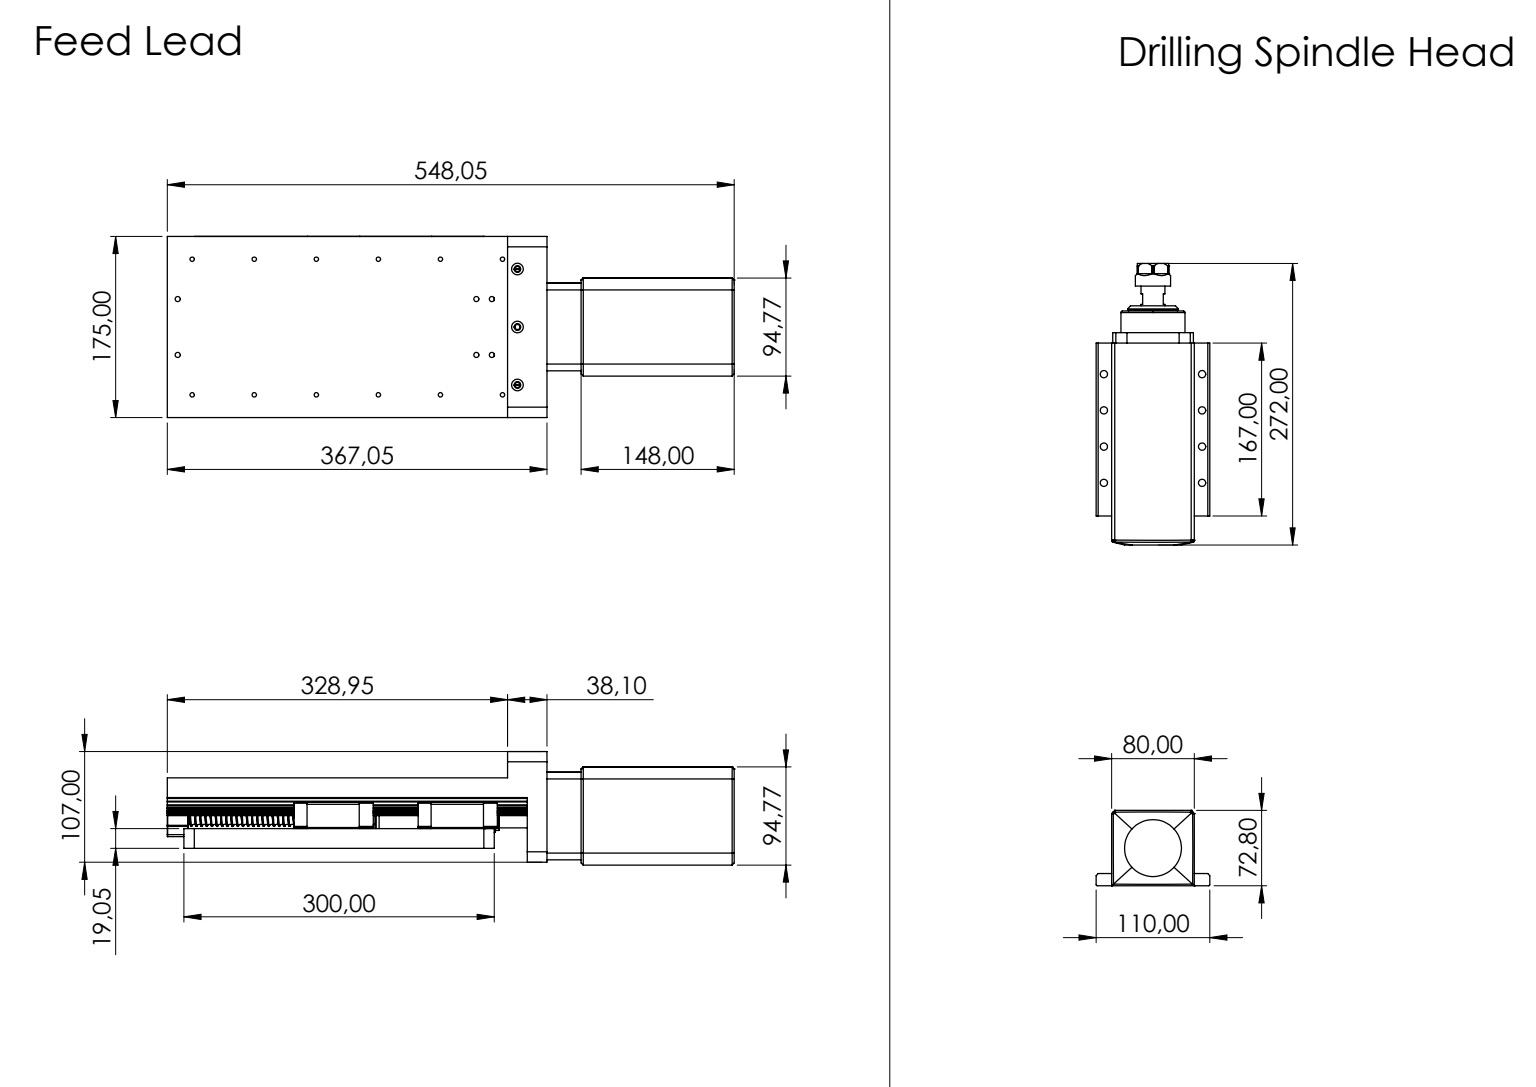
ISO-10303-21;
HEADER;
FILE_DESCRIPTION (('STEP AP214'),
    '1' );
FILE_NAME ('Drilling Spindle Head.step',
    '2026-10-07T11:37:37',
    ( '' ),
    ( '' ),
    'SwSTEP 2.0',
    'SolidWorks 2020',
    '' );
FILE_SCHEMA (( 'AUTOMOTIVE_DESIGN' ));
ENDSEC;

DATA;
#5=LINE ( 'NONE', #3140, #30301 ) ;
#8=EDGE_CURVE ( 'NONE', #34789, #75812, #45689, .T. ) ;
#18=EDGE_CURVE ( 'NONE', #81211, #49424, #24383, .T. ) ;
#40=CARTESIAN_POINT ( 'NONE',  ( 90.06670390244703128, -104.2784471599414644, 0.2178068554180012661 ) ) ;
#41=CIRCLE ( 'NONE', #63855, 11.49999999999999645 ) ;
#57=FACE_OUTER_BOUND ( 'NONE', #13007, .T. ) ;
#62=EDGE_CURVE ( 'NONE', #88900, #78359, #73421, .T. ) ;
#77=CARTESIAN_POINT ( 'NONE',  ( 128.6924155486683503, -121.3595312563307260, 250.2191008560389776 ) ) ;
#86=CARTESIAN_POINT ( 'NONE',  ( 143.0667039024470171, -90.27844715994091018, 230.7030882296565721 ) ) ;
#104=CARTESIAN_POINT ( 'NONE',  ( 107.0667039024470313, -104.2784471599420897, -20.48315503890502143 ) ) ;
#107=CARTESIAN_POINT ( 'NONE',  ( 102.3035641816324102, -89.52844715994213232, -21.78219314458246103 ) ) ;
#108=ORIENTED_EDGE ( 'NONE', *, *, #23655, .T. ) ;
#117=ORIENTED_EDGE ( 'NONE', *, *, #52215, .T. ) ;
#119=EDGE_CURVE ( 'NONE', #83222, #86794, #67726, .T. ) ;
#129=ORIENTED_EDGE ( 'NONE', *, *, #9296, .T. ) ;
#134=EDGE_CURVE ( 'NONE', #34012, #57634, #4396, .T. ) ;
#149=CARTESIAN_POINT ( 'NONE',  ( 70.08426215166053908, -140.6784470016797570, 245.7568090486316805 ) ) ;
#153=ORIENTED_EDGE ( 'NONE', *, *, #81834, .T. ) ;
#161=CARTESIAN_POINT ( 'NONE',  ( 93.91125933621934507, -111.8737466215629013, -21.78219314458179667 ) ) ;
#162=DIRECTION ( 'NONE',  ( 3.100000000000000258E-29, -3.100000000000000044E-14, -1.000000000000000000 ) ) ;
#166=ADVANCED_FACE ( 'NONE', ( #82057 ), #80705, .F. ) ;
#170=CARTESIAN_POINT ( 'NONE',  ( 147.0667039024470739, -140.6784471599409017, 222.2178068554179902 ) ) ;
#211=CARTESIAN_POINT ( 'NONE',  ( 67.65599188636636541, -68.44419502099285069, 246.9104243438740696 ) ) ;
#220=CARTESIAN_POINT ( 'NONE',  ( 107.0667039024470313, -104.2784471599414502, 0.2178068554180012661 ) ) ;
#222=ORIENTED_EDGE ( 'NONE', *, *, #9367, .T. ) ;
#256=VECTOR ( 'NONE', #25789, 1000.000000000000000 ) ;
#281=CARTESIAN_POINT ( 'NONE',  ( 147.0268936274260057, -137.6319380618105015, 245.9633055630636704 ) ) ;
#299=ORIENTED_EDGE ( 'NONE', *, *, #29707, .F. ) ;
#314=DIRECTION ( 'NONE',  ( 1.000000000000000078E-15, -1.000000000000000000, 3.100000000000000044E-14 ) ) ;
#334=DIRECTION ( 'NONE',  ( -1.000000000000000078E-15, 1.000000000000000000, 0.000000000000000000 ) ) ;
#335=ORIENTED_EDGE ( 'NONE', *, *, #11625, .F. ) ;
#377=DIRECTION ( 'NONE',  ( -3.100000000000000258E-29, 3.100000000000000044E-14, 1.000000000000000000 ) ) ;
#379=FACE_OUTER_BOUND ( 'NONE', #43441, .T. ) ;
#381=CYLINDRICAL_SURFACE ( 'NONE', #47045, 27.49999999999999645 ) ;
#390=DIRECTION ( 'NONE',  ( 0.000000000000000000, 0.000000000000000000, -1.000000000000000000 ) ) ;
#399=AXIS2_PLACEMENT_3D ( 'NONE', #39695, #12012, #46047 ) ;
#405=LINE ( 'NONE', #34471, #15075 ) ;
#407=DIRECTION ( 'NONE',  ( -1.000000000000000078E-15, 1.000000000000000000, 0.000000000000000000 ) ) ;
#413=ORIENTED_EDGE ( 'NONE', *, *, #1503, .F. ) ;
#498=CARTESIAN_POINT ( 'NONE',  ( 68.18676274767041434, -81.16192765749869409, 247.4310652601930087 ) ) ;
#503=PLANE ( 'NONE',  #15905 ) ;
#508=DIRECTION ( 'NONE',  ( -1.000000000000000000, -1.734723475976808672E-15, 0.000000000000000000 ) ) ;
#521=ORIENTED_EDGE ( 'NONE', *, *, #75430, .F. ) ;
#525=CARTESIAN_POINT ( 'NONE',  ( 114.6154092934512647, -77.76606036807542921, 250.2178068554179902 ) ) ;
#553=ORIENTED_EDGE ( 'NONE', *, *, #37978, .T. ) ;
#587=CARTESIAN_POINT ( 'NONE',  ( 96.67439905703392355, -92.77844715994214653, -21.78219314458237932 ) ) ;
#588=CARTESIAN_POINT ( 'NONE',  ( 70.69106258991376990, -139.4536831229399070, 247.3802696298695594 ) ) ;
#602=CARTESIAN_POINT ( 'NONE',  ( 68.69590989347372556, -139.3001951612658900, 245.8075977448462197 ) ) ;
#604=DIRECTION ( 'NONE',  ( -0.6757246285173468259, -5.929722281754665310E-16, 0.7371541402007408816 ) ) ;
#612=CARTESIAN_POINT ( 'NONE',  ( 103.2512128930084288, -131.5792096921222480, 250.2178068554180470 ) ) ;
#622=EDGE_CURVE ( 'NONE', #11051, #83707, #61099, .T. ) ;
#624=DIRECTION ( 'NONE',  ( -3.100000000000000258E-29, 3.100000000000000044E-14, 1.000000000000000000 ) ) ;
#625=EDGE_LOOP ( 'NONE', ( #85460, #52936 ) ) ;
#638=VERTEX_POINT ( 'NONE', #15986 ) ;
#645=FACE_OUTER_BOUND ( 'NONE', #52755, .T. ) ;
#646=CIRCLE ( 'NONE', #12254, 3.000000000000002665 ) ;
#650=CARTESIAN_POINT ( 'NONE',  ( 54.06670390244700997, -79.67844715994098692, 222.2178068554179902 ) ) ;
#651=CARTESIAN_POINT ( 'NONE',  ( 67.18382773639109473, -67.99014260483819783, 246.1660416551738990 ) ) ;
#655=ORIENTED_EDGE ( 'NONE', *, *, #13603, .F. ) ;
#661=AXIS2_PLACEMENT_3D ( 'NONE', #79117, #10504, #25470 ) ;
#663=DIRECTION ( 'NONE',  ( -0.8660254037844382635, -0.5000000000000008882, 1.550000000000000022E-14 ) ) ;
#672=DIRECTION ( 'NONE',  ( 3.100000000000000258E-29, -3.100000000000000044E-14, -1.000000000000000000 ) ) ;
#694=DIRECTION ( 'NONE',  ( -0.8660254037844392627, 0.4999999999999990008, -1.549999999999999706E-14 ) ) ;
#696=FACE_OUTER_BOUND ( 'NONE', #29082, .T. ) ;
#701=VERTEX_POINT ( 'NONE', #9167 ) ;
#714=PLANE ( 'NONE',  #87235 ) ;
#716=ORIENTED_EDGE ( 'NONE', *, *, #77579, .T. ) ;
#719=CARTESIAN_POINT ( 'NONE',  ( 107.5667039024470455, -113.7784471599413791, 2.217806855418308132 ) ) ;
#720=CARTESIAN_POINT ( 'NONE',  ( 146.8610933598213251, -137.5366814833658395, 246.4167843500817412 ) ) ;
#734=CARTESIAN_POINT ( 'NONE',  ( 107.0667039024470313, -104.2784471599418197, -11.78219314458200984 ) ) ;
#753=VERTEX_POINT ( 'NONE', #23701 ) ;
#786=ORIENTED_EDGE ( 'NONE', *, *, #30299, .T. ) ;
#793=AXIS2_PLACEMENT_3D ( 'NONE', #52763, #58282, #86014 ) ;
#811=AXIS2_PLACEMENT_3D ( 'NONE', #82943, #28399, #22065 ) ;
#817=DIRECTION ( 'NONE',  ( -3.100000000000000258E-29, 3.100000000000000044E-14, 1.000000000000000000 ) ) ;
#830=CYLINDRICAL_SURFACE ( 'NONE', #17828, 3.500000000000003109 ) ;
#835=DIRECTION ( 'NONE',  ( -1.000000000000000000, -1.734723475976808672E-15, 0.000000000000000000 ) ) ;
#887=EDGE_CURVE ( 'NONE', #701, #2874, #49105, .T. ) ;
#916=LINE ( 'NONE', #34531, #21635 ) ;
#921=FACE_BOUND ( 'NONE', #56521, .T. ) ;
#922=EDGE_CURVE ( 'NONE', #4290, #47689, #37387, .T. ) ;
#930=CIRCLE ( 'NONE', #79267, 30.99999999999998579 ) ;
#936=VECTOR ( 'NONE', #85029, 1000.000000000000000 ) ;
#942=ORIENTED_EDGE ( 'NONE', *, *, #84667, .T. ) ;
#958=DIRECTION ( 'NONE',  ( -1.000000000000000078E-15, 1.000000000000000000, 0.000000000000000000 ) ) ;
#960=VERTEX_POINT ( 'NONE', #11251 ) ;
#967=CARTESIAN_POINT ( 'NONE',  ( 99.06670390244704549, -104.2784471599421323, -21.78219314458201694 ) ) ;
#975=CARTESIAN_POINT ( 'NONE',  ( 90.06670420047028358, -137.6784471599409585, 222.2178068554179902 ) ) ;
#981=CARTESIAN_POINT ( 'NONE',  ( 103.2512128930081730, -76.97768462775967180, 250.2178068554180470 ) ) ;
#984=CARTESIAN_POINT ( 'NONE',  ( 68.76253601752615907, -136.8623718444874555, 247.4903208786739981 ) ) ;
#998=CARTESIAN_POINT ( 'NONE',  ( 158.0667039024469886, -67.87844715994090450, 120.2178068554179902 ) ) ;
#1013=DIRECTION ( 'NONE',  ( -3.100000000000000258E-29, 3.100000000000000044E-14, 1.000000000000000000 ) ) ;
#1027=DIRECTION ( 'NONE',  ( 0.000000000000000000, 0.000000000000000000, -1.000000000000000000 ) ) ;
#1060=CARTESIAN_POINT ( 'NONE',  ( 68.70366513962476063, -139.2930699478345389, 245.9105554508155649 ) ) ;
#1067=AXIS2_PLACEMENT_3D ( 'NONE', #89420, #55748, #68523 ) ;
#1076=DIRECTION ( 'NONE',  ( 0.000000000000000000, 0.000000000000000000, 1.000000000000000000 ) ) ;
#1093=DIRECTION ( 'NONE',  ( 1.000000000000000000, 1.132880637372608296E-15, 0.000000000000000000 ) ) ;
#1108=CARTESIAN_POINT ( 'NONE',  ( 107.0667039024470313, -104.2784471599413934, 2.217806855418003043 ) ) ;
#1119=AXIS2_PLACEMENT_3D ( 'NONE', #62798, #47484, #18902 ) ;
#1121=LINE ( 'NONE', #34282, #64196 ) ;
#1125=VECTOR ( 'NONE', #24217, 1000.000000000000000 ) ;
#1141=AXIS2_PLACEMENT_3D ( 'NONE', #65937, #38679, #53176 ) ;
#1172=CARTESIAN_POINT ( 'NONE',  ( 107.0667039024470313, -104.2784471599420471, -19.18411693322902423 ) ) ;
#1177=DIRECTION ( 'NONE',  ( -3.100000000000000258E-29, 3.100000000000000044E-14, 1.000000000000000000 ) ) ;
#1179=CARTESIAN_POINT ( 'NONE',  ( 151.0667039024469886, -79.67844715994088745, 190.2178068554179902 ) ) ;
#1185=ORIENTED_EDGE ( 'NONE', *, *, #8505, .T. ) ;
#1215=VECTOR ( 'NONE', #17266, 1000.000000000000000 ) ;
#1217=ORIENTED_EDGE ( 'NONE', *, *, #20900, .F. ) ;
#1226=CARTESIAN_POINT ( 'NONE',  ( 74.06670390244701707, -90.27844715994098124, 45.21780685541799727 ) ) ;
#1252=VECTOR ( 'NONE', #76868, 1000.000000000000000 ) ;
#1284=EDGE_LOOP ( 'NONE', ( #79248, #45274, #6602, #1217 ) ) ;
#1286=DIRECTION ( 'NONE',  ( 0.8660254037844345998, 0.5000000000000069944, -1.550000000000018954E-14 ) ) ;
#1289=ORIENTED_EDGE ( 'NONE', *, *, #60837, .T. ) ;
#1303=EDGE_LOOP ( 'NONE', ( #77384, #63806 ) ) ;
#1304=VERTEX_POINT ( 'NONE', #47095 ) ;
#1309=DIRECTION ( 'NONE',  ( 0.7759704746411385523, -0.6307692307692301936, 0.000000000000000000 ) ) ;
#1336=ORIENTED_EDGE ( 'NONE', *, *, #44690, .T. ) ;
#1337=VERTEX_POINT ( 'NONE', #84803 ) ;
#1348=ORIENTED_EDGE ( 'NONE', *, *, #46560, .F. ) ;
#1361=ORIENTED_EDGE ( 'NONE', *, *, #7930, .F. ) ;
#1369=ORIENTED_EDGE ( 'NONE', *, *, #61406, .F. ) ;
#1409=CARTESIAN_POINT ( 'NONE',  ( 67.06670390244705970, -127.7048595798752899, 245.5588919304049682 ) ) ;
#1424=CARTESIAN_POINT ( 'NONE',  ( 144.0667052733537901, -83.77844715994089597, 55.21780685541800437 ) ) ;
#1431=CYLINDRICAL_SURFACE ( 'NONE', #27367, 3.000000000000002665 ) ;
#1435=VECTOR ( 'NONE', #88705, 1000.000000000000227 ) ;
#1500=CARTESIAN_POINT ( 'NONE',  ( 99.48898161933324502, -91.15344715994181968, -11.78219314458242550 ) ) ;
#1503=EDGE_CURVE ( 'NONE', #25396, #23110, #20428, .T. ) ;
#1504=ORIENTED_EDGE ( 'NONE', *, *, #70487, .F. ) ;
#1506=DIRECTION ( 'NONE',  ( -3.100000000000000258E-29, 3.100000000000000044E-14, 1.000000000000000000 ) ) ;
#1507=CARTESIAN_POINT ( 'NONE',  ( 70.74156425739846554, -139.3372952672478675, 247.4251605867160890 ) ) ;
#1539=VERTEX_POINT ( 'NONE', #34271 ) ;
#1546=AXIS2_PLACEMENT_3D ( 'NONE', #84659, #29240, #27879 ) ;
#1567=CARTESIAN_POINT ( 'NONE',  ( 67.64413875234457407, -68.43291640910719309, 246.8985623378813159 ) ) ;
#1569=ORIENTED_EDGE ( 'NONE', *, *, #59201, .F. ) ;
#1573=ADVANCED_FACE ( 'NONE', ( #75171, #55136 ), #5237, .T. ) ;
#1585=ORIENTED_EDGE ( 'NONE', *, *, #13032, .F. ) ;
#1602=ORIENTED_EDGE ( 'NONE', *, *, #5397, .T. ) ;
#1605=EDGE_CURVE ( 'NONE', #72685, #51113, #82002, .T. ) ;
#1616=AXIS2_PLACEMENT_3D ( 'NONE', #45612, #38825, #79744 ) ;
#1627=VERTEX_POINT ( 'NONE', #6140 ) ;
#1673=DIRECTION ( 'NONE',  ( -1.000000000000000000, -1.541976423090496028E-15, 0.000000000000000000 ) ) ;
#1678=DIRECTION ( 'NONE',  ( 0.5000000000000015543, 0.8660254037844377084, -2.688821387764056676E-14 ) ) ;
#1679=PLANE ( 'NONE',  #16706 ) ;
#1684=VECTOR ( 'NONE', #64083, 1000.000000000000000 ) ;
#1698=CARTESIAN_POINT ( 'NONE',  ( 107.9678037105606450, -121.2545485715094316, -21.78219314458149114 ) ) ;
#1708=ORIENTED_EDGE ( 'NONE', *, *, #73968, .F. ) ;
#1714=EDGE_CURVE ( 'NONE', #61133, #37103, #77865, .T. ) ;
#1722=CARTESIAN_POINT ( 'NONE',  ( 66.95718368952854860, -124.7784471599409954, 55.21780685541800437 ) ) ;
#1723=ORIENTED_EDGE ( 'NONE', *, *, #20357, .T. ) ;
#1738=DIRECTION ( 'NONE',  ( 1.000000000000000078E-15, -1.000000000000000000, 0.000000000000000000 ) ) ;
#1741=CARTESIAN_POINT ( 'NONE',  ( 110.0667047667142953, -67.87844715994094713, 115.9678068554179902 ) ) ;
#1742=VERTEX_POINT ( 'NONE', #13838 ) ;
#1745=VERTEX_POINT ( 'NONE', #41521 ) ;
#1758=LINE ( 'NONE', #63982, #48154 ) ;
#1769=CIRCLE ( 'NONE', #75679, 2.999999999999988898 ) ;
#1783=CARTESIAN_POINT ( 'NONE',  ( 74.19170390244700286, -80.65344715994098124, 45.21780685541799727 ) ) ;
#1809=CARTESIAN_POINT ( 'NONE',  ( 68.91673588226457525, -69.56165432392101877, 247.5002287295815790 ) ) ;
#1820=B_SPLINE_CURVE_WITH_KNOTS ( 'NONE', 3,
 ( #34572, #20518, #75917, #13685, #69105 ),
 .UNSPECIFIED., .F., .F.,
 ( 4, 1, 4 ),
 ( 0.000000000000000000, 0.4316414630428307975, 1.000000000000000000 ),
 .UNSPECIFIED. ) ;
#1835=AXIS2_PLACEMENT_3D ( 'NONE', #87398, #74220, #60113 ) ;
#1851=EDGE_CURVE ( 'NONE', #85229, #66416, #26062, .T. ) ;
#1857=CARTESIAN_POINT ( 'NONE',  ( 67.36714851195648635, -67.87168324244640871, 246.8533852577239998 ) ) ;
#1864=VERTEX_POINT ( 'NONE', #16088 ) ;
#1907=EDGE_CURVE ( 'NONE', #41462, #11071, #64672, .T. ) ;
#1923=FACE_OUTER_BOUND ( 'NONE', #29612, .T. ) ;
#1929=LINE ( 'NONE', #56417, #15979 ) ;
#1934=VECTOR ( 'NONE', #63013, 1000.000000000000000 ) ;
#1951=CARTESIAN_POINT ( 'NONE',  ( 70.50919912965197511, -139.8621867207610308, 247.1491889055018305 ) ) ;
#1990=DIRECTION ( 'NONE',  ( -1.000000000000000000, -1.000000000000000078E-15, 5.773159642023980606E-15 ) ) ;
#1991=FACE_OUTER_BOUND ( 'NONE', #56263, .T. ) ;
#1992=CARTESIAN_POINT ( 'NONE',  ( 146.5099599153435008, -138.2352025272441836, 245.9283337036430055 ) ) ;
#2001=DIRECTION ( 'NONE',  ( -1.000000000000000000, 0.000000000000000000, 0.000000000000000000 ) ) ;
#2010=ORIENTED_EDGE ( 'NONE', *, *, #76441, .F. ) ;
#2011=ORIENTED_EDGE ( 'NONE', *, *, #41800, .F. ) ;
#2013=EDGE_CURVE ( 'NONE', #61542, #42555, #33274, .T. ) ;
#2016=CARTESIAN_POINT ( 'NONE',  ( 145.3595637443018234, -69.45303146431501773, 247.4784022495120155 ) ) ;
#2030=DIRECTION ( 'NONE',  ( 1.000000000000000000, 1.000000000000000078E-15, 0.000000000000000000 ) ) ;
#2032=ORIENTED_EDGE ( 'NONE', *, *, #52612, .F. ) ;
#2057=CARTESIAN_POINT ( 'NONE',  ( 68.09411347895392908, -99.27098689615887395, 247.4783998280180128 ) ) ;
#2058=ORIENTED_EDGE ( 'NONE', *, *, #78733, .F. ) ;
#2060=ORIENTED_EDGE ( 'NONE', *, *, #17855, .F. ) ;
#2106=EDGE_CURVE ( 'NONE', #64360, #47447, #53685, .T. ) ;
#2107=VERTEX_POINT ( 'NONE', #61415 ) ;
#2119=LINE ( 'NONE', #17528, #69835 ) ;
#2121=AXIS2_PLACEMENT_3D ( 'NONE', #62039, #89773, #41583 ) ;
#2122=LINE ( 'NONE', #71173, #32626 ) ;
#2160=ORIENTED_EDGE ( 'NONE', *, *, #19869, .F. ) ;
#2164=CARTESIAN_POINT ( 'NONE',  ( 151.0667039024469886, -67.87844715994090450, 190.2178068554179902 ) ) ;
#2168=LINE ( 'NONE', #56199, #62006 ) ;
#2185=CIRCLE ( 'NONE', #13772, 3.999999999999992895 ) ;
#2203=ORIENTED_EDGE ( 'NONE', *, *, #46360, .F. ) ;
#2205=LINE ( 'NONE', #8118, #27880 ) ;
#2209=CARTESIAN_POINT ( 'NONE',  ( 110.2536356736639078, -101.8611209747513868, -19.78219314458209865 ) ) ;
#2215=VECTOR ( 'NONE', #80038, 1000.000000000000000 ) ;
#2218=VECTOR ( 'NONE', #39800, 1000.000000000000000 ) ;
#2222=DIRECTION ( 'NONE',  ( 0.000000000000000000, 0.000000000000000000, 1.000000000000000000 ) ) ;
#2224=EDGE_CURVE ( 'NONE', #51923, #24886, #89215, .T. ) ;
#2254=DIRECTION ( 'NONE',  ( -1.000000000000000000, -1.000000000000000078E-15, 0.000000000000000000 ) ) ;
#2263=CIRCLE ( 'NONE', #22569, 7.999999999999992895 ) ;
#2264=ORIENTED_EDGE ( 'NONE', *, *, #48437, .T. ) ;
#2267=DIRECTION ( 'NONE',  ( 3.100000000000000258E-29, -3.100000000000000044E-14, -1.000000000000000000 ) ) ;
#2270=CARTESIAN_POINT ( 'NONE',  ( 143.6785940946288633, -138.5762527540428835, 247.5817532094160072 ) ) ;
#2273=DIRECTION ( 'NONE',  ( -1.000000000000000078E-15, 1.000000000000000000, 0.000000000000000000 ) ) ;
#2274=ORIENTED_EDGE ( 'NONE', *, *, #31325, .T. ) ;
#2298=B_SPLINE_CURVE_WITH_KNOTS ( 'NONE', 3,
 ( #3064, #28982, #86185, #14912 ),
 .UNSPECIFIED., .F., .F.,
 ( 4, 4 ),
 ( -0.3974825557268150122, -0.3842043193313849914 ),
 .UNSPECIFIED. ) ;
#2302=ORIENTED_EDGE ( 'NONE', *, *, #57521, .T. ) ;
#2303=DIRECTION ( 'NONE',  ( -0.4999999999999989453, -0.8660254037844392627, 2.684678751731760294E-14 ) ) ;
#2324=AXIS2_PLACEMENT_3D ( 'NONE', #19974, #41733, #69919 ) ;
#2337=CARTESIAN_POINT ( 'NONE',  ( 147.0667039024469886, -67.87844715994090450, 222.2178068554179902 ) ) ;
#2348=CARTESIAN_POINT ( 'NONE',  ( 115.0988951105837117, -100.2184096729307328, 2.217806855417864043 ) ) ;
#2390=B_SPLINE_CURVE_WITH_KNOTS ( 'NONE', 3,
 ( #7423, #48730, #29221, #63284, #69654, #35115, #62824, #602, #15597, #21515, #1060, #56908, #49185, #76919, #50085, #77819, #28770, #38692, #65952, #44608, #2409, #23754, #23321, #16931, #36922, #64624, #51861, #72344, #10111, #66397, #17814, #71461, #50987, #43722, #17371, #51422, #9224, #38255, #78728, #16485, #79171, #4187, #37820, #65074, #58684 ),
 .UNSPECIFIED., .F., .F.,
 ( 4, 2, 2, 2, 1, 1, 2, 2, 2, 1, 1, 2, 2, 2, 2, 1, 1, 1, 2, 2, 2, 2, 1, 1, 2, 2, 4 ),
 ( 0.000000000000000000, 0.03125000000003638062, 0.04687500000005471318, 0.06250000000007303880, 0.09375000000011092516, 0.1093750000001298545, 0.1171875000001566386, 0.1250000000001834088, 0.1875000000003400336, 0.2187500000004195255, 0.2343750000004746481, 0.2421875000004988232, 0.2500000000005230261, 0.3750000000008891776, 0.4375000000010721979, 0.4687500000011416423, 0.4843750000011794454, 0.4921875000012016499, 0.4960937500012127521, 0.5000000000012239099, 0.6250000000010771384, 0.6875000000010104140, 0.7187500000009768852, 0.7343750000009601209, 0.7421875000009404699, 0.7500000000009208190, 1.000000000000000000 ),
 .UNSPECIFIED. ) ;
#2394=DIRECTION ( 'NONE',  ( 0.000000000000000000, 0.000000000000000000, 1.000000000000000000 ) ) ;
#2399=DIRECTION ( 'NONE',  ( 0.8660254037844382635, 0.5000000000000008882, -1.550000000000000022E-14 ) ) ;
#2402=ORIENTED_EDGE ( 'NONE', *, *, #19038, .F. ) ;
#2409=CARTESIAN_POINT ( 'NONE',  ( 68.75201276470878042, -139.2464705024164857, 246.2314480513125261 ) ) ;
#2466=CARTESIAN_POINT ( 'NONE',  ( 145.2750608293226833, -69.56425712815943996, 247.5000682988239760 ) ) ;
#2467=CARTESIAN_POINT ( 'NONE',  ( 146.2016781114348305, -68.71199849507584645, 247.1480963241265272 ) ) ;
#2481=ORIENTED_EDGE ( 'NONE', *, *, #35705, .F. ) ;
#2532=ORIENTED_EDGE ( 'NONE', *, *, #31514, .F. ) ;
#2534=DIRECTION ( 'NONE',  ( -3.100000000000000258E-29, 3.100000000000000044E-14, 1.000000000000000000 ) ) ;
#2559=VECTOR ( 'NONE', #87502, 1000.000000000000000 ) ;
#2572=CARTESIAN_POINT ( 'NONE',  ( 67.06681736700808472, -67.87844715931913697, 245.5130139978070076 ) ) ;
#2577=VECTOR ( 'NONE', #78490, 1000.000000000000000 ) ;
#2587=ORIENTED_EDGE ( 'NONE', *, *, #83860, .T. ) ;
#2593=LINE ( 'NONE', #1698, #76570 ) ;
#2630=LINE ( 'NONE', #24848, #17598 ) ;
#2634=AXIS2_PLACEMENT_3D ( 'NONE', #66343, #30502, #71407 ) ;
#2636=DIRECTION ( 'NONE',  ( 0.000000000000000000, 0.000000000000000000, -1.000000000000000000 ) ) ;
#2648=VECTOR ( 'NONE', #89767, 1000.000000000000000 ) ;
#2668=AXIS2_PLACEMENT_3D ( 'NONE', #71158, #37954, #77965 ) ;
#2669=ORIENTED_EDGE ( 'NONE', *, *, #58690, .F. ) ;
#2677=CARTESIAN_POINT ( 'NONE',  ( 107.0667039024470313, -104.2784471599418197, -11.78219314458200984 ) ) ;
#2691=ORIENTED_EDGE ( 'NONE', *, *, #72281, .T. ) ;
#2702=CARTESIAN_POINT ( 'NONE',  ( 68.90393785523644965, -69.55022374562288690, 247.4982723397321251 ) ) ;
#2707=DIRECTION ( 'NONE',  ( -0.000000000000000000, -0.000000000000000000, -1.000000000000000000 ) ) ;
#2737=CARTESIAN_POINT ( 'NONE',  ( 56.06670390244699576, -67.87844715994098976, 190.2178068554179902 ) ) ;
#2745=DIRECTION ( 'NONE',  ( 1.000000000000000078E-15, -1.000000000000000000, 0.000000000000000000 ) ) ;
#2749=CARTESIAN_POINT ( 'NONE',  ( 107.0667039024469886, -67.87844715994094713, 93.21780685541800437 ) ) ;
#2772=CARTESIAN_POINT ( 'NONE',  ( 67.06670390244707392, -137.6766936484476958, 245.4930518797220032 ) ) ;
#2777=VECTOR ( 'NONE', #34885, 999.9999999999998863 ) ;
#2833=VERTEX_POINT ( 'NONE', #28364 ) ;
#2834=CYLINDRICAL_SURFACE ( 'NONE', #80225, 3.499999999999996003 ) ;
#2858=CARTESIAN_POINT ( 'NONE',  ( 67.06670390244700286, -67.87844715994098976, 222.2178068554179902 ) ) ;
#2874=VERTEX_POINT ( 'NONE', #58738 ) ;
#2875=CARTESIAN_POINT ( 'NONE',  ( 107.0667039024470313, -104.2784471599420897, -20.48315503890502143 ) ) ;
#2885=CARTESIAN_POINT ( 'NONE',  ( 77.06670390244701707, -90.27844715994098124, 230.7030882296565721 ) ) ;
#2909=CARTESIAN_POINT ( 'NONE',  ( 90.57859886853759690, -68.78570139166994579, 247.5000682988239760 ) ) ;
#2910=CARTESIAN_POINT ( 'NONE',  ( 146.9135422721272448, -68.02287184880887594, 246.2552768418564710 ) ) ;
#2921=ORIENTED_EDGE ( 'NONE', *, *, #10620, .F. ) ;
#2927=VECTOR ( 'NONE', #1076, 1000.000000000000000 ) ;
#2929=ORIENTED_EDGE ( 'NONE', *, *, #70817, .T. ) ;
#2951=VECTOR ( 'NONE', #72879, 1000.000000000000000 ) ;
#3003=CARTESIAN_POINT ( 'NONE',  ( 129.9417039024469886, -68.87844715994091871, 138.7178068554180186 ) ) ;
#3021=ORIENTED_EDGE ( 'NONE', *, *, #29193, .T. ) ;
#3022=ORIENTED_EDGE ( 'NONE', *, *, #18736, .F. ) ;
#3023=EDGE_CURVE ( 'NONE', #28371, #5243, #34541, .T. ) ;
#3032=AXIS2_PLACEMENT_3D ( 'NONE', #32379, #68272, #87814 ) ;
#3053=VERTEX_POINT ( 'NONE', #87807 ) ;
#3059=ORIENTED_EDGE ( 'NONE', *, *, #48221, .T. ) ;
#3060=VECTOR ( 'NONE', #65842, 999.9999999999998863 ) ;
#3064=CARTESIAN_POINT ( 'NONE',  ( 107.9678037105606023, -87.30234574837474781, -19.18411693322955003 ) ) ;
#3075=CARTESIAN_POINT ( 'NONE',  ( 143.0667039024470171, -118.2784471599408960, 230.7030882296565721 ) ) ;
#3077=CARTESIAN_POINT ( 'NONE',  ( 82.96822048844396136, -129.2743616038035555, 249.3173333679100097 ) ) ;
#3082=ORIENTED_EDGE ( 'NONE', *, *, #36963, .F. ) ;
#3089=FACE_OUTER_BOUND ( 'NONE', #23564, .T. ) ;
#3126=CIRCLE ( 'NONE', #14750, 1.500000000000001332 ) ;
#3136=CIRCLE ( 'NONE', #7483, 4.500000000000003553 ) ;
#3140=CARTESIAN_POINT ( 'NONE',  ( 67.06670390244707392, -137.6784471599409869, 228.4678068554179902 ) ) ;
#3142=CARTESIAN_POINT ( 'NONE',  ( 92.91125933621934507, -113.6057974291316981, -19.26696060647573105 ) ) ;
#3143=CYLINDRICAL_SURFACE ( 'NONE', #12103, 24.50000000000000711 ) ;
#3171=AXIS2_PLACEMENT_3D ( 'NONE', #33661, #51948, #31080 ) ;
#3193=ORIENTED_EDGE ( 'NONE', *, *, #4873, .T. ) ;
#3194=CARTESIAN_POINT ( 'NONE',  ( 110.2536356736639220, -106.6957733451320394, 2.217806855418086087 ) ) ;
#3197=CIRCLE ( 'NONE', #10449, 3.500000000000003109 ) ;
#3263=ORIENTED_EDGE ( 'NONE', *, *, #64249, .T. ) ;
#3266=DIRECTION ( 'NONE',  ( 1.000000000000000078E-15, -1.000000000000000000, 3.100000000000000044E-14 ) ) ;
#3289=ORIENTED_EDGE ( 'NONE', *, *, #36504, .T. ) ;
#3332=FACE_OUTER_BOUND ( 'NONE', #52166, .T. ) ;
#3347=AXIS2_PLACEMENT_3D ( 'NONE', #55568, #56024, #63315 ) ;
#3356=CARTESIAN_POINT ( 'NONE',  ( 86.71899144006731319, -85.80981821983746727, 250.2201230397200220 ) ) ;
#3358=DIRECTION ( 'NONE',  ( -1.000000000000000000, 0.000000000000000000, 0.000000000000000000 ) ) ;
#3367=ADVANCED_FACE ( 'NONE', ( #24580 ), #52247, .F. ) ;
#3370=DIRECTION ( 'NONE',  ( 3.100000000000000258E-29, -3.100000000000000044E-14, -1.000000000000000000 ) ) ;
#3381=VERTEX_POINT ( 'NONE', #80009 ) ;
#3391=ORIENTED_EDGE ( 'NONE', *, *, #2013, .T. ) ;
#3399=CARTESIAN_POINT ( 'NONE',  ( 123.1292039024470029, -68.87844715994093292, 222.2178068554179902 ) ) ;
#3408=ADVANCED_BREP_SHAPE_REPRESENTATION ( '', ( #20639, #50656 ), #4304 ) ;
#3411=CARTESIAN_POINT ( 'NONE',  ( 67.49635100332064042, -137.4243301806155841, 246.7471779864713994 ) ) ;
#3412=DIRECTION ( 'NONE',  ( -3.100000000000000258E-29, 3.100000000000000044E-14, 1.000000000000000000 ) ) ;
#3439=ORIENTED_EDGE ( 'NONE', *, *, #23571, .T. ) ;
#3443=CARTESIAN_POINT ( 'NONE',  ( 147.0667039024470739, -137.6784471599409017, 228.4678068554179902 ) ) ;
#3464=EDGE_LOOP ( 'NONE', ( #42569, #33408, #27715, #60217, #68798, #53637, #1185, #81075, #30294, #70743, #67951, #15665, #4398, #59481, #21360, #55428, #73289, #84793, #23699, #19501, #86373, #70073 ) ) ;
#3465=EDGE_LOOP ( 'NONE', ( #22122, #15213, #52644, #21783 ) ) ;
#3476=DIRECTION ( 'NONE',  ( -1.000000000000000078E-15, 1.000000000000000000, 0.000000000000000000 ) ) ;
#3479=ORIENTED_EDGE ( 'NONE', *, *, #7458, .T. ) ;
#3524=VECTOR ( 'NONE', #83759, 1000.000000000000000 ) ;
#3528=ORIENTED_EDGE ( 'NONE', *, *, #29932, .T. ) ;
#3539=DIRECTION ( 'NONE',  ( -1.000000000000000000, -1.541976423090496028E-15, 0.000000000000000000 ) ) ;
#3543=ORIENTED_EDGE ( 'NONE', *, *, #20270, .F. ) ;
#3551=EDGE_CURVE ( 'NONE', #88193, #23818, #74962, .T. ) ;
#3578=CARTESIAN_POINT ( 'NONE',  ( 112.7812478461076040, -67.87844715994094713, 245.8358747327640117 ) ) ;
#3596=LINE ( 'NONE', #65219, #86816 ) ;
#3628=DIRECTION ( 'NONE',  ( 1.000000000000000078E-15, -1.000000000000000000, 0.000000000000000000 ) ) ;
#3634=FACE_BOUND ( 'NONE', #68129, .T. ) ;
#3641=DIRECTION ( 'NONE',  ( -1.000000000000000078E-15, 1.000000000000000000, 0.000000000000000000 ) ) ;
#3710=VECTOR ( 'NONE', #80088, 1000.000000000000000 ) ;
#3730=AXIS2_PLACEMENT_3D ( 'NONE', #30373, #9044, #2222 ) ;
#3747=PLANE ( 'NONE',  #31791 ) ;
#3757=VECTOR ( 'NONE', #82035, 1000.000000000000000 ) ;
#3786=CARTESIAN_POINT ( 'NONE',  ( 98.58946256649487339, -99.96145986183429955, -19.78219314458215550 ) ) ;
#3792=ORIENTED_EDGE ( 'NONE', *, *, #60951, .F. ) ;
#3794=CARTESIAN_POINT ( 'NONE',  ( 130.8259623650636172, -69.00418878328892447, 247.5000682988239760 ) ) ;
#3800=DIRECTION ( 'NONE',  ( 3.100000000000000258E-29, -3.100000000000000044E-14, -1.000000000000000000 ) ) ;
#3829=CARTESIAN_POINT ( 'NONE',  ( 107.0667039024470313, -104.2784471599408676, 19.21780685541799016 ) ) ;
#3832=ORIENTED_EDGE ( 'NONE', *, *, #72216, .F. ) ;
#3834=AXIS2_PLACEMENT_3D ( 'NONE', #63675, #55033, #13732 ) ;
#3842=AXIS2_PLACEMENT_3D ( 'NONE', #36859, #57745, #72282 ) ;
#3843=CARTESIAN_POINT ( 'NONE',  ( 107.0667039024470313, -104.2784471599414502, 0.2178068554180012661 ) ) ;
#3844=CARTESIAN_POINT ( 'NONE',  ( 143.2522959336310748, -139.0102598546870922, 247.5112310255240118 ) ) ;
#3850=EDGE_CURVE ( 'NONE', #44698, #89450, #63272, .T. ) ;
#3854=CARTESIAN_POINT ( 'NONE',  ( 67.10629922391730418, -137.6313948336576232, 245.9678581484365907 ) ) ;
#3858=ORIENTED_EDGE ( 'NONE', *, *, #2106, .T. ) ;
#3879=DIRECTION ( 'NONE',  ( 3.100000000000000258E-29, -3.100000000000000044E-14, -1.000000000000000000 ) ) ;
#3901=CARTESIAN_POINT ( 'NONE',  ( 82.02983075842482208, -92.77767617834393832, 250.2178068554179902 ) ) ;
#3905=CIRCLE ( 'NONE', #50324, 173.3227045127110273 ) ;
#3909=ORIENTED_EDGE ( 'NONE', *, *, #10072, .T. ) ;
#3917=AXIS2_PLACEMENT_3D ( 'NONE', #27024, #56950, #14751 ) ;
#3918=AXIS2_PLACEMENT_3D ( 'NONE', #54513, #5968, #40012 ) ;
#3930=CARTESIAN_POINT ( 'NONE',  ( 110.2536356736639078, -101.8611209747513868, -19.78219314458209865 ) ) ;
#3952=CARTESIAN_POINT ( 'NONE',  ( 97.06670390244703128, -109.9573555057411340, 17.71780685541815714 ) ) ;
#3955=ORIENTED_EDGE ( 'NONE', *, *, #34121, .F. ) ;
#3956=FACE_OUTER_BOUND ( 'NONE', #75464, .T. ) ;
#3960=CARTESIAN_POINT ( 'NONE',  ( 103.8797721312301547, -106.6957733451327215, -19.78219314458193168 ) ) ;
#3965=CARTESIAN_POINT ( 'NONE',  ( 107.0667039024470313, -104.2784471599413934, 2.217806855418003043 ) ) ;
#3973=VERTEX_POINT ( 'NONE', #44001 ) ;
#3975=VECTOR ( 'NONE', #27151, 1000.000000000000000 ) ;
#3980=ORIENTED_EDGE ( 'NONE', *, *, #65488, .F. ) ;
#3981=DIRECTION ( 'NONE',  ( 0.000000000000000000, 0.000000000000000000, -1.000000000000000000 ) ) ;
#3983=FACE_OUTER_BOUND ( 'NONE', #80737, .T. ) ;
#3984=EDGE_CURVE ( 'NONE', #79449, #88193, #70403, .T. ) ;
#3986=CARTESIAN_POINT ( 'NONE',  ( 122.2189888861420286, -111.9861225405540353, -19.18411693322877198 ) ) ;
#4008=ADVANCED_FACE ( 'NONE', ( #24920 ), #47573, .T. ) ;
#4023=FACE_OUTER_BOUND ( 'NONE', #50223, .T. ) ;
#4049=ORIENTED_EDGE ( 'NONE', *, *, #30302, .T. ) ;
#4051=CARTESIAN_POINT ( 'NONE',  ( 125.5177273812784762, -131.0330679306342461, 55.21780685541800437 ) ) ;
#4069=ORIENTED_EDGE ( 'NONE', *, *, #17170, .T. ) ;
#4081=CARTESIAN_POINT ( 'NONE',  ( 91.91229715706504066, -111.9484203394872850, -19.21044887263775891 ) ) ;
#4089=PLANE ( 'NONE',  #64691 ) ;
#4092=CARTESIAN_POINT ( 'NONE',  ( 67.06673837846007302, -137.6758525980020806, 245.5072637273240161 ) ) ;
#4094=CIRCLE ( 'NONE', #86776, 7.999999999999992895 ) ;
#4100=VERTEX_POINT ( 'NONE', #67139 ) ;
#4108=DIRECTION ( 'NONE',  ( 1.000000000000000000, 1.000000000000013883E-15, 4.440892098500630106E-16 ) ) ;
#4111=VERTEX_POINT ( 'NONE', #81691 ) ;
#4122=DIRECTION ( 'NONE',  ( 0.4999999999999994449, 0.8660254037844390407, -2.684678751731759347E-14 ) ) ;
#4130=CARTESIAN_POINT ( 'NONE',  ( 122.2221484686745185, -96.57698625956679450, -11.78219314458225853 ) ) ;
#4132=VECTOR ( 'NONE', #47429, 1000.000000000000000 ) ;
#4137=ADVANCED_FACE ( 'NONE', ( #38983 ), #88939, .F. ) ;
#4139=ORIENTED_EDGE ( 'NONE', *, *, #52958, .T. ) ;
#4179=CIRCLE ( 'NONE', #31725, 3.499999999999996003 ) ;
#4187=CARTESIAN_POINT ( 'NONE',  ( 69.39098523492604897, -138.6132424365590623, 247.3878207843068537 ) ) ;
#4207=ORIENTED_EDGE ( 'NONE', *, *, #20358, .F. ) ;
#4211=CARTESIAN_POINT ( 'NONE',  ( 52.06670390244699576, -68.87844715994100397, 180.4678068554179902 ) ) ;
#4218=DIRECTION ( 'NONE',  ( -1.000000000000000000, -8.163404592832032979E-16, 0.000000000000000000 ) ) ;
#4222=ORIENTED_EDGE ( 'NONE', *, *, #83968, .T. ) ;
#4227=CARTESIAN_POINT ( 'NONE',  ( 107.5667039024470455, -113.7784471599420613, -19.78219314458171141 ) ) ;
#4238=ORIENTED_EDGE ( 'NONE', *, *, #48664, .F. ) ;
#4254=EDGE_CURVE ( 'NONE', #84281, #82155, #2593, .T. ) ;
#4271=DIRECTION ( 'NONE',  ( -1.000000000000000078E-15, 1.000000000000000000, 0.000000000000000000 ) ) ;
#4284=VERTEX_POINT ( 'NONE', #78901 ) ;
#4290=VERTEX_POINT ( 'NONE', #85277 ) ;
#4295=CARTESIAN_POINT ( 'NONE',  ( 143.3672529448882642, -139.2813379893231343, 247.4476445910851510 ) ) ;
#4304=( GEOMETRIC_REPRESENTATION_CONTEXT ( 3 ) GLOBAL_UNCERTAINTY_ASSIGNED_CONTEXT ( ( #33563 ) ) GLOBAL_UNIT_ASSIGNED_CONTEXT ( ( #70451, #75914, #70908 ) ) REPRESENTATION_CONTEXT ( 'NONE', 'WORKASPACE' ) );
#4317=DIRECTION ( 'NONE',  ( -1.000000000000000000, -1.000000000000000078E-15, 0.000000000000000000 ) ) ;
#4327=CARTESIAN_POINT ( 'NONE',  ( 107.5667039024470455, -113.7784471599413791, 2.217806855418308132 ) ) ;
#4333=CARTESIAN_POINT ( 'NONE',  ( 104.0667030381801936, -67.87844715994094713, 173.2178086137559774 ) ) ;
#4351=VERTEX_POINT ( 'NONE', #78005 ) ;
#4354=CARTESIAN_POINT ( 'NONE',  ( 139.9417039024470171, -80.65344715994091018, 45.21780685541799727 ) ) ;
#4358=VECTOR ( 'NONE', #85533, 1000.000000000000000 ) ;
#4359=ADVANCED_FACE ( 'NONE', ( #23495 ), #57986, .F. ) ;
#4365=CARTESIAN_POINT ( 'NONE',  ( 107.0667039024470313, -104.2784471599409528, 222.2178068554179902 ) ) ;
#4372=EDGE_CURVE ( 'NONE', #14487, #29010, #58426, .T. ) ;
#4373=CARTESIAN_POINT ( 'NONE',  ( 122.2221484686747317, -101.0284471599423171, -21.78219314458213063 ) ) ;
#4381=VERTEX_POINT ( 'NONE', #8512 ) ;
#4396=LINE ( 'NONE', #89310, #30010 ) ;
#4398=ORIENTED_EDGE ( 'NONE', *, *, #64525, .T. ) ;
#4400=ORIENTED_EDGE ( 'NONE', *, *, #36676, .F. ) ;
#4420=EDGE_LOOP ( 'NONE', ( #18490, #13736, #2274, #22151 ) ) ;
#4437=CARTESIAN_POINT ( 'NONE',  ( 144.0769060499356726, -139.5326789363695070, 247.4193337233699879 ) ) ;
#4439=CARTESIAN_POINT ( 'NONE',  ( 70.06670390834486284, -140.6784471658387758, 245.4415720115519832 ) ) ;
#4443=ORIENTED_EDGE ( 'NONE', *, *, #9309, .T. ) ;
#4445=DIRECTION ( 'NONE',  ( 0.000000000000000000, 0.000000000000000000, -1.000000000000000000 ) ) ;
#4447=DIRECTION ( 'NONE',  ( -0.000000000000000000, -0.000000000000000000, -1.000000000000000000 ) ) ;
#4450=VECTOR ( 'NONE', #68836, 1000.000000000000000 ) ;
#4455=CARTESIAN_POINT ( 'NONE',  ( 107.0667039024470313, -104.2784471599408676, 19.21780685541799016 ) ) ;
#4463=EDGE_CURVE ( 'NONE', #1539, #26346, #26878, .T. ) ;
#4478=DIRECTION ( 'NONE',  ( 1.000000000000000000, 1.000000000000000078E-15, 0.000000000000000000 ) ) ;
#4479=CARTESIAN_POINT ( 'NONE',  ( 125.5177273812784762, -137.6784471599409301, 222.2178068554179902 ) ) ;
#4498=DIRECTION ( 'NONE',  ( -3.100000000000000258E-29, 3.100000000000000044E-14, 1.000000000000000000 ) ) ;
#4509=AXIS2_PLACEMENT_3D ( 'NONE', #33754, #28266, #13318 ) ;
#4517=VERTEX_POINT ( 'NONE', #32501 ) ;
#4520=CARTESIAN_POINT ( 'NONE',  ( 122.2189888861420286, -111.9861225405540353, -19.18411693322877198 ) ) ;
#4523=LINE ( 'NONE', #45386, #1215 ) ;
#4538=ORIENTED_EDGE ( 'NONE', *, *, #17583, .T. ) ;
#4540=B_SPLINE_SURFACE_WITH_KNOTS ( 'NONE', 3, 3, ( 
 ( #64494, #2270, #29525, #9526 ),
 ( #84952, #37228, #16342, #70415 ),
 ( #57208, #9975, #77229, #16787 ),
 ( #37680, #64933, #43578, #29972 ),
 ( #42675, #58546, #30858, #58114 ) ),
 .UNSPECIFIED., .F., .F., .F.,
 ( 4, 1, 4 ),
 ( 4, 4 ),
 ( 0.000000000000000000, 0.5714285714285709528, 1.000000000000000000 ),
 ( 4.195560071017320097E-05, 0.2154603786882610117 ),
 .UNSPECIFIED. ) ;
#4553=VECTOR ( 'NONE', #7313, 1000.000000000000000 ) ;
#4558=DIRECTION ( 'NONE',  ( -3.100000000000000258E-29, 3.100000000000000044E-14, 1.000000000000000000 ) ) ;
#4575=FACE_OUTER_BOUND ( 'NONE', #80124, .T. ) ;
#4627=CARTESIAN_POINT ( 'NONE',  ( 83.34564128298197261, -139.5081389887196792, 247.5112265945679724 ) ) ;
#4675=DIRECTION ( 'NONE',  ( -0.8660254037844382635, -0.5000000000000008882, 1.550000000000000022E-14 ) ) ;
#4684=DIRECTION ( 'NONE',  ( 0.000000000000000000, 0.000000000000000000, -1.000000000000000000 ) ) ;
#4696=ORIENTED_EDGE ( 'NONE', *, *, #70237, .F. ) ;
#4697=PLANE ( 'NONE',  #3032 ) ;
#4712=ORIENTED_EDGE ( 'NONE', *, *, #13239, .F. ) ;
#4717=ORIENTED_EDGE ( 'NONE', *, *, #71378, .T. ) ;
#4738=DIRECTION ( 'NONE',  ( 0.000000000000000000, 0.000000000000000000, -1.000000000000000000 ) ) ;
#4764=ORIENTED_EDGE ( 'NONE', *, *, #39152, .T. ) ;
#4765=EDGE_CURVE ( 'NONE', #7062, #74740, #81876, .T. ) ;
#4789=DIRECTION ( 'NONE',  ( -1.000000000000000000, -1.734723475976808672E-15, 0.000000000000000000 ) ) ;
#4803=EDGE_CURVE ( 'NONE', #31453, #63618, #67841, .T. ) ;
#4805=AXIS2_PLACEMENT_3D ( 'NONE', #33070, #54377, #19444 ) ;
#4809=FACE_OUTER_BOUND ( 'NONE', #78924, .T. ) ;
#4829=CARTESIAN_POINT ( 'NONE',  ( 77.11675609725448055, -140.6784471599409869, 245.5822774315739991 ) ) ;
#4838=DIRECTION ( 'NONE',  ( 1.000000000000000000, 0.000000000000000000, 0.000000000000000000 ) ) ;
#4848=CARTESIAN_POINT ( 'NONE',  ( 123.5667039024469886, -71.37844715994093292, 222.2178068554179902 ) ) ;
#4855=CARTESIAN_POINT ( 'NONE',  ( 92.91125933621934507, -113.6057974291314565, -11.78219314458173272 ) ) ;
#4872=ORIENTED_EDGE ( 'NONE', *, *, #37268, .T. ) ;
#4873=EDGE_CURVE ( 'NONE', #80721, #83896, #54180, .T. ) ;
#4874=ORIENTED_EDGE ( 'NONE', *, *, #88312, .T. ) ;
#4880=CARTESIAN_POINT ( 'NONE',  ( 87.66583711884676688, -139.6647249350598656, 247.4938686140749837 ) ) ;
#4882=CARTESIAN_POINT ( 'NONE',  ( 69.59601834107196794, -140.2077779303689908, 245.9389812651000113 ) ) ;
#4901=EDGE_CURVE ( 'NONE', #82261, #75851, #23145, .T. ) ;
#4915=ORIENTED_EDGE ( 'NONE', *, *, #50358, .T. ) ;
#4927=ORIENTED_EDGE ( 'NONE', *, *, #39896, .T. ) ;
#4951=CARTESIAN_POINT ( 'NONE',  ( 85.31670390244703128, -104.2784471599409670, 19.21780685541800437 ) ) ;
#4971=CARTESIAN_POINT ( 'NONE',  ( 108.5351697880554696, -105.7036166034834963, -19.78219314458196010 ) ) ;
#4976=CARTESIAN_POINT ( 'NONE',  ( 106.5667039024470313, -99.52844715994206126, -19.78219314458215550 ) ) ;
#4981=ORIENTED_EDGE ( 'NONE', *, *, #19440, .T. ) ;
#4984=PLANE ( 'NONE',  #41057 ) ;
#4993=AXIS2_PLACEMENT_3D ( 'NONE', #26299, #53975, #21740 ) ;
#5004=DIRECTION ( 'NONE',  ( 0.8660254037844387076, -0.4999999999999998335, 1.550000000000002231E-14 ) ) ;
#5030=EDGE_CURVE ( 'NONE', #48763, #65538, #23636, .T. ) ;
#5038=CIRCLE ( 'NONE', #54348, 24.50000000000000711 ) ;
#5040=ORIENTED_EDGE ( 'NONE', *, *, #14758, .T. ) ;
#5043=CARTESIAN_POINT ( 'NONE',  ( 117.0667039024470313, -104.2784471599412086, 7.717806855417980394 ) ) ;
#5054=LINE ( 'NONE', #60449, #40154 ) ;
#5059=CARTESIAN_POINT ( 'NONE',  ( 107.0667039024470313, -104.2784471599418197, -11.78219314458200984 ) ) ;
#5067=CARTESIAN_POINT ( 'NONE',  ( 162.0667039024469886, -68.87844715994089029, 55.21780685541800437 ) ) ;
#5089=FACE_OUTER_BOUND ( 'NONE', #13996, .T. ) ;
#5115=ORIENTED_EDGE ( 'NONE', *, *, #87035, .T. ) ;
#5120=CARTESIAN_POINT ( 'NONE',  ( 106.1586424053106299, -121.2541776101292186, -11.78219314458148226 ) ) ;
#5161=CARTESIAN_POINT ( 'NONE',  ( 56.06670390244700997, -79.67844715994098692, 85.21780685541799016 ) ) ;
#5174=EDGE_CURVE ( 'NONE', #45687, #15550, #19931, .T. ) ;
#5188=CARTESIAN_POINT ( 'NONE',  ( 140.0667039024470171, -90.27844715994091018, 51.21780685541800437 ) ) ;
#5224=CARTESIAN_POINT ( 'NONE',  ( 92.81551872686563343, -113.5468731908973723, -19.18411693322874356 ) ) ;
#5237=PLANE ( 'NONE',  #87148 ) ;
#5238=DIRECTION ( 'NONE',  ( 0.7118375500324360949, -0.7021341844428906631, 0.01717234406061140736 ) ) ;
#5243=VERTEX_POINT ( 'NONE', #75793 ) ;
#5253=ORIENTED_EDGE ( 'NONE', *, *, #11813, .T. ) ;
#5264=ORIENTED_EDGE ( 'NONE', *, *, #25267, .F. ) ;
#5285=EDGE_CURVE ( 'NONE', #87042, #9292, #46553, .T. ) ;
#5291=B_SPLINE_CURVE_WITH_KNOTS ( 'NONE', 3,
 ( #34983, #70420, #13656, #35884 ),
 .UNSPECIFIED., .F., .F.,
 ( 4, 4 ),
 ( -0.3974825557268110154, -0.3842043193313819938 ),
 .UNSPECIFIED. ) ;
#5304=CYLINDRICAL_SURFACE ( 'NONE', #27886, 4.500000000000003553 ) ;
#5356=VECTOR ( 'NONE', #78484, 1000.000000000000000 ) ;
#5377=ORIENTED_EDGE ( 'NONE', *, *, #9296, .F. ) ;
#5378=EDGE_LOOP ( 'NONE', ( #88618, #74920, #19766, #63380, #521, #25496 ) ) ;
#5382=DIRECTION ( 'NONE',  ( 1.000000000000000078E-15, -1.000000000000000000, 0.000000000000000000 ) ) ;
#5397=EDGE_CURVE ( 'NONE', #52525, #17066, #2630, .T. ) ;
#5398=CIRCLE ( 'NONE', #59056, 3.500000000000003109 ) ;
#5403=CARTESIAN_POINT ( 'NONE',  ( 90.06670420047028358, -131.9777253117771636, 222.2178068554179902 ) ) ;
#5413=ORIENTED_EDGE ( 'NONE', *, *, #57133, .T. ) ;
#5416=CARTESIAN_POINT ( 'NONE',  ( 107.0667039024470313, -104.2784471599409102, 17.71780685541799016 ) ) ;
#5425=CARTESIAN_POINT ( 'NONE',  ( 144.1872411114284773, -138.0587426716868151, 247.6570821702239869 ) ) ;
#5426=AXIS2_PLACEMENT_3D ( 'NONE', #64233, #7475, #43317 ) ;
#5459=VECTOR ( 'NONE', #11881, 1000.000000000000000 ) ;
#5461=VERTEX_POINT ( 'NONE', #3952 ) ;
#5468=CYLINDRICAL_SURFACE ( 'NONE', #34455, 1.999999999999995781 ) ;
#5499=EDGE_CURVE ( 'NONE', #33876, #11706, #66860, .T. ) ;
#5527=EDGE_LOOP ( 'NONE', ( #19094, #2058, #66080, #20754 ) ) ;
#5548=CARTESIAN_POINT ( 'NONE',  ( 70.56670390244700286, -68.87844715994098976, 222.2178068554179902 ) ) ;
#5555=AXIS2_PLACEMENT_3D ( 'NONE', #2749, #43157, #77256 ) ;
#5559=CARTESIAN_POINT ( 'NONE',  ( 144.9829487194917590, -139.7622023428961029, 245.5930228935639832 ) ) ;
#5560=CARTESIAN_POINT ( 'NONE',  ( 127.3855720247629222, -85.76459861161312404, 250.2191008560389776 ) ) ;
#5574=ORIENTED_EDGE ( 'NONE', *, *, #86507, .F. ) ;
#5586=CARTESIAN_POINT ( 'NONE',  ( 106.1656040943334460, -121.2545485715091047, -11.78219314458148226 ) ) ;
#5592=LINE ( 'NONE', #12858, #82256 ) ;
#5596=VECTOR ( 'NONE', #39950, 1000.000000000000000 ) ;
#5605=EDGE_CURVE ( 'NONE', #75812, #26236, #75241, .T. ) ;
#5613=FACE_OUTER_BOUND ( 'NONE', #66534, .T. ) ;
#5619=ORIENTED_EDGE ( 'NONE', *, *, #51143, .F. ) ;
#5639=ORIENTED_EDGE ( 'NONE', *, *, #63169, .F. ) ;
#5642=DIRECTION ( 'NONE',  ( 1.000000000000000000, 0.000000000000000000, 0.000000000000000000 ) ) ;
#5647=CARTESIAN_POINT ( 'NONE',  ( 107.0667039024470313, -104.2784471599409528, 45.21780685541799727 ) ) ;
#5649=CARTESIAN_POINT ( 'NONE',  ( 92.91125933621934507, -113.6057974291316981, -19.26696060647573105 ) ) ;
#5678=DIRECTION ( 'NONE',  ( 1.000000000000000000, 1.000000000000000078E-15, 0.000000000000000000 ) ) ;
#5692=DIRECTION ( 'NONE',  ( -3.100000000000000258E-29, 3.100000000000000044E-14, 1.000000000000000000 ) ) ;
#5693=DIRECTION ( 'NONE',  ( -0.09234423430305457869, -0.06932666101729537123, 0.9933108055705301975 ) ) ;
#5704=CARTESIAN_POINT ( 'NONE',  ( 122.2221484686747459, -107.5284471599419192, -21.78219314458190681 ) ) ;
#5707=DIRECTION ( 'NONE',  ( -3.100000000000000258E-29, 3.100000000000000044E-14, 1.000000000000000000 ) ) ;
#5756=DIRECTION ( 'NONE',  ( 1.000000000000000000, 0.000000000000000000, 0.000000000000000000 ) ) ;
#5783=CARTESIAN_POINT ( 'NONE',  ( 113.5015236877822389, -120.9585416479406348, -9.274842254010115639 ) ) ;
#5785=CARTESIAN_POINT ( 'NONE',  ( 145.4449125191942187, -139.3071378063975203, 245.7427791856104875 ) ) ;
#5792=ORIENTED_EDGE ( 'NONE', *, *, #53890, .F. ) ;
#5794=DIRECTION ( 'NONE',  ( -1.000000000000000000, -1.000000000000000078E-15, 0.000000000000000000 ) ) ;
#5798=EDGE_CURVE ( 'NONE', #960, #25814, #3136, .T. ) ;
#5802=EDGE_CURVE ( 'NONE', #75262, #34651, #57469, .T. ) ;
#5809=EDGE_CURVE ( 'NONE', #33347, #54218, #77122, .T. ) ;
#5816=EDGE_CURVE ( 'NONE', #33347, #61554, #35229, .T. ) ;
#5821=ORIENTED_EDGE ( 'NONE', *, *, #41372, .T. ) ;
#5825=ADVANCED_FACE ( 'NONE', ( #83853, #63852 ), #714, .T. ) ;
#5840=ORIENTED_EDGE ( 'NONE', *, *, #23811, .T. ) ;
#5848=ADVANCED_FACE ( 'NONE', ( #7093 ), #15257, .T. ) ;
#5863=CARTESIAN_POINT ( 'NONE',  ( 107.0667039024470313, -104.2784471599418197, -11.78219314458200984 ) ) ;
#5868=DIRECTION ( 'NONE',  ( 0.08219486863338737459, 0.05370816768103092026, 0.9951680442491540601 ) ) ;
#5878=CARTESIAN_POINT ( 'NONE',  ( 63.06670390244700997, -79.67844715994098692, 120.2178068554179902 ) ) ;
#5893=CARTESIAN_POINT ( 'NONE',  ( 52.06670390244700286, -77.67844715994100113, 180.4678068554179902 ) ) ;
#5922=EDGE_CURVE ( 'NONE', #14739, #67885, #32103, .T. ) ;
#5929=ORIENTED_EDGE ( 'NONE', *, *, #30363, .T. ) ;
#5940=EDGE_CURVE ( 'NONE', #11071, #61542, #58361, .T. ) ;
#5965=VERTEX_POINT ( 'NONE', #64739 ) ;
#5968=DIRECTION ( 'NONE',  ( 0.000000000000000000, 0.000000000000000000, 1.000000000000000000 ) ) ;
#5980=AXIS2_PLACEMENT_3D ( 'NONE', #38848, #5238, #5693 ) ;
#6023=CARTESIAN_POINT ( 'NONE',  ( 144.0667052733537901, -83.77844715994089597, 55.21780685541800437 ) ) ;
#6036=EDGE_CURVE ( 'NONE', #57999, #76564, #46678, .T. ) ;
#6040=DIRECTION ( 'NONE',  ( 0.7071067811865446862, -0.7071067811865504593, 0.000000000000000000 ) ) ;
#6041=B_SPLINE_SURFACE_WITH_KNOTS ( 'NONE', 3, 3, ( 
 ( #46816, #74104, #23846, #64722 ),
 ( #25959, #79261, #74549, #65162 ),
 ( #17023, #44706, #64285, #11429 ),
 ( #2057, #39131, #32303, #87732 ),
 ( #25504, #46370, #57447, #85189 ),
 ( #22961, #78376, #51078, #16138 ),
 ( #71554, #37017, #61356, #67738 ) ),
 .UNSPECIFIED., .F., .F., .F.,
 ( 4, 1, 1, 1, 4 ),
 ( 4, 4 ),
 ( -0.0004298309602272039798, 0.2857142857142860315, 0.5714285714285709528, 0.8571428571428569843, 1.000429830960229971 ),
 ( 0.08686432420013849576, 1.000429830960229971 ),
 .UNSPECIFIED. ) ;
#6057=CIRCLE ( 'NONE', #51036, 175.7032523792620111 ) ;
#6063=DIRECTION ( 'NONE',  ( 1.000000000000000000, 0.000000000000000000, 0.000000000000000000 ) ) ;
#6068=ORIENTED_EDGE ( 'NONE', *, *, #82003, .F. ) ;
#6097=CARTESIAN_POINT ( 'NONE',  ( 106.5667039024470313, -108.2470741265389620, -19.78219314458190681 ) ) ;
#6124=EDGE_CURVE ( 'NONE', #1539, #13040, #66964, .T. ) ;
#6132=DIRECTION ( 'NONE',  ( 1.000000000000000078E-15, -1.000000000000000000, 0.000000000000000000 ) ) ;
#6137=CARTESIAN_POINT ( 'NONE',  ( 107.5667039024470313, -100.3098201933451605, -19.78219314458212708 ) ) ;
#6140=CARTESIAN_POINT ( 'NONE',  ( 144.1741131095133994, -138.0461895383712942, 247.6591799766680140 ) ) ;
#6149=ORIENTED_EDGE ( 'NONE', *, *, #14150, .T. ) ;
#6168=CARTESIAN_POINT ( 'NONE',  ( 158.0667039024469886, -67.87844715994090450, 85.21780685541799016 ) ) ;
#6170=ORIENTED_EDGE ( 'NONE', *, *, #39839, .T. ) ;
#6176=EDGE_CURVE ( 'NONE', #1337, #53380, #82971, .T. ) ;
#6177=AXIS2_PLACEMENT_3D ( 'NONE', #63854, #43383, #64303 ) ;
#6192=DIRECTION ( 'NONE',  ( -3.100000000000000258E-29, 3.100000000000000044E-14, 1.000000000000000000 ) ) ;
#6224=ORIENTED_EDGE ( 'NONE', *, *, #69511, .T. ) ;
#6227=CARTESIAN_POINT ( 'NONE',  ( 107.5667039024470455, -113.7784471599420613, -19.78219314458171141 ) ) ;
#6234=ORIENTED_EDGE ( 'NONE', *, *, #59230, .T. ) ;
#6242=AXIS2_PLACEMENT_3D ( 'NONE', #76921, #14249, #8788 ) ;
#6257=VECTOR ( 'NONE', #72913, 1000.000000000000000 ) ;
#6264=CARTESIAN_POINT ( 'NONE',  ( 74.67063729340679856, -69.52133568612056536, 247.5307829608580050 ) ) ;
#6282=ORIENTED_EDGE ( 'NONE', *, *, #88739, .F. ) ;
#6293=CARTESIAN_POINT ( 'NONE',  ( 107.5667039024470313, -100.3098201933444926, 2.217806855417892020 ) ) ;
#6294=CARTESIAN_POINT ( 'NONE',  ( 56.06670390244700997, -79.67844715994098692, 120.2178068554179902 ) ) ;
#6300=DIRECTION ( 'NONE',  ( 0.7017307308178937220, -0.7121747104280534701, -0.01952340268762070216 ) ) ;
#6310=ORIENTED_EDGE ( 'NONE', *, *, #55368, .T. ) ;
#6329=DIRECTION ( 'NONE',  ( 1.000000000000000000, 1.000000000000000078E-15, 0.000000000000000000 ) ) ;
#6333=DIRECTION ( 'NONE',  ( 0.000000000000000000, 0.000000000000000000, 1.000000000000000000 ) ) ;
#6395=ORIENTED_EDGE ( 'NONE', *, *, #72472, .F. ) ;
#6414=CARTESIAN_POINT ( 'NONE',  ( 117.0467990990870675, -131.0263588434231110, 250.2203867545810283 ) ) ;
#6419=ORIENTED_EDGE ( 'NONE', *, *, #7776, .F. ) ;
#6425=CARTESIAN_POINT ( 'NONE',  ( 158.0667039024469886, -67.87844715994090450, 120.2178068554179902 ) ) ;
#6429=EDGE_CURVE ( 'NONE', #58142, #24085, #13382, .T. ) ;
#6441=CARTESIAN_POINT ( 'NONE',  ( 135.1911801492854011, -84.41530667025313051, 249.3055338466990065 ) ) ;
#6442=EDGE_LOOP ( 'NONE', ( #81703, #80864, #13278, #43018, #80926, #20940 ) ) ;
#6466=DIRECTION ( 'NONE',  ( -3.100000000000000258E-29, 3.100000000000000044E-14, 1.000000000000000000 ) ) ;
#6520=ORIENTED_EDGE ( 'NONE', *, *, #66494, .F. ) ;
#6588=CIRCLE ( 'NONE', #58759, 3.499999999999996003 ) ;
#6592=CARTESIAN_POINT ( 'NONE',  ( 104.0667030381801936, -70.87844715994094713, 173.2178086137559774 ) ) ;
#6602=ORIENTED_EDGE ( 'NONE', *, *, #38525, .F. ) ;
#6610=ORIENTED_EDGE ( 'NONE', *, *, #82344, .T. ) ;
#6629=CARTESIAN_POINT ( 'NONE',  ( 69.56670390244704549, -118.2784471599409812, 45.21780685541799727 ) ) ;
#6660=CARTESIAN_POINT ( 'NONE',  ( 107.0667039024469886, -70.87844715994094713, 93.21780685541800437 ) ) ;
#6663=EDGE_LOOP ( 'NONE', ( #44477, #73581 ) ) ;
#6676=VERTEX_POINT ( 'NONE', #6425 ) ;
#6699=DIRECTION ( 'NONE',  ( 0.000000000000000000, 0.000000000000000000, -1.000000000000000000 ) ) ;
#6706=CARTESIAN_POINT ( 'NONE',  ( 67.05444493988859733, -69.17499946017586865, 247.4285673639549827 ) ) ;
#6712=( BOUNDED_CURVE ( )  B_SPLINE_CURVE ( 3, ( #29501, #58964, #85827, #57184 ),
 .UNSPECIFIED., .F., .T. ) 
 B_SPLINE_CURVE_WITH_KNOTS ( ( 4, 4 ),
 ( 5.813027347256379151, 6.753343267102791536 ),
 .UNSPECIFIED. ) 
 CURVE ( )  GEOMETRIC_REPRESENTATION_ITEM ( )  RATIONAL_B_SPLINE_CURVE ( ( 1.000000000000000000, 0.9276644927932374829, 0.9276644927932374829, 1.000000000000000000 ) ) 
 REPRESENTATION_ITEM ( '' )  );
#6729=ADVANCED_FACE ( 'NONE', ( #21409 ), #89554, .T. ) ;
#6750=CARTESIAN_POINT ( 'NONE',  ( 107.0667039024470313, -104.2784471599420755, -19.78219314458201694 ) ) ;
#6776=EDGE_CURVE ( 'NONE', #38828, #71132, #1820, .T. ) ;
#6778=EDGE_LOOP ( 'NONE', ( #30179, #38020, #19796, #18154 ) ) ;
#6794=DIRECTION ( 'NONE',  ( -0.000000000000000000, -0.000000000000000000, -1.000000000000000000 ) ) ;
#6806=EDGE_CURVE ( 'NONE', #59337, #59214, #36383, .T. ) ;
#6809=CARTESIAN_POINT ( 'NONE',  ( 107.0667039024470313, -104.2784471599421323, -21.78219314458201694 ) ) ;
#6810=AXIS2_PLACEMENT_3D ( 'NONE', #48859, #14378, #28434 ) ;
#6846=CARTESIAN_POINT ( 'NONE',  ( 78.56670390244701707, -90.27844715994098124, 51.21780685541800437 ) ) ;
#6854=VERTEX_POINT ( 'NONE', #64533 ) ;
#6863=CARTESIAN_POINT ( 'NONE',  ( 68.78290018810869810, -67.86861087870656206, 247.4717563792629846 ) ) ;
#6874=DIRECTION ( 'NONE',  ( 0.000000000000000000, 0.000000000000000000, 1.000000000000000000 ) ) ;
#6883=CIRCLE ( 'NONE', #80887, 4.500000000000003553 ) ;
#6885=CARTESIAN_POINT ( 'NONE',  ( 132.1532570847676595, -116.6569832596315166, 250.2191008560389776 ) ) ;
#6896=CARTESIAN_POINT ( 'NONE',  ( 67.78013389119247734, -136.6656689513177696, 247.3338295459389826 ) ) ;
#6928=ADVANCED_FACE ( 'NONE', ( #3634, #60261 ), #87993, .T. ) ;
#6942=ORIENTED_EDGE ( 'NONE', *, *, #70237, .T. ) ;
#6944=CARTESIAN_POINT ( 'NONE',  ( 107.0667039024470313, -104.2784471599409528, 222.2178068554179902 ) ) ;
#6950=EDGE_LOOP ( 'NONE', ( #51440, #38418, #68909, #17358 ) ) ;
#6986=CARTESIAN_POINT ( 'NONE',  ( 107.0667039024470313, -104.2784471599420755, -19.78219314458201694 ) ) ;
#6997=VECTOR ( 'NONE', #73521, 1000.000000000000000 ) ;
#7000=DIRECTION ( 'NONE',  ( -1.000000000000000000, -1.734723475976808672E-15, 0.000000000000000000 ) ) ;
#7013=ORIENTED_EDGE ( 'NONE', *, *, #30020, .F. ) ;
#7023=CARTESIAN_POINT ( 'NONE',  ( 90.69304023831777783, -109.5826158781451340, -10.56397404668060780 ) ) ;
#7034=AXIS2_PLACEMENT_3D ( 'NONE', #26127, #53795, #67003 ) ;
#7040=LINE ( 'NONE', #48792, #36648 ) ;
#7049=VECTOR ( 'NONE', #29422, 1000.000000000000000 ) ;
#7050=LINE ( 'NONE', #68830, #34635 ) ;
#7062=VERTEX_POINT ( 'NONE', #28905 ) ;
#7093=FACE_OUTER_BOUND ( 'NONE', #29007, .T. ) ;
#7140=EDGE_CURVE ( 'NONE', #68199, #3973, #46633, .T. ) ;
#7171=LINE ( 'NONE', #63466, #86584 ) ;
#7181=CARTESIAN_POINT ( 'NONE',  ( 97.81670390244700286, -67.87844715994096134, 222.2178068554179902 ) ) ;
#7185=ORIENTED_EDGE ( 'NONE', *, *, #8377, .T. ) ;
#7190=ORIENTED_EDGE ( 'NONE', *, *, #23703, .F. ) ;
#7202=CARTESIAN_POINT ( 'NONE',  ( 129.7322073617410751, -147.4828892792592399, 72.80491793818269741 ) ) ;
#7229=CARTESIAN_POINT ( 'NONE',  ( 107.0667039024470597, -133.7784471599409528, 25.71780685541800437 ) ) ;
#7232=CARTESIAN_POINT ( 'NONE',  ( 162.0667039024469886, -68.87844715994089029, 222.2178068554179902 ) ) ;
#7233=DIRECTION ( 'NONE',  ( -0.7071067811865453523, -0.7071067811865496822, 0.000000000000000000 ) ) ;
#7258=DIRECTION ( 'NONE',  ( -3.100000000000000258E-29, 3.100000000000000044E-14, 1.000000000000000000 ) ) ;
#7267=ORIENTED_EDGE ( 'NONE', *, *, #75622, .T. ) ;
#7269=AXIS2_PLACEMENT_3D ( 'NONE', #35245, #42949, #69784 ) ;
#7272=DIRECTION ( 'NONE',  ( -0.9999999999998281375, 0.000000000000000000, 5.861124988064729938E-07 ) ) ;
#7278=VECTOR ( 'NONE', #36907, 1000.000000000000000 ) ;
#7298=FACE_OUTER_BOUND ( 'NONE', #46385, .T. ) ;
#7313=DIRECTION ( 'NONE',  ( -1.087812297297669405E-15, 1.000000000000000000, -3.100000000000000044E-14 ) ) ;
#7328=CARTESIAN_POINT ( 'NONE',  ( 118.5667039024470313, -104.2784471599411376, 17.71780685541799016 ) ) ;
#7335=VECTOR ( 'NONE', #54998, 1000.000000000000000 ) ;
#7351=EDGE_CURVE ( 'NONE', #36821, #75352, #80186, .T. ) ;
#7353=CARTESIAN_POINT ( 'NONE',  ( 67.17963690485876782, -137.3494469986182764, 246.8019061136969867 ) ) ;
#7369=EDGE_CURVE ( 'NONE', #52825, #27442, #31113, .T. ) ;
#7384=ORIENTED_EDGE ( 'NONE', *, *, #59975, .F. ) ;
#7390=AXIS2_PLACEMENT_3D ( 'NONE', #33918, #70259, #36186 ) ;
#7391=DIRECTION ( 'NONE',  ( 1.000000000000000078E-15, -1.000000000000000000, 0.000000000000000000 ) ) ;
#7400=DIRECTION ( 'NONE',  ( -0.000000000000000000, -0.000000000000000000, 1.000000000000000000 ) ) ;
#7421=DIRECTION ( 'NONE',  ( -1.000000000000000078E-15, 1.000000000000000000, -3.100000000000000044E-14 ) ) ;
#7423=CARTESIAN_POINT ( 'NONE',  ( 68.69171528984767860, -139.3034585473416769, 245.6607614303540004 ) ) ;
#7434=ORIENTED_EDGE ( 'NONE', *, *, #61383, .T. ) ;
#7440=DIRECTION ( 'NONE',  ( 0.7071067811865503483, 0.7071067811865445751, 0.000000000000000000 ) ) ;
#7449=DIRECTION ( 'NONE',  ( -3.100000000000000258E-29, 3.100000000000000044E-14, 1.000000000000000000 ) ) ;
#7458=EDGE_CURVE ( 'NONE', #37406, #65511, #13810, .T. ) ;
#7469=CARTESIAN_POINT ( 'NONE',  ( 134.5667039024471023, -105.9704134719595601, 250.2178068554179902 ) ) ;
#7475=DIRECTION ( 'NONE',  ( 5.440892098500631367E-15, -1.000000000000000000, 3.100000000000000044E-14 ) ) ;
#7483=AXIS2_PLACEMENT_3D ( 'NONE', #8442, #14363, #62935 ) ;
#7504=ORIENTED_EDGE ( 'NONE', *, *, #24315, .T. ) ;
#7511=ORIENTED_EDGE ( 'NONE', *, *, #32436, .F. ) ;
#7512=ORIENTED_EDGE ( 'NONE', *, *, #19440, .F. ) ;
#7545=ADVANCED_FACE ( 'NONE', ( #26102 ), #61056, .T. ) ;
#7550=CARTESIAN_POINT ( 'NONE',  ( 146.5536166493005226, -137.3844657570545564, 246.8455049394716809 ) ) ;
#7580=ORIENTED_EDGE ( 'NONE', *, *, #8070, .T. ) ;
#7593=CIRCLE ( 'NONE', #62694, 17.00000000000000000 ) ;
#7594=ORIENTED_EDGE ( 'NONE', *, *, #51478, .T. ) ;
#7631=ORIENTED_EDGE ( 'NONE', *, *, #40285, .T. ) ;
#7636=CYLINDRICAL_SURFACE ( 'NONE', #44553, 3.500000000000003109 ) ;
#7637=ADVANCED_FACE ( 'NONE', ( #22881 ), #42389, .F. ) ;
#7644=DIRECTION ( 'NONE',  ( 0.000000000000000000, 0.000000000000000000, 1.000000000000000000 ) ) ;
#7650=DIRECTION ( 'NONE',  ( -3.100000000000000258E-29, 3.100000000000000044E-14, 1.000000000000000000 ) ) ;
#7652=EDGE_CURVE ( 'NONE', #22487, #20369, #62399, .T. ) ;
#7671=CARTESIAN_POINT ( 'NONE',  ( 143.0667039024470171, -83.77844715994091018, 55.21780685541800437 ) ) ;
#7699=CARTESIAN_POINT ( 'NONE',  ( 107.0667039024470313, -104.2784471599418197, -11.78219314458200984 ) ) ;
#7714=LINE ( 'NONE', #30397, #14577 ) ;
#7731=LINE ( 'NONE', #8182, #68030 ) ;
#7736=CARTESIAN_POINT ( 'NONE',  ( 121.2862988949694483, -113.5675617909524817, -19.21044887263773049 ) ) ;
#7763=CARTESIAN_POINT ( 'NONE',  ( 107.0667039024470313, -104.2784471599421323, -21.78219314458201694 ) ) ;
#7767=LINE ( 'NONE', #63624, #1684 ) ;
#7776=EDGE_CURVE ( 'NONE', #47465, #51228, #45057, .T. ) ;
#7783=LINE ( 'NONE', #35471, #74148 ) ;
#7794=CARTESIAN_POINT ( 'NONE',  ( 89.44289600121240369, -83.08196156581377068, 250.2178068554179902 ) ) ;
#7805=AXIS2_PLACEMENT_3D ( 'NONE', #55343, #29018, #76713 ) ;
#7834=CARTESIAN_POINT ( 'NONE',  ( 107.0667039024470313, -104.2784471599409528, 23.21780685541800082 ) ) ;
#7855=CARTESIAN_POINT ( 'NONE',  ( 61.06670403655746782, -83.77844715994098124, 55.21780685541800437 ) ) ;
#7856=CARTESIAN_POINT ( 'NONE',  ( 70.35947989645553946, -140.1803810602137617, 246.8545327174207387 ) ) ;
#7867=VECTOR ( 'NONE', #23528, 1000.000000000000000 ) ;
#7869=LINE ( 'NONE', #69652, #12638 ) ;
#7880=CARTESIAN_POINT ( 'NONE',  ( 92.91125933621933086, -94.95109689075242443, -19.26696060647628528 ) ) ;
#7889=CARTESIAN_POINT ( 'NONE',  ( 107.5667039024470313, -108.2470741265389620, -19.78219314458190681 ) ) ;
#7891=EDGE_LOOP ( 'NONE', ( #32107, #84662, #32304, #2160 ) ) ;
#7895=CARTESIAN_POINT ( 'NONE',  ( 91.91125933621933086, -101.0284471599423739, -21.78219314458213063 ) ) ;
#7897=LINE ( 'NONE', #35596, #31580 ) ;
#7909=CIRCLE ( 'NONE', #81907, 3.500000000000003109 ) ;
#7911=FACE_OUTER_BOUND ( 'NONE', #33733, .T. ) ;
#7914=CIRCLE ( 'NONE', #42710, 4.000000000000002665 ) ;
#7918=DIRECTION ( 'NONE',  ( -1.000000000000000000, -1.541976423090496028E-15, 0.000000000000000000 ) ) ;
#7920=CARTESIAN_POINT ( 'NONE',  ( 67.58630777427835312, -68.37784050924791757, 246.8383462433463933 ) ) ;
#7930=EDGE_CURVE ( 'NONE', #67598, #66630, #40745, .T. ) ;
#7934=CIRCLE ( 'NONE', #58680, 4.500000000000003553 ) ;
#7938=ORIENTED_EDGE ( 'NONE', *, *, #69390, .T. ) ;
#7966=PLANE ( 'NONE',  #65500 ) ;
#7998=EDGE_CURVE ( 'NONE', #1864, #11319, #83651, .T. ) ;
#8004=LINE ( 'NONE', #22995, #29369 ) ;
#8010=CONICAL_SURFACE ( 'NONE', #28276, 24.50000000000000711, 0.7419472680059182590 ) ;
#8011=VERTEX_POINT ( 'NONE', #64102 ) ;
#8016=CARTESIAN_POINT ( 'NONE',  ( 70.06964507117767482, -140.6784471599286519, 245.5331643397809671 ) ) ;
#8044=CARTESIAN_POINT ( 'NONE',  ( 107.0667039024470313, -119.4690460831836276, -21.78219314458154798 ) ) ;
#8048=ADVANCED_FACE ( 'NONE', ( #42283 ), #84559, .T. ) ;
#8049=CARTESIAN_POINT ( 'NONE',  ( 115.0439452383992318, -109.4614598618342853, -19.78219314458184996 ) ) ;
#8070=EDGE_CURVE ( 'NONE', #17172, #39484, #42723, .T. ) ;
#8083=CARTESIAN_POINT ( 'NONE',  ( 107.0667039024470313, -104.2784471599420755, -19.78219314458201694 ) ) ;
#8096=DIRECTION ( 'NONE',  ( 1.000000000000000000, 1.000000000000000078E-15, 0.000000000000000000 ) ) ;
#8100=EDGE_CURVE ( 'NONE', #67885, #54402, #7783, .T. ) ;
#8118=CARTESIAN_POINT ( 'NONE',  ( 106.5667039024470313, -108.2470741265382799, 2.217806855418114065 ) ) ;
#8120=CARTESIAN_POINT ( 'NONE',  ( 114.6444261855607891, -91.15344715994180547, -11.78219314458242550 ) ) ;
#8122=PLANE ( 'NONE',  #78712 ) ;
#8147=DIRECTION ( 'NONE',  ( -1.000000000000000000, 0.000000000000000000, 0.000000000000000000 ) ) ;
#8154=ORIENTED_EDGE ( 'NONE', *, *, #53746, .T. ) ;
#8168=CARTESIAN_POINT ( 'NONE',  ( 68.91169813362903085, -69.55710376154327435, 247.4994584470433381 ) ) ;
#8182=CARTESIAN_POINT ( 'NONE',  ( 52.06670390244699576, -67.87844715994100397, 55.21780685541800437 ) ) ;
#8183=DIRECTION ( 'NONE',  ( 1.000000000000000000, 5.440892098500631367E-15, -1.376676550535195643E-28 ) ) ;
#8189=ORIENTED_EDGE ( 'NONE', *, *, #75557, .F. ) ;
#8216=ORIENTED_EDGE ( 'NONE', *, *, #16078, .T. ) ;
#8219=CARTESIAN_POINT ( 'NONE',  ( 67.06670390244707392, -137.6779871412748832, 245.9128651760420041 ) ) ;
#8224=PRESENTATION_STYLE_ASSIGNMENT (( #77716 ) ) ;
#8267=FACE_OUTER_BOUND ( 'NONE', #9614, .T. ) ;
#8279=CARTESIAN_POINT ( 'NONE',  ( 120.2221484686747317, -96.68314769832136335, -21.78219314458224076 ) ) ;
#8303=FACE_OUTER_BOUND ( 'NONE', #76421, .T. ) ;
#8307=CARTESIAN_POINT ( 'NONE',  ( 107.5667039024470455, -113.7784471599420613, -19.78219314458171141 ) ) ;
#8308=LINE ( 'NONE', #1500, #29453 ) ;
#8315=CARTESIAN_POINT ( 'NONE',  ( 70.55471543514235577, -139.7618167078771023, 247.2193956393660983 ) ) ;
#8319=CYLINDRICAL_SURFACE ( 'NONE', #87204, 3.499999999999996003 ) ;
#8325=FACE_OUTER_BOUND ( 'NONE', #20911, .T. ) ;
#8327=LINE ( 'NONE', #55537, #13770 ) ;
#8369=CARTESIAN_POINT ( 'NONE',  ( 107.0667039024470313, -104.2784471599408676, 19.21780685541799016 ) ) ;
#8371=CARTESIAN_POINT ( 'NONE',  ( 70.06871658682176474, -140.6784471599409869, 245.5179332689559999 ) ) ;
#8377=EDGE_CURVE ( 'NONE', #79697, #6854, #40398, .T. ) ;
#8378=CARTESIAN_POINT ( 'NONE',  ( 67.45090841991523689, -68.24843840015816454, 246.6732856276495909 ) ) ;
#8391=AXIS2_PLACEMENT_3D ( 'NONE', #72589, #17177, #10353 ) ;
#8392=VECTOR ( 'NONE', #46829, 1000.000000000000000 ) ;
#8394=DIRECTION ( 'NONE',  ( 1.000000000000000000, 0.000000000000000000, 0.000000000000000000 ) ) ;
#8399=CIRCLE ( 'NONE', #59135, 21.75000000000000711 ) ;
#8400=CARTESIAN_POINT ( 'NONE',  ( 135.5667039024470171, -90.27844715994091018, 51.21780685541800437 ) ) ;
#8404=CARTESIAN_POINT ( 'NONE',  ( 143.2710647978358054, -69.54852422598250428, 247.5103554657479776 ) ) ;
#8414=ORIENTED_EDGE ( 'NONE', *, *, #29367, .T. ) ;
#8415=AXIS2_PLACEMENT_3D ( 'NONE', #78203, #15516, #39406 ) ;
#8438=DIRECTION ( 'NONE',  ( -1.000000000000000000, -8.540177112501204385E-16, 0.000000000000000000 ) ) ;
#8439=DIRECTION ( 'NONE',  ( -1.000000000000000000, -1.206764157201257538E-15, 0.000000000000000000 ) ) ;
#8442=CARTESIAN_POINT ( 'NONE',  ( 74.06670390244701707, -90.27844715994098124, 51.21780685541800437 ) ) ;
#8447=CARTESIAN_POINT ( 'NONE',  ( 146.5179483142460128, -137.3672551618605269, 246.8848049447683763 ) ) ;
#8468=AXIS2_PLACEMENT_3D ( 'NONE', #19654, #12859, #81464 ) ;
#8500=CIRCLE ( 'NONE', #2668, 3.500000000000003109 ) ;
#8505=EDGE_CURVE ( 'NONE', #3053, #49629, #34019, .T. ) ;
#8506=DIRECTION ( 'NONE',  ( 1.000000000000000000, 8.953411488912556626E-16, 0.000000000000000000 ) ) ;
#8507=ORIENTED_EDGE ( 'NONE', *, *, #32673, .F. ) ;
#8512=CARTESIAN_POINT ( 'NONE',  ( 76.06670390244703128, -104.2784471599409812, 25.71780685541800437 ) ) ;
#8520=CIRCLE ( 'NONE', #65057, 15.50000000000000000 ) ;
#8563=AXIS2_PLACEMENT_3D ( 'NONE', #60502, #74596, #32349 ) ;
#8567=ORIENTED_EDGE ( 'NONE', *, *, #86852, .F. ) ;
#8570=ORIENTED_EDGE ( 'NONE', *, *, #77192, .F. ) ;
#8577=ADVANCED_FACE ( 'NONE', ( #22213 ), #49888, .T. ) ;
#8590=EDGE_CURVE ( 'NONE', #16335, #48763, #48088, .T. ) ;
#8611=DIRECTION ( 'NONE',  ( -1.000000000000000078E-15, 1.000000000000000000, 0.000000000000000000 ) ) ;
#8632=ORIENTED_EDGE ( 'NONE', *, *, #25255, .T. ) ;
#8665=AXIS2_PLACEMENT_3D ( 'NONE', #71975, #85616, #85167 ) ;
#8667=COLOUR_RGB ( '', 0.66274510, 0.83137255, 0.94901961) ;
#8679=SURFACE_SIDE_STYLE ('',( #22304 ) ) ;
#8692=EDGE_CURVE ( 'NONE', #23885, #31453, #63990, .T. ) ;
#8704=AXIS2_PLACEMENT_3D ( 'NONE', #17853, #43769, #31036 ) ;
#8708=CARTESIAN_POINT ( 'NONE',  ( 97.69261636184602082, -78.35517403977323170, 250.2178068554180470 ) ) ;
#8746=DIRECTION ( 'NONE',  ( -7.559289460184342508E-16, 0.7559289460184340781, -0.6546536707080007345 ) ) ;
#8755=ORIENTED_EDGE ( 'NONE', *, *, #71273, .T. ) ;
#8759=EDGE_LOOP ( 'NONE', ( #15462, #58081, #53631, #61782 ) ) ;
#8767=VERTEX_POINT ( 'NONE', #28863 ) ;
#8772=CARTESIAN_POINT ( 'NONE',  ( 70.65700412096775551, -139.5313073890320368, 247.3443455604209760 ) ) ;
#8777=EDGE_LOOP ( 'NONE', ( #27747, #33110, #33191, #81616 ) ) ;
#8788=DIRECTION ( 'NONE',  ( 0.7759704746411385523, -0.6307692307692301936, 0.000000000000000000 ) ) ;
#8791=EDGE_CURVE ( 'NONE', #49629, #51345, #55894, .T. ) ;
#8796=EDGE_LOOP ( 'NONE', ( #37537, #4238 ) ) ;
#8798=CARTESIAN_POINT ( 'NONE',  ( 97.69261636184624820, -130.2017202801087876, 250.2178068554180470 ) ) ;
#8808=DIRECTION ( 'NONE',  ( -1.000000000000000000, -8.540177112501204385E-16, 0.000000000000000000 ) ) ;
#8821=ADVANCED_FACE ( 'NONE', ( #696 ), #28360, .T. ) ;
#8822=CARTESIAN_POINT ( 'NONE',  ( 147.0667039036620451, -137.6784471587259020, 245.4218662566639750 ) ) ;
#8834=DIRECTION ( 'NONE',  ( 0.000000000000000000, 0.000000000000000000, -1.000000000000000000 ) ) ;
#8842=VECTOR ( 'NONE', #62070, 1000.000000000000000 ) ;
#8844=CARTESIAN_POINT ( 'NONE',  ( 145.4407362117956097, -69.39660493469676794, 247.4650063441803809 ) ) ;
#8846=LINE ( 'NONE', #37428, #84515 ) ;
#8853=ORIENTED_EDGE ( 'NONE', *, *, #79635, .F. ) ;
#8857=PLANE ( 'NONE',  #25890 ) ;
#8874=VERTEX_POINT ( 'NONE', #14796 ) ;
#8875=CIRCLE ( 'NONE', #53752, 175.7032523735949781 ) ;
#8883=DIRECTION ( 'NONE',  ( 1.000000000000000000, 1.000000000000000078E-15, -0.000000000000000000 ) ) ;
#8894=CARTESIAN_POINT ( 'NONE',  ( 91.91125933621934507, -107.5284471599419049, -21.78219314458190681 ) ) ;
#8903=EDGE_CURVE ( 'NONE', #48200, #21095, #17022, .T. ) ;
#8925=ADVANCED_FACE ( 'NONE', ( #16137 ), #30204, .T. ) ;
#8930=ORIENTED_EDGE ( 'NONE', *, *, #36053, .T. ) ;
#8943=FACE_OUTER_BOUND ( 'NONE', #20353, .T. ) ;
#8950=DIRECTION ( 'NONE',  ( 1.000000000000000000, 1.000000000000000078E-15, -0.000000000000000000 ) ) ;
#8959=ORIENTED_EDGE ( 'NONE', *, *, #7652, .T. ) ;
#8966=DIRECTION ( 'NONE',  ( 0.000000000000000000, 0.000000000000000000, 1.000000000000000000 ) ) ;
#8981=DIRECTION ( 'NONE',  ( 0.000000000000000000, 0.000000000000000000, -1.000000000000000000 ) ) ;
#9006=LINE ( 'NONE', #36251, #13747 ) ;
#9017=AXIS2_PLACEMENT_3D ( 'NONE', #26749, #89901, #55334 ) ;
#9019=CARTESIAN_POINT ( 'NONE',  ( 70.56670390244700286, -67.87844715994098976, 55.21780685541800437 ) ) ;
#9021=AXIS2_PLACEMENT_3D ( 'NONE', #24719, #65606, #12780 ) ;
#9044=DIRECTION ( 'NONE',  ( 1.000000000000000000, 1.000000000000000078E-15, -0.000000000000000000 ) ) ;
#9063=ORIENTED_EDGE ( 'NONE', *, *, #61454, .T. ) ;
#9075=EDGE_LOOP ( 'NONE', ( #73691, #80111, #44227, #16782, #27296 ) ) ;
#9089=VECTOR ( 'NONE', #89726, 1000.000000000000000 ) ;
#9096=VERTEX_POINT ( 'NONE', #5224 ) ;
#9101=EDGE_CURVE ( 'NONE', #28081, #17066, #88357, .T. ) ;
#9108=CARTESIAN_POINT ( 'NONE',  ( 68.06670390244705970, -121.7784471599409954, 55.21780685541800437 ) ) ;
#9127=VERTEX_POINT ( 'NONE', #81988 ) ;
#9137=CARTESIAN_POINT ( 'NONE',  ( 107.0667039024470313, -104.2784471599421323, -21.78219314458201694 ) ) ;
#9143=CARTESIAN_POINT ( 'NONE',  ( 67.06670390244700286, -67.87844716047356997, 245.4920193514540188 ) ) ;
#9161=CARTESIAN_POINT ( 'NONE',  ( 102.3035641816324102, -89.52844715994213232, -21.78219314458246103 ) ) ;
#9167=CARTESIAN_POINT ( 'NONE',  ( 143.0667039024470171, -90.27844715994091018, 222.2178068554179902 ) ) ;
#9169=EDGE_LOOP ( 'NONE', ( #51584, #84923, #18907, #86107 ) ) ;
#9176=ORIENTED_EDGE ( 'NONE', *, *, #36504, .F. ) ;
#9186=DIRECTION ( 'NONE',  ( 0.3535533905932722321, 0.6123724356958172299, 0.7071067811865286989 ) ) ;
#9191=EDGE_CURVE ( 'NONE', #81699, #76096, #56487, .T. ) ;
#9196=VERTEX_POINT ( 'NONE', #34708 ) ;
#9204=ADVANCED_FACE ( 'NONE', ( #1991 ), #52818, .T. ) ;
#9214=CARTESIAN_POINT ( 'NONE',  ( 70.21108942365968630, -140.4774569966043885, 246.4394912367985739 ) ) ;
#9217=ORIENTED_EDGE ( 'NONE', *, *, #61350, .T. ) ;
#9224=CARTESIAN_POINT ( 'NONE',  ( 69.30126767323736203, -138.7022917610363777, 247.3064795105084102 ) ) ;
#9226=CARTESIAN_POINT ( 'NONE',  ( 135.5667039024470455, -118.2784471599408960, 51.21780685541800437 ) ) ;
#9229=FACE_BOUND ( 'NONE', #1303, .T. ) ;
#9265=CARTESIAN_POINT ( 'NONE',  ( 132.2857443282839824, -83.77844715994092439, 45.21780685541799727 ) ) ;
#9271=VERTEX_POINT ( 'NONE', #78760 ) ;
#9292=VERTEX_POINT ( 'NONE', #31024 ) ;
#9296=EDGE_CURVE ( 'NONE', #57531, #81381, #37507, .T. ) ;
#9309=EDGE_CURVE ( 'NONE', #25396, #42066, #79202, .T. ) ;
#9319=EDGE_CURVE ( 'NONE', #11706, #33876, #76083, .T. ) ;
#9330=DIRECTION ( 'NONE',  ( -1.000000000000000078E-15, 1.000000000000000000, 0.000000000000000000 ) ) ;
#9347=DIRECTION ( 'NONE',  ( 1.000000000000000000, 0.000000000000000000, 0.000000000000000000 ) ) ;
#9350=VECTOR ( 'NONE', #62960, 1000.000000000000000 ) ;
#9365=ORIENTED_EDGE ( 'NONE', *, *, #68567, .F. ) ;
#9367=EDGE_CURVE ( 'NONE', #61103, #84281, #56897, .T. ) ;
#9384=CARTESIAN_POINT ( 'NONE',  ( 82.78637150392549415, -117.3006669637344714, 250.2178068554180470 ) ) ;
#9401=PLANE ( 'NONE',  #48807 ) ;
#9403=ORIENTED_EDGE ( 'NONE', *, *, #86345, .F. ) ;
#9412=CARTESIAN_POINT ( 'NONE',  ( 107.0667039024470313, -104.2784471599409528, 23.21780685541800082 ) ) ;
#9444=EDGE_LOOP ( 'NONE', ( #4222, #7504, #36954, #60326, #3909 ) ) ;
#9461=PLANE ( 'NONE',  #83227 ) ;
#9486=VECTOR ( 'NONE', #87349, 1000.000000000000000 ) ;
#9500=EDGE_CURVE ( 'NONE', #65538, #9127, #82330, .T. ) ;
#9513=CARTESIAN_POINT ( 'NONE',  ( 68.56670390244707392, -139.1784471599409869, 228.4678068554179902 ) ) ;
#9526=CARTESIAN_POINT ( 'NONE',  ( 142.6617037637538772, -139.6113389983086108, 247.4111996305669834 ) ) ;
#9535=EDGE_LOOP ( 'NONE', ( #63387, #29373 ) ) ;
#9543=DIRECTION ( 'NONE',  ( 1.075267683398002218E-15, -1.000000000000000000, 3.100000000000000044E-14 ) ) ;
#9551=ORIENTED_EDGE ( 'NONE', *, *, #58496, .T. ) ;
#9608=FACE_OUTER_BOUND ( 'NONE', #50137, .T. ) ;
#9614=EDGE_LOOP ( 'NONE', ( #23057, #72319, #10441, #33365 ) ) ;
#9618=DIRECTION ( 'NONE',  ( 1.000000000000000000, 1.000000000000000078E-15, 0.000000000000000000 ) ) ;
#9621=ORIENTED_EDGE ( 'NONE', *, *, #3984, .F. ) ;
#9636=( BOUNDED_CURVE ( )  B_SPLINE_CURVE ( 3, ( #80555, #18311, #40091, #17867 ),
 .UNSPECIFIED., .F., .T. ) 
 B_SPLINE_CURVE_WITH_KNOTS ( ( 4, 4 ),
 ( 5.813027347256380040, 6.753343267102792424 ),
 .UNSPECIFIED. ) 
 CURVE ( )  GEOMETRIC_REPRESENTATION_ITEM ( )  RATIONAL_B_SPLINE_CURVE ( ( 1.000000000000000000, 0.9276644927932374829, 0.9276644927932374829, 1.000000000000000000 ) ) 
 REPRESENTATION_ITEM ( '' )  );
#9638=ORIENTED_EDGE ( 'NONE', *, *, #60540, .T. ) ;
#9677=EDGE_CURVE ( 'NONE', #15221, #62972, #21887, .T. ) ;
#9685=CARTESIAN_POINT ( 'NONE',  ( 161.0667039024469886, -67.87844715994089029, 96.96780685541800437 ) ) ;
#9691=CARTESIAN_POINT ( 'NONE',  ( 106.5667039024470455, -113.2645475377471058, 2.217806855418280598 ) ) ;
#9720=CARTESIAN_POINT ( 'NONE',  ( 111.8591559558596060, -71.06560796536048485, 248.4067532124560103 ) ) ;
#9721=CARTESIAN_POINT ( 'NONE',  ( 146.9828512772299121, -67.95600236836138208, 246.0626215148325286 ) ) ;
#9770=CARTESIAN_POINT ( 'NONE',  ( 107.0667039024470313, -104.2784471599409528, 23.21780685541800082 ) ) ;
#9772=CARTESIAN_POINT ( 'NONE',  ( 143.5715564487395852, -139.7453820604759187, 247.2256998566546713 ) ) ;
#9778=DIRECTION ( 'NONE',  ( 0.000000000000000000, 0.000000000000000000, 1.000000000000000000 ) ) ;
#9781=CARTESIAN_POINT ( 'NONE',  ( 70.06670390441306040, -140.6784471619069734, 245.4415720117440003 ) ) ;
#9794=ORIENTED_EDGE ( 'NONE', *, *, #39227, .F. ) ;
#9807=DIRECTION ( 'NONE',  ( 0.000000000000000000, 0.000000000000000000, 1.000000000000000000 ) ) ;
#9808=EDGE_CURVE ( 'NONE', #69984, #86558, #30919, .T. ) ;
#9831=ORIENTED_EDGE ( 'NONE', *, *, #36375, .F. ) ;
#9856=ORIENTED_EDGE ( 'NONE', *, *, #30132, .T. ) ;
#9863=CARTESIAN_POINT ( 'NONE',  ( 52.06670390244700997, -79.67844715994100113, 55.21780685541800437 ) ) ;
#9872=EDGE_LOOP ( 'NONE', ( #22194, #88936 ) ) ;
#9883=DIRECTION ( 'NONE',  ( -1.000000000000000000, -1.206764157201257538E-15, 0.000000000000000000 ) ) ;
#9900=VECTOR ( 'NONE', #33881, 1000.000000000000000 ) ;
#9903=CARTESIAN_POINT ( 'NONE',  ( 107.0667039024470313, -104.2784471599413791, 2.217806855418003043 ) ) ;
#9927=EDGE_CURVE ( 'NONE', #9271, #35871, #2185, .T. ) ;
#9941=CIRCLE ( 'NONE', #43242, 2.999999999999975131 ) ;
#9960=CARTESIAN_POINT ( 'NONE',  ( 112.7920658800750005, -68.84166263841879640, 247.5834178368470191 ) ) ;
#9965=VERTEX_POINT ( 'NONE', #32246 ) ;
#9975=CARTESIAN_POINT ( 'NONE',  ( 144.7505022533608496, -139.5561530133492170, 246.9828090814930022 ) ) ;
#9976=CARTESIAN_POINT ( 'NONE',  ( 123.4403675665762989, -109.5826158781450914, -10.56397404668061135 ) ) ;
#9983=EDGE_CURVE ( 'NONE', #84959, #7062, #13479, .T. ) ;
#10001=EDGE_LOOP ( 'NONE', ( #13076, #16866, #26174, #40502 ) ) ;
#10015=CARTESIAN_POINT ( 'NONE',  ( 137.0667039024470171, -90.27844715994091018, 51.21780685541800437 ) ) ;
#10017=EDGE_CURVE ( 'NONE', #5965, #20346, #28194, .T. ) ;
#10028=DIRECTION ( 'NONE',  ( 3.100000000000000258E-29, -3.100000000000000044E-14, -1.000000000000000000 ) ) ;
#10035=CARTESIAN_POINT ( 'NONE',  ( 67.06673837846007302, -137.6758525980020806, 245.5072637273240161 ) ) ;
#10044=ORIENTED_EDGE ( 'NONE', *, *, #81496, .F. ) ;
#10063=CARTESIAN_POINT ( 'NONE',  ( 131.2274048610838406, -69.45962296279897430, 247.5830566269779922 ) ) ;
#10064=ADVANCED_FACE ( 'NONE', ( #43879 ), #1679, .T. ) ;
#10071=CARTESIAN_POINT ( 'NONE',  ( 59.56670390244699576, -67.87844715994098976, 85.21780685541799016 ) ) ;
#10072=EDGE_CURVE ( 'NONE', #12139, #34789, #46750, .T. ) ;
#10087=ORIENTED_EDGE ( 'NONE', *, *, #81401, .T. ) ;
#10101=VERTEX_POINT ( 'NONE', #21676 ) ;
#10111=CARTESIAN_POINT ( 'NONE',  ( 68.95691901195219486, -139.0437307363913817, 246.8274569434534840 ) ) ;
#10136=CARTESIAN_POINT ( 'NONE',  ( 144.0667052733537901, -75.82844715994092155, 55.21780685541800437 ) ) ;
#10140=EDGE_CURVE ( 'NONE', #30286, #53126, #2122, .T. ) ;
#10155=FACE_OUTER_BOUND ( 'NONE', #73262, .T. ) ;
#10156=CIRCLE ( 'NONE', #82733, 17.00000000000000000 ) ;
#10164=FACE_OUTER_BOUND ( 'NONE', #78384, .T. ) ;
#10165=CARTESIAN_POINT ( 'NONE',  ( 146.3552114757505080, -68.56422815332481946, 247.0266215615655767 ) ) ;
#10213=DIRECTION ( 'NONE',  ( -1.000000000000000000, -1.206764157201257538E-15, 0.000000000000000000 ) ) ;
#10214=CARTESIAN_POINT ( 'NONE',  ( 143.7067540604739690, -140.0404100990022584, 247.0021857859347847 ) ) ;
#10236=PLANE ( 'NONE',  #42665 ) ;
#10244=LINE ( 'NONE', #4327, #77795 ) ;
#10258=ORIENTED_EDGE ( 'NONE', *, *, #55698, .T. ) ;
#10261=CARTESIAN_POINT ( 'NONE',  ( 116.3167039024470029, -68.87844715994093292, 55.21780685541800437 ) ) ;
#10277=CARTESIAN_POINT ( 'NONE',  ( 121.2221484686747459, -113.6057974291316839, -19.26696060647573105 ) ) ;
#10289=CARTESIAN_POINT ( 'NONE',  ( 85.06670390244700286, -71.37844715994096134, 55.21780685541800437 ) ) ;
#10293=EDGE_LOOP ( 'NONE', ( #78266, #51391, #72287, #47534 ) ) ;
#10302=CARTESIAN_POINT ( 'NONE',  ( 144.0637245237351749, -140.6784087391956746, 245.5331728883010101 ) ) ;
#10309=CIRCLE ( 'NONE', #52349, 4.500000000000003553 ) ;
#10329=ORIENTED_EDGE ( 'NONE', *, *, #51143, .T. ) ;
#10332=DIRECTION ( 'NONE',  ( -0.000000000000000000, -0.000000000000000000, -1.000000000000000000 ) ) ;
#10335=ADVANCED_FACE ( 'NONE', ( #86134 ), #23909, .F. ) ;
#10342=DIRECTION ( 'NONE',  ( -0.8660254037844382635, -0.5000000000000008882, 1.550000000000000022E-14 ) ) ;
#10345=FACE_OUTER_BOUND ( 'NONE', #86076, .T. ) ;
#10348=EDGE_LOOP ( 'NONE', ( #5840, #60301, #8959, #32910, #3193 ) ) ;
#10353=DIRECTION ( 'NONE',  ( 1.000000000000000000, 1.000000000000000078E-15, 0.000000000000000000 ) ) ;
#10370=CARTESIAN_POINT ( 'NONE',  ( 99.08946256649485917, -109.4614598618336174, 2.217806855418169576 ) ) ;
#10374=ORIENTED_EDGE ( 'NONE', *, *, #33623, .F. ) ;
#10396=DIRECTION ( 'NONE',  ( 0.000000000000000000, 0.000000000000000000, -1.000000000000000000 ) ) ;
#10413=CARTESIAN_POINT ( 'NONE',  ( 131.8286686973700910, -67.87844715994091871, 245.6137563491429887 ) ) ;
#10429=EDGE_CURVE ( 'NONE', #43983, #18666, #20660, .T. ) ;
#10441=ORIENTED_EDGE ( 'NONE', *, *, #73968, .T. ) ;
#10449=AXIS2_PLACEMENT_3D ( 'NONE', #34682, #41486, #29669 ) ;
#10462=CARTESIAN_POINT ( 'NONE',  ( 115.0439452383991892, -99.09543445804915507, 2.217806855417836509 ) ) ;
#10465=VECTOR ( 'NONE', #79350, 1000.000000000000000 ) ;
#10470=ORIENTED_EDGE ( 'NONE', *, *, #36676, .T. ) ;
#10478=EDGE_LOOP ( 'NONE', ( #9551, #35108, #63456, #33435 ) ) ;
#10492=DIRECTION ( 'NONE',  ( -0.4999999999999985567, -0.8660254037844395958, 2.602085213965200860E-14 ) ) ;
#10504=DIRECTION ( 'NONE',  ( 0.000000000000000000, 0.000000000000000000, -1.000000000000000000 ) ) ;
#10505=EDGE_LOOP ( 'NONE', ( #77700, #79668, #86686, #34967 ) ) ;
#10562=ADVANCED_FACE ( 'NONE', ( #68362 ), #89259, .T. ) ;
#10585=ADVANCED_FACE ( 'NONE', ( #63789 ), #22909, .F. ) ;
#10591=LINE ( 'NONE', #3786, #17637 ) ;
#10603=DIRECTION ( 'NONE',  ( -1.000000000000000000, -1.734723475976808672E-15, 0.000000000000000000 ) ) ;
#10612=B_SPLINE_CURVE_WITH_KNOTS ( 'NONE', 3,
 ( #44819, #23950, #52499, #86175, #80263 ),
 .UNSPECIFIED., .F., .F.,
 ( 4, 1, 4 ),
 ( 0.1438945294004070063, 4.132355267033809731, 7.123703416098150498 ),
 .UNSPECIFIED. ) ;
#10620=EDGE_CURVE ( 'NONE', #61315, #86385, #56163, .T. ) ;
#10640=ORIENTED_EDGE ( 'NONE', *, *, #24101, .F. ) ;
#10648=CARTESIAN_POINT ( 'NONE',  ( 143.6231792275268617, -139.8594620027156736, 247.1482994587078394 ) ) ;
#10661=CARTESIAN_POINT ( 'NONE',  ( 107.0667039024470313, -104.2784471599421323, -21.78219314458201694 ) ) ;
#10667=CARTESIAN_POINT ( 'NONE',  ( 103.8797721312301405, -101.8611209747514010, -19.78219314458209865 ) ) ;
#10672=VECTOR ( 'NONE', #17000, 1000.000000000000000 ) ;
#10686=ORIENTED_EDGE ( 'NONE', *, *, #66208, .F. ) ;
#10693=VECTOR ( 'NONE', #82168, 1000.000000000000000 ) ;
#10699=LINE ( 'NONE', #1783, #48684 ) ;
#10725=ORIENTED_EDGE ( 'NONE', *, *, #26800, .F. ) ;
#10727=ORIENTED_EDGE ( 'NONE', *, *, #56375, .T. ) ;
#10733=ADVANCED_FACE ( 'NONE', ( #42867 ), #77868, .F. ) ;
#10745=ORIENTED_EDGE ( 'NONE', *, *, #16731, .F. ) ;
#10772=PLANE ( 'NONE',  #79949 ) ;
#10773=ORIENTED_EDGE ( 'NONE', *, *, #39623, .F. ) ;
#10807=EDGE_CURVE ( 'NONE', #75812, #80812, #81454, .T. ) ;
#10813=VECTOR ( 'NONE', #83878, 1000.000000000000000 ) ;
#10833=CARTESIAN_POINT ( 'NONE',  ( 147.0761462423337775, -68.28389950123539620, 246.9923701901030029 ) ) ;
#10838=AXIS2_PLACEMENT_3D ( 'NONE', #82700, #54489, #67247 ) ;
#10861=CARTESIAN_POINT ( 'NONE',  ( 90.06670390244703128, -104.2784471599417770, -9.937637710810031777 ) ) ;
#10896=CARTESIAN_POINT ( 'NONE',  ( 140.0667039024470171, -90.27844715994091018, 45.21780685541799727 ) ) ;
#10900=CARTESIAN_POINT ( 'NONE',  ( 120.2221484686747317, -96.68314769832106492, -11.78219314458223188 ) ) ;
#10917=VECTOR ( 'NONE', #20418, 1000.000000000000000 ) ;
#10978=EDGE_CURVE ( 'NONE', #6676, #53380, #28238, .T. ) ;
#10991=AXIS2_PLACEMENT_3D ( 'NONE', #57252, #15946, #78639 ) ;
#10998=CARTESIAN_POINT ( 'NONE',  ( 145.4469796106781416, -124.3929973698032114, 247.5412109164290086 ) ) ;
#11005=AXIS2_PLACEMENT_3D ( 'NONE', #33413, #73849, #11636 ) ;
#11050=CARTESIAN_POINT ( 'NONE',  ( 117.9332873271178102, -93.05227202534730679, -21.78219314458237932 ) ) ;
#11051=VERTEX_POINT ( 'NONE', #9161 ) ;
#11057=EDGE_LOOP ( 'NONE', ( #61723, #24419, #34680, #36827 ) ) ;
#11066=DIRECTION ( 'NONE',  ( -0.08901729878539284269, 0.06045726171402947963, 0.9941935626541712478 ) ) ;
#11071=VERTEX_POINT ( 'NONE', #24128 ) ;
#11087=CIRCLE ( 'NONE', #18348, 17.00000000000000000 ) ;
#11096=CARTESIAN_POINT ( 'NONE',  ( 106.1656040943334318, -87.30234574837481887, -21.78219314458254630 ) ) ;
#11102=CARTESIAN_POINT ( 'NONE',  ( 67.63716323619298976, -137.3564796873130263, 246.9094381074559408 ) ) ;
#11106=ORIENTED_EDGE ( 'NONE', *, *, #83522, .F. ) ;
#11141=DIRECTION ( 'NONE',  ( -3.100000000000000258E-29, 3.100000000000000044E-14, 1.000000000000000000 ) ) ;
#11151=CYLINDRICAL_SURFACE ( 'NONE', #18351, 24.50000000000000711 ) ;
#11159=CARTESIAN_POINT ( 'NONE',  ( 99.03451269431033666, -100.2184096729307470, 2.217806855417864043 ) ) ;
#11188=ORIENTED_EDGE ( 'NONE', *, *, #25908, .T. ) ;
#11192=CARTESIAN_POINT ( 'NONE',  ( 147.0667039024469886, -67.87844715994090450, 222.2178068554179902 ) ) ;
#11201=DIRECTION ( 'NONE',  ( 1.000000000000000078E-15, -1.000000000000000000, 0.000000000000000000 ) ) ;
#11213=LINE ( 'NONE', #52079, #61641 ) ;
#11214=CARTESIAN_POINT ( 'NONE',  ( 143.0667039024470455, -124.7784471599409102, 55.21780685541800437 ) ) ;
#11219=DIRECTION ( 'NONE',  ( -3.100000000000000258E-29, 3.100000000000000044E-14, 1.000000000000000000 ) ) ;
#11237=CARTESIAN_POINT ( 'NONE',  ( 144.0665648704335808, -140.6784485900456900, 245.9352930260599805 ) ) ;
#11245=ORIENTED_EDGE ( 'NONE', *, *, #20264, .T. ) ;
#11247=ORIENTED_EDGE ( 'NONE', *, *, #9808, .F. ) ;
#11251=CARTESIAN_POINT ( 'NONE',  ( 69.56670390244701707, -90.27844715994098124, 51.21780685541800437 ) ) ;
#11289=ORIENTED_EDGE ( 'NONE', *, *, #17583, .F. ) ;
#11293=ORIENTED_EDGE ( 'NONE', *, *, #1714, .T. ) ;
#11302=AXIS2_PLACEMENT_3D ( 'NONE', #7699, #7258, #27693 ) ;
#11308=ADVANCED_FACE ( 'NONE', ( #39076 ), #5468, .T. ) ;
#11311=CARTESIAN_POINT ( 'NONE',  ( 107.0667039024470313, -104.2784471599413934, 2.217806855418003043 ) ) ;
#11313=CARTESIAN_POINT ( 'NONE',  ( 121.2221484686747317, -94.95109689075241022, -19.26696060647628528 ) ) ;
#11319=VERTEX_POINT ( 'NONE', #60406 ) ;
#11360=ORIENTED_EDGE ( 'NONE', *, *, #63686, .T. ) ;
#11377=B_SPLINE_CURVE_WITH_KNOTS ( 'NONE', 3,
 ( #9143, #31353, #43186, #22778, #10035 ),
 .UNSPECIFIED., .F., .F.,
 ( 4, 1, 4 ),
 ( -7.123703416098150498, -3.135239217345689777, -0.1438962376298542623 ),
 .UNSPECIFIED. ) ;
#11385=FACE_OUTER_BOUND ( 'NONE', #8759, .T. ) ;
#11386=CARTESIAN_POINT ( 'NONE',  ( 121.2221484686747317, -94.95109689075249548, -21.78219314458229405 ) ) ;
#11387=EDGE_LOOP ( 'NONE', ( #29293, #32623, #67846, #60044, #23685, #87514 ) ) ;
#11403=VERTEX_POINT ( 'NONE', #28125 ) ;
#11416=ORIENTED_EDGE ( 'NONE', *, *, #39381, .F. ) ;
#11422=ORIENTED_EDGE ( 'NONE', *, *, #62805, .F. ) ;
#11429=CARTESIAN_POINT ( 'NONE',  ( 80.15209520963914258, -113.0957571362959726, 250.2190963482990185 ) ) ;
#11450=ADVANCED_FACE ( 'NONE', ( #84016 ), #69932, .F. ) ;
#11452=CARTESIAN_POINT ( 'NONE',  ( 140.0667039024470455, -118.2784471599408960, 45.21780685541799727 ) ) ;
#11454=DIRECTION ( 'NONE',  ( 0.000000000000000000, 0.000000000000000000, -1.000000000000000000 ) ) ;
#11458=EDGE_CURVE ( 'NONE', #31568, #60190, #57731, .T. ) ;
#11459=CARTESIAN_POINT ( 'NONE',  ( 147.0667039024469886, -67.87574355753805833, 246.0361703021810058 ) ) ;
#11476=DIRECTION ( 'NONE',  ( 3.100000000000000258E-29, -3.100000000000000044E-14, -1.000000000000000000 ) ) ;
#11490=LINE ( 'NONE', #75510, #38517 ) ;
#11503=VERTEX_POINT ( 'NONE', #87138 ) ;
#11506=VECTOR ( 'NONE', #50545, 1000.000000000000000 ) ;
#11533=VERTEX_POINT ( 'NONE', #59405 ) ;
#11548=ORIENTED_EDGE ( 'NONE', *, *, #32031, .T. ) ;
#11586=CARTESIAN_POINT ( 'NONE',  ( 104.0667030381796963, -67.87844715994094713, 93.21780742166239975 ) ) ;
#11605=ORIENTED_EDGE ( 'NONE', *, *, #61383, .F. ) ;
#11612=VECTOR ( 'NONE', #36961, 1000.000000000000000 ) ;
#11614=DIRECTION ( 'NONE',  ( 1.000000000000000000, 0.000000000000000000, 0.000000000000000000 ) ) ;
#11620=DIRECTION ( 'NONE',  ( 0.000000000000000000, 0.000000000000000000, -1.000000000000000000 ) ) ;
#11624=VECTOR ( 'NONE', #64177, 1000.000000000000000 ) ;
#11625=EDGE_CURVE ( 'NONE', #68999, #70410, #86692, .T. ) ;
#11632=DIRECTION ( 'NONE',  ( -3.100000000000000258E-29, 3.100000000000000044E-14, 1.000000000000000000 ) ) ;
#11636=DIRECTION ( 'NONE',  ( -1.000000000000000000, -1.734723475976808672E-15, 0.000000000000000000 ) ) ;
#11640=ORIENTED_EDGE ( 'NONE', *, *, #4463, .F. ) ;
#11649=CARTESIAN_POINT ( 'NONE',  ( 90.69304023831777783, -98.97427844173844846, -10.56397404668094353 ) ) ;
#11668=CARTESIAN_POINT ( 'NONE',  ( 111.8298436232616240, -119.0284471599421181, -21.78219314458157285 ) ) ;
#11692=AXIS2_PLACEMENT_3D ( 'NONE', #88653, #2303, #28646 ) ;
#11700=CARTESIAN_POINT ( 'NONE',  ( 87.66417971789877583, -139.1778880632977575, 247.6203581219589864 ) ) ;
#11702=CARTESIAN_POINT ( 'NONE',  ( 69.05801668363947954, -139.6697599411332931, 245.6076672521240027 ) ) ;
#11706=VERTEX_POINT ( 'NONE', #53466 ) ;
#11719=ORIENTED_EDGE ( 'NONE', *, *, #34908, .T. ) ;
#11739=CARTESIAN_POINT ( 'NONE',  ( 89.92341034714860371, -67.87844715994096134, 245.7176246637040151 ) ) ;
#11760=ORIENTED_EDGE ( 'NONE', *, *, #75430, .T. ) ;
#11768=CARTESIAN_POINT ( 'NONE',  ( 53.06670390244699576, -67.87844715994100397, 222.2178068554179902 ) ) ;
#11800=VERTEX_POINT ( 'NONE', #80778 ) ;
#11808=PLANE ( 'NONE',  #37805 ) ;
#11813=EDGE_CURVE ( 'NONE', #59337, #80549, #51934, .T. ) ;
#11820=CARTESIAN_POINT ( 'NONE',  ( 69.95483947742927455, -138.0502943369556021, 247.6584922829669893 ) ) ;
#11859=B_SPLINE_CURVE_WITH_KNOTS ( 'NONE', 3,
 ( #4092, #2772, #72251, #36832, #30466, #58165 ),
 .UNSPECIFIED., .F., .F.,
 ( 4, 2, 4 ),
 ( -0.008545295454838610846, -0.004274282335290478449, 0.000000000000000000 ),
 .UNSPECIFIED. ) ;
#11860=VERTEX_POINT ( 'NONE', #35740 ) ;
#11863=FACE_OUTER_BOUND ( 'NONE', #31505, .T. ) ;
#11881=DIRECTION ( 'NONE',  ( 1.000000000000000078E-15, -1.000000000000000000, 0.000000000000000000 ) ) ;
#11892=DIRECTION ( 'NONE',  ( -1.000000000000000078E-15, 1.000000000000000000, 0.000000000000000000 ) ) ;
#11896=FACE_OUTER_BOUND ( 'NONE', #87984, .T. ) ;
#11897=FACE_OUTER_BOUND ( 'NONE', #9444, .T. ) ;
#11908=DIRECTION ( 'NONE',  ( 0.7071067811865453523, 0.7071067811865496822, 0.000000000000000000 ) ) ;
#11909=ORIENTED_EDGE ( 'NONE', *, *, #18263, .F. ) ;
#11945=AXIS2_PLACEMENT_3D ( 'NONE', #82521, #20283, #82963 ) ;
#11955=ADVANCED_FACE ( 'NONE', ( #35285 ), #15318, .F. ) ;
#11956=ADVANCED_FACE ( 'NONE', ( #68927 ), #14875, .T. ) ;
#11987=CARTESIAN_POINT ( 'NONE',  ( 56.06670390244700997, -79.67844715994098692, 155.2178068554179902 ) ) ;
#11993=CARTESIAN_POINT ( 'NONE',  ( 90.06670420047024095, -102.7784471599409670, 222.2178068554179902 ) ) ;
#12012=DIRECTION ( 'NONE',  ( -0.8660254037844377084, -0.5000000000000016653, 1.550000000000002231E-14 ) ) ;
#12016=LINE ( 'NONE', #86981, #86588 ) ;
#12020=FACE_OUTER_BOUND ( 'NONE', #40734, .T. ) ;
#12033=CARTESIAN_POINT ( 'NONE',  ( 107.0667039024470313, -104.2784471599409528, 250.2178068554179902 ) ) ;
#12058=ORIENTED_EDGE ( 'NONE', *, *, #49569, .F. ) ;
#12062=CARTESIAN_POINT ( 'NONE',  ( 107.0667039024470313, -104.2784471599409528, 19.21780685541800437 ) ) ;
#12063=DIRECTION ( 'NONE',  ( -1.000000000000000000, -8.163404592832032979E-16, 0.000000000000000000 ) ) ;
#12103=AXIS2_PLACEMENT_3D ( 'NONE', #66692, #10396, #87594 ) ;
#12115=ORIENTED_EDGE ( 'NONE', *, *, #55593, .T. ) ;
#12117=LINE ( 'NONE', #3075, #32597 ) ;
#12132=ORIENTED_EDGE ( 'NONE', *, *, #24995, .T. ) ;
#12134=ADVANCED_FACE ( 'NONE', ( #53702 ), #83247, .T. ) ;
#12139=VERTEX_POINT ( 'NONE', #26035 ) ;
#12144=CARTESIAN_POINT ( 'NONE',  ( 144.5610809520308351, -138.4343374614282425, 247.5945153064158717 ) ) ;
#12148=EDGE_LOOP ( 'NONE', ( #34251, #50136, #46001, #47466 ) ) ;
#12150=ORIENTED_EDGE ( 'NONE', *, *, #9808, .T. ) ;
#12153=AXIS2_PLACEMENT_3D ( 'NONE', #7229, #77168, #62629 ) ;
#12180=ORIENTED_EDGE ( 'NONE', *, *, #41968, .T. ) ;
#12196=ORIENTED_EDGE ( 'NONE', *, *, #23708, .T. ) ;
#12197=CARTESIAN_POINT ( 'NONE',  ( 162.0667039024470171, -77.67844715994088745, 96.96780685541800437 ) ) ;
#12202=CARTESIAN_POINT ( 'NONE',  ( 127.4058501689330996, -85.76982405743852667, 250.2178068554179902 ) ) ;
#12244=EDGE_LOOP ( 'NONE', ( #20031, #5929, #3263, #39852, #25252, #6395 ) ) ;
#12245=DIRECTION ( 'NONE',  ( -0.000000000000000000, -0.000000000000000000, 1.000000000000000000 ) ) ;
#12254=AXIS2_PLACEMENT_3D ( 'NONE', #85320, #2636, #49410 ) ;
#12269=ORIENTED_EDGE ( 'NONE', *, *, #8100, .T. ) ;
#12275=VECTOR ( 'NONE', #6333, 1000.000000000000000 ) ;
#12278=DIRECTION ( 'NONE',  ( 0.5000000000000015543, -0.8660254037844377084, 2.602085213965216006E-14 ) ) ;
#12283=CARTESIAN_POINT ( 'NONE',  ( 85.06670390244701707, -80.35669973212957018, 222.2178068554179902 ) ) ;
#12292=CARTESIAN_POINT ( 'NONE',  ( 85.06670390244700286, -74.11757344603526576, 55.21780685541800437 ) ) ;
#12304=ORIENTED_EDGE ( 'NONE', *, *, #37775, .F. ) ;
#12318=AXIS2_PLACEMENT_3D ( 'NONE', #53321, #81086, #19290 ) ;
#12322=DIRECTION ( 'NONE',  ( 1.000000000000000078E-15, -1.000000000000000000, 0.000000000000000000 ) ) ;
#12354=ADVANCED_FACE ( 'NONE', ( #41871 ), #70506, .T. ) ;
#12363=CARTESIAN_POINT ( 'NONE',  ( 139.8778540137985829, -131.0224759750418286, 248.3919668373590071 ) ) ;
#12367=ORIENTED_EDGE ( 'NONE', *, *, #69463, .F. ) ;
#12375=LINE ( 'NONE', #40065, #42784 ) ;
#12379=AXIS2_PLACEMENT_3D ( 'NONE', #5059, #39568, #32757 ) ;
#12426=DIRECTION ( 'NONE',  ( 0.000000000000000000, 0.000000000000000000, -1.000000000000000000 ) ) ;
#12433=CARTESIAN_POINT ( 'NONE',  ( 146.0667039024470171, -94.02844715994091018, 55.21780685541800437 ) ) ;
#12454=DIRECTION ( 'NONE',  ( -3.100000000000000258E-29, 3.100000000000000044E-14, 1.000000000000000000 ) ) ;
#12462=EDGE_LOOP ( 'NONE', ( #37127, #40691, #85433, #10745 ) ) ;
#12477=AXIS2_PLACEMENT_3D ( 'NONE', #16417, #64121, #37301 ) ;
#12479=EDGE_CURVE ( 'NONE', #76165, #41047, #76143, .T. ) ;
#12491=LINE ( 'NONE', #66995, #30907 ) ;
#12529=EDGE_LOOP ( 'NONE', ( #716, #23097, #41804 ) ) ;
#12541=B_SPLINE_SURFACE_WITH_KNOTS ( 'NONE', 3, 3, ( 
 ( #61617, #13047, #66648, #11700, #38942, #61177 ),
 ( #4437, #88905, #67099, #4880, #26657, #54337 ),
 ( #82103, #19851, #60271, #81205, #88002, #47537 ),
 ( #11237, #45732, #75270, #68454, #89353, #80305 ),
 ( #18054, #73460, #32124, #59821, #52982, #8016 ) ),
 .UNSPECIFIED., .F., .F., .F.,
 ( 4, 1, 4 ),
 ( 4, 1, 1, 4 ),
 ( -2.453700414991130114E-06, 0.5714285714285709528, 1.000002453700419958 ),
 ( 0.1139507740808489988, 4.342301322120899698, 5.399388959130909882, 7.513564233150940019 ),
 .UNSPECIFIED. ) ;
#12543=PLANE ( 'NONE',  #63480 ) ;
#12561=EDGE_CURVE ( 'NONE', #15404, #21921, #38209, .T. ) ;
#12565=DIRECTION ( 'NONE',  ( 1.000000000000000000, 0.000000000000000000, 0.000000000000000000 ) ) ;
#12568=CARTESIAN_POINT ( 'NONE',  ( 59.56670390244699576, -67.87844715994098976, 155.2178068554179902 ) ) ;
#12586=ORIENTED_EDGE ( 'NONE', *, *, #63026, .T. ) ;
#12596=CARTESIAN_POINT ( 'NONE',  ( 145.1753220238131519, -139.0425770237959284, 246.8297448300953079 ) ) ;
#12598=CARTESIAN_POINT ( 'NONE',  ( 68.87339889186067410, -139.0446803891145748, 247.0600586179500056 ) ) ;
#12619=ADVANCED_FACE ( 'NONE', ( #69049 ), #18660, .F. ) ;
#12638=VECTOR ( 'NONE', #7421, 1000.000000000000000 ) ;
#12639=CARTESIAN_POINT ( 'NONE',  ( 115.5439452383991892, -99.96145986183427112, -19.78219314458215550 ) ) ;
#12646=CARTESIAN_POINT ( 'NONE',  ( 103.8797721312301405, -101.8611209747507189, 2.217806855417919998 ) ) ;
#12693=DIRECTION ( 'NONE',  ( -1.000000000000000000, -8.163404592832032979E-16, 0.000000000000000000 ) ) ;
#12699=CARTESIAN_POINT ( 'NONE',  ( 88.79221564186276794, -137.6784471599409585, 55.21780685541800437 ) ) ;
#12704=DIRECTION ( 'NONE',  ( -3.100000000000000258E-29, 3.100000000000000044E-14, 1.000000000000000000 ) ) ;
#12708=CARTESIAN_POINT ( 'NONE',  ( 153.0667039024470739, -124.7784471599408960, 222.2178068554179902 ) ) ;
#12712=LINE ( 'NONE', #71269, #38395 ) ;
#12716=ORIENTED_EDGE ( 'NONE', *, *, #18622, .T. ) ;
#12728=AXIS2_PLACEMENT_3D ( 'NONE', #77167, #14944, #42613 ) ;
#12736=CIRCLE ( 'NONE', #83810, 3.000000000000002665 ) ;
#12747=VECTOR ( 'NONE', #15978, 1000.000000000000000 ) ;
#12780=DIRECTION ( 'NONE',  ( -1.000000000000000000, -1.206764157201257538E-15, 0.000000000000000000 ) ) ;
#12782=EDGE_CURVE ( 'NONE', #51228, #27673, #54272, .T. ) ;
#12791=DIRECTION ( 'NONE',  ( -1.000000000000000000, -8.163404592832032979E-16, 0.000000000000000000 ) ) ;
#12793=ORIENTED_EDGE ( 'NONE', *, *, #87035, .F. ) ;
#12797=CARTESIAN_POINT ( 'NONE',  ( 81.84766347661002328, -83.77844715994096703, 55.21780685541800437 ) ) ;
#12806=CYLINDRICAL_SURFACE ( 'NONE', #27488, 8.999999999999994671 ) ;
#12807=PLANE ( 'NONE',  #32565 ) ;
#12815=CARTESIAN_POINT ( 'NONE',  ( 147.0667039024470171, -101.1152392874521126, 245.7200378389940170 ) ) ;
#12824=CARTESIAN_POINT ( 'NONE',  ( 145.4713219652040834, -135.8544957252408949, 247.4783998280190076 ) ) ;
#12825=EDGE_LOOP ( 'NONE', ( #44983, #30253, #88553, #3980 ) ) ;
#12858=CARTESIAN_POINT ( 'NONE',  ( 69.56670390244704549, -118.2784471599409812, 45.21780685541799727 ) ) ;
#12859=DIRECTION ( 'NONE',  ( -3.100000000000000258E-29, 3.100000000000000044E-14, 1.000000000000000000 ) ) ;
#12864=VECTOR ( 'NONE', #85937, 1000.000000000000000 ) ;
#12887=ADVANCED_FACE ( 'NONE', ( #21203 ), #37068, .F. ) ;
#12904=FILL_AREA_STYLE ('',( #67855 ) ) ;
#12919=CARTESIAN_POINT ( 'NONE',  ( 107.0667039024470313, -104.2784471599420755, -19.78219314458201694 ) ) ;
#12926=DIRECTION ( 'NONE',  ( 3.100000000000000258E-29, -3.100000000000000044E-14, -1.000000000000000000 ) ) ;
#12953=FACE_OUTER_BOUND ( 'NONE', #25311, .T. ) ;
#12961=EDGE_LOOP ( 'NONE', ( #46566, #51561, #86350, #44808, #22333, #89842 ) ) ;
#12977=ORIENTED_EDGE ( 'NONE', *, *, #46724, .T. ) ;
#12987=VERTEX_POINT ( 'NONE', #49333 ) ;
#13007=EDGE_LOOP ( 'NONE', ( #61397, #49239, #14174, #50224 ) ) ;
#13023=EDGE_CURVE ( 'NONE', #13042, #28081, #23459, .T. ) ;
#13032=EDGE_CURVE ( 'NONE', #9271, #67598, #37519, .T. ) ;
#13040=VERTEX_POINT ( 'NONE', #24329 ) ;
#13042=VERTEX_POINT ( 'NONE', #87450 ) ;
#13044=ORIENTED_EDGE ( 'NONE', *, *, #29691, .F. ) ;
#13047=CARTESIAN_POINT ( 'NONE',  ( 129.9879594898645792, -139.1139133488901223, 247.5865165982399958 ) ) ;
#13056=FACE_OUTER_BOUND ( 'NONE', #25871, .T. ) ;
#13076=ORIENTED_EDGE ( 'NONE', *, *, #9927, .F. ) ;
#13097=EDGE_LOOP ( 'NONE', ( #86654, #8755, #61773, #34359, #41546, #31577 ) ) ;
#13137=CARTESIAN_POINT ( 'NONE',  ( 107.0667039024470313, -104.2784471599418197, -11.78219314458200984 ) ) ;
#13156=EDGE_LOOP ( 'NONE', ( #58346, #12716, #28827, #19212 ) ) ;
#13159=CARTESIAN_POINT ( 'NONE',  ( 135.5667039024470455, -118.2784471599408960, 45.21780685541799727 ) ) ;
#13168=LINE ( 'NONE', #81292, #69009 ) ;
#13169=ORIENTED_EDGE ( 'NONE', *, *, #48854, .F. ) ;
#13170=ORIENTED_EDGE ( 'NONE', *, *, #5285, .T. ) ;
#13177=ADVANCED_FACE ( 'NONE', ( #32350 ), #53676, .F. ) ;
#13194=CARTESIAN_POINT ( 'NONE',  ( 122.2221484686747459, -107.5284471599419192, -21.78219314458190681 ) ) ;
#13221=CARTESIAN_POINT ( 'NONE',  ( 91.91125933621934507, -111.8737466215625744, -11.78219314458178779 ) ) ;
#13238=CARTESIAN_POINT ( 'NONE',  ( 121.3693057586265809, -136.8327113968526305, 248.4142799812389910 ) ) ;
#13239=EDGE_CURVE ( 'NONE', #49274, #27685, #12375, .T. ) ;
#13246=CARTESIAN_POINT ( 'NONE',  ( 110.7536356736639078, -102.7271463785358492, -19.78219314458207378 ) ) ;
#13262=CARTESIAN_POINT ( 'NONE',  ( 145.3578527675120142, -69.40277113351952210, 247.4783998280190076 ) ) ;
#13278=ORIENTED_EDGE ( 'NONE', *, *, #83229, .T. ) ;
#13304=ORIENTED_EDGE ( 'NONE', *, *, #83230, .F. ) ;
#13318=DIRECTION ( 'NONE',  ( -1.000000000000000000, -1.181088324069315053E-15, 0.000000000000000000 ) ) ;
#13324=ORIENTED_EDGE ( 'NONE', *, *, #54781, .T. ) ;
#13346=CARTESIAN_POINT ( 'NONE',  ( 107.0667039024470313, -104.2784471599409528, 45.21780685541799727 ) ) ;
#13374=EDGE_LOOP ( 'NONE', ( #79789, #46053, #73118, #6610 ) ) ;
#13382=CIRCLE ( 'NONE', #77187, 17.00000000000000000 ) ;
#13389=ORIENTED_EDGE ( 'NONE', *, *, #2224, .T. ) ;
#13392=CARTESIAN_POINT ( 'NONE',  ( 70.06796229133446730, -140.6784471599409869, 245.5026818104030042 ) ) ;
#13417=ADVANCED_FACE ( 'NONE', ( #36846 ), #65001, .T. ) ;
#13431=VERTEX_POINT ( 'NONE', #24120 ) ;
#13448=LINE ( 'NONE', #61577, #9900 ) ;
#13452=LINE ( 'NONE', #89318, #66679 ) ;
#13461=AXIS2_PLACEMENT_3D ( 'NONE', #23891, #31127, #58826 ) ;
#13479=B_SPLINE_CURVE_WITH_KNOTS ( 'NONE', 3,
 ( #59942, #46309, #82224, #11820, #19978, #47659 ),
 .UNSPECIFIED., .F., .F.,
 ( 4, 2, 4 ),
 ( 1.223758863293699992E-06, 0.0009153852925891950649, 0.001829959312313299931 ),
 .UNSPECIFIED. ) ;
#13524=EDGE_CURVE ( 'NONE', #78255, #30086, #37055, .T. ) ;
#13525=CARTESIAN_POINT ( 'NONE',  ( 145.3076464064830873, -69.48838775773263876, 247.4862654744191843 ) ) ;
#13528=CARTESIAN_POINT ( 'NONE',  ( 89.89786210216969664, -69.33318169163436551, 247.6453889683499767 ) ) ;
#13537=ORIENTED_EDGE ( 'NONE', *, *, #73590, .T. ) ;
#13561=FACE_OUTER_BOUND ( 'NONE', #51610, .T. ) ;
#13577=ADVANCED_FACE ( 'NONE', ( #17304 ), #44984, .F. ) ;
#13595=ADVANCED_FACE ( 'NONE', ( #67678 ), #46313, .F. ) ;
#13603=EDGE_CURVE ( 'NONE', #89615, #5243, #80878, .T. ) ;
#13609=EDGE_LOOP ( 'NONE', ( #37790, #66839, #87375, #40221, #13870 ) ) ;
#13620=ADVANCED_FACE ( 'NONE', ( #79541 ), #18634, .F. ) ;
#13624=ORIENTED_EDGE ( 'NONE', *, *, #65176, .T. ) ;
#13642=AXIS2_PLACEMENT_3D ( 'NONE', #68055, #19903, #61228 ) ;
#13656=CARTESIAN_POINT ( 'NONE',  ( 106.0988357118831118, -121.2196481995798507, -19.23816774841949240 ) ) ;
#13676=CARTESIAN_POINT ( 'NONE',  ( 103.6786524251748460, -132.6284614801578243, 250.2203867545810283 ) ) ;
#13685=CARTESIAN_POINT ( 'NONE',  ( 68.69857366530352749, -82.21785355595537226, 247.5323269625177716 ) ) ;
#13704=CARTESIAN_POINT ( 'NONE',  ( 141.2325875157518453, -122.8456360496983137, 248.3919668373590071 ) ) ;
#13730=FACE_OUTER_BOUND ( 'NONE', #77812, .T. ) ;
#13732=DIRECTION ( 'NONE',  ( 1.000000000000000000, 1.000000000000000078E-15, 0.000000000000000000 ) ) ;
#13736=ORIENTED_EDGE ( 'NONE', *, *, #69065, .T. ) ;
#13737=ADVANCED_FACE ( 'NONE', ( #42193 ), #82227, .F. ) ;
#13744=DIRECTION ( 'NONE',  ( -0.5000000000000015543, 0.8660254037844377084, -2.602085213965216006E-14 ) ) ;
#13747=VECTOR ( 'NONE', #57120, 1000.000000000000000 ) ;
#13764=AXIS2_PLACEMENT_3D ( 'NONE', #28925, #15301, #1673 ) ;
#13770=VECTOR ( 'NONE', #41923, 1000.000000000000000 ) ;
#13772=AXIS2_PLACEMENT_3D ( 'NONE', #74490, #4558, #80420 ) ;
#13810=LINE ( 'NONE', #53319, #26230 ) ;
#13813=EDGE_CURVE ( 'NONE', #56525, #67362, #13168, .T. ) ;
#13823=CARTESIAN_POINT ( 'NONE',  ( 56.06670390244700997, -79.67844715994098692, 190.2178068554179902 ) ) ;
#13828=ORIENTED_EDGE ( 'NONE', *, *, #58596, .F. ) ;
#13838=CARTESIAN_POINT ( 'NONE',  ( 161.0667039024469886, -67.87844715994089029, 55.21780685541800437 ) ) ;
#13843=CARTESIAN_POINT ( 'NONE',  ( 68.20141520875638719, -68.96305191817310742, 247.2983592438824587 ) ) ;
#13846=EDGE_LOOP ( 'NONE', ( #65648, #6170, #76256, #12115 ) ) ;
#13857=CARTESIAN_POINT ( 'NONE',  ( 146.0042039024470171, -68.87844715994090450, 222.2178068554179902 ) ) ;
#13861=CARTESIAN_POINT ( 'NONE',  ( 144.1829449321824654, -138.0544793359106848, 247.6577929143110168 ) ) ;
#13870=ORIENTED_EDGE ( 'NONE', *, *, #35319, .F. ) ;
#13876=VERTEX_POINT ( 'NONE', #43082 ) ;
#13899=CARTESIAN_POINT ( 'NONE',  ( 124.0667039024470313, -104.2784471599417486, -9.937637710810031777 ) ) ;
#13907=CARTESIAN_POINT ( 'NONE',  ( 68.12920390244700286, -68.87844715994098976, 55.21780685541800437 ) ) ;
#13926=DIRECTION ( 'NONE',  ( -3.100000000000000258E-29, 3.100000000000000044E-14, 1.000000000000000000 ) ) ;
#13935=CARTESIAN_POINT ( 'NONE',  ( 143.5667039024469886, -67.87844715994090450, 55.21780685541800437 ) ) ;
#13936=CARTESIAN_POINT ( 'NONE',  ( 145.2632846747241899, -139.1299635158950423, 246.6334900878847520 ) ) ;
#13951=CARTESIAN_POINT ( 'NONE',  ( 140.0667039024470171, -90.27844715994091018, 45.21780685541799727 ) ) ;
#13954=VECTOR ( 'NONE', #46000, 1000.000000000000000 ) ;
#13958=AXIS2_PLACEMENT_3D ( 'NONE', #18866, #46990, #20219 ) ;
#13978=EDGE_CURVE ( 'NONE', #82359, #18397, #10699, .T. ) ;
#13987=CARTESIAN_POINT ( 'NONE',  ( 108.0667039024470455, -121.2010968907524529, -19.26696060647547881 ) ) ;
#13996=EDGE_LOOP ( 'NONE', ( #52890, #24026 ) ) ;
#14000=CARTESIAN_POINT ( 'NONE',  ( 154.5667039024469886, -67.87844715994090450, 120.2178068554179902 ) ) ;
#14018=LINE ( 'NONE', #75805, #61078 ) ;
#14021=CARTESIAN_POINT ( 'NONE',  ( 112.0840054422653935, -139.4321760210394814, 247.7260698222571307 ) ) ;
#14041=DIRECTION ( 'NONE',  ( -3.100000000000000258E-29, 3.100000000000000044E-14, 1.000000000000000000 ) ) ;
#14079=AXIS2_PLACEMENT_3D ( 'NONE', #9412, #8981, #21713 ) ;
#14091=CIRCLE ( 'NONE', #64867, 3.500000000000003109 ) ;
#14094=ORIENTED_EDGE ( 'NONE', *, *, #86196, .T. ) ;
#14096=EDGE_CURVE ( 'NONE', #26687, #29557, #89376, .T. ) ;
#14100=CARTESIAN_POINT ( 'NONE',  ( 77.06670390244703128, -118.2784471599409812, 51.21780685541800437 ) ) ;
#14113=EDGE_CURVE ( 'NONE', #68597, #84959, #32812, .T. ) ;
#14122=ORIENTED_EDGE ( 'NONE', *, *, #5605, .F. ) ;
#14128=CARTESIAN_POINT ( 'NONE',  ( 107.0667039024470313, -104.2784471599414502, 0.2178068554180012661 ) ) ;
#14132=CARTESIAN_POINT ( 'NONE',  ( 68.24424899846859205, -67.86899452490857243, 247.3945403487729777 ) ) ;
#14142=EDGE_CURVE ( 'NONE', #88900, #48200, #37177, .T. ) ;
#14150=EDGE_CURVE ( 'NONE', #12139, #71132, #75864, .T. ) ;
#14157=CARTESIAN_POINT ( 'NONE',  ( 127.3855721265797456, -122.7922957798182324, 250.2191008560389776 ) ) ;
#14161=ORIENTED_EDGE ( 'NONE', *, *, #32658, .F. ) ;
#14165=CARTESIAN_POINT ( 'NONE',  ( 86.72755763596092038, -85.76982405743865456, 250.2178068554179902 ) ) ;
#14173=VERTEX_POINT ( 'NONE', #83338 ) ;
#14174=ORIENTED_EDGE ( 'NONE', *, *, #21162, .T. ) ;
#14192=AXIS2_PLACEMENT_3D ( 'NONE', #66691, #46682, #4478 ) ;
#14215=VECTOR ( 'NONE', #63073, 1000.000000000000000 ) ;
#14224=CIRCLE ( 'NONE', #76609, 32.50000000000000711 ) ;
#14230=CIRCLE ( 'NONE', #76613, 1.999999999999995781 ) ;
#14245=PLANE ( 'NONE',  #19896 ) ;
#14249=DIRECTION ( 'NONE',  ( 0.000000000000000000, 0.000000000000000000, -1.000000000000000000 ) ) ;
#14254=CARTESIAN_POINT ( 'NONE',  ( 92.84710890992452903, -94.98933252893162660, -19.21044887263828471 ) ) ;
#14281=AXIS2_PLACEMENT_3D ( 'NONE', #73323, #24299, #51965 ) ;
#14320=CARTESIAN_POINT ( 'NONE',  ( 107.0667039024470313, -104.2784471599420755, -19.78219314458201694 ) ) ;
#14341=PLANE ( 'NONE',  #37977 ) ;
#14352=AXIS2_PLACEMENT_3D ( 'NONE', #28215, #70018, #66764 ) ;
#14357=LINE ( 'NONE', #36133, #39843 ) ;
#14363=DIRECTION ( 'NONE',  ( 0.000000000000000000, 0.000000000000000000, 1.000000000000000000 ) ) ;
#14374=LINE ( 'NONE', #22986, #29259 ) ;
#14378=DIRECTION ( 'NONE',  ( -3.100000000000000258E-29, 3.100000000000000044E-14, 1.000000000000000000 ) ) ;
#14388=ORIENTED_EDGE ( 'NONE', *, *, #39819, .F. ) ;
#14409=DIRECTION ( 'NONE',  ( 0.000000000000000000, 0.000000000000000000, 1.000000000000000000 ) ) ;
#14414=DIRECTION ( 'NONE',  ( -3.100000000000000258E-29, 3.100000000000000044E-14, 1.000000000000000000 ) ) ;
#14419=CIRCLE ( 'NONE', #24528, 7.999999999999992895 ) ;
#14421=SHAPE_REPRESENTATION ( 'Drilling Spindle Head', ( #50656 ), #4304 ) ;
#14423=EDGE_CURVE ( 'NONE', #35871, #66630, #73720, .T. ) ;
#14446=ORIENTED_EDGE ( 'NONE', *, *, #19754, .T. ) ;
#14458=CARTESIAN_POINT ( 'NONE',  ( 127.0667052882549797, -69.62844715994091871, 222.2178068554179902 ) ) ;
#14470=DIRECTION ( 'NONE',  ( 1.000000000000000000, 1.000000000000000078E-15, 0.000000000000000000 ) ) ;
#14482=LINE ( 'NONE', #48962, #22999 ) ;
#14487=VERTEX_POINT ( 'NONE', #5586 ) ;
#14490=VERTEX_POINT ( 'NONE', #81895 ) ;
#14491=EDGE_LOOP ( 'NONE', ( #63711, #38033, #31133, #40883, #25757, #61120, #48992, #39101, #78134, #88008, #46204, #24166, #35264, #35702, #89487, #8154, #47794, #17875, #9176, #75874, #59865, #55822 ) ) ;
#14496=LINE ( 'NONE', #8120, #14215 ) ;
#14500=FACE_OUTER_BOUND ( 'NONE', #13374, .T. ) ;
#14526=ORIENTED_EDGE ( 'NONE', *, *, #35214, .F. ) ;
#14556=CARTESIAN_POINT ( 'NONE',  ( 151.0667039024469886, -67.87844715994090450, 190.2178068554179902 ) ) ;
#14559=ADVANCED_FACE ( 'NONE', ( #68260 ), #88265, .T. ) ;
#14577=VECTOR ( 'NONE', #16325, 1000.000000000000000 ) ;
#14585=DIRECTION ( 'NONE',  ( 0.000000000000000000, 0.000000000000000000, 1.000000000000000000 ) ) ;
#14591=CARTESIAN_POINT ( 'NONE',  ( 113.7313622454167046, -108.7036397175020994, -19.78219314458187839 ) ) ;
#14592=EDGE_LOOP ( 'NONE', ( #48302, #21990, #89799, #10258 ) ) ;
#14609=AXIS2_PLACEMENT_3D ( 'NONE', #7763, #58146, #64966 ) ;
#14610=ORIENTED_EDGE ( 'NONE', *, *, #58596, .T. ) ;
#14621=CARTESIAN_POINT ( 'NONE',  ( 107.5667039024470313, -108.2470741265382799, 2.217806855418114065 ) ) ;
#14627=ORIENTED_EDGE ( 'NONE', *, *, #84152, .T. ) ;
#14632=CARTESIAN_POINT ( 'NONE',  ( 147.0667039027857470, -137.6784471596013191, 245.4218662566959779 ) ) ;
#14634=CIRCLE ( 'NONE', #71251, 32.50000000000000711 ) ;
#14645=ORIENTED_EDGE ( 'NONE', *, *, #37613, .F. ) ;
#14653=AXIS2_PLACEMENT_3D ( 'NONE', #43686, #71422, #36884 ) ;
#14666=DIRECTION ( 'NONE',  ( 3.100000000000000258E-29, -3.100000000000000044E-14, -1.000000000000000000 ) ) ;
#14675=ORIENTED_EDGE ( 'NONE', *, *, #77567, .F. ) ;
#14677=DIRECTION ( 'NONE',  ( -1.000000000000000000, -1.075267683398002218E-15, 2.333298185338067508E-30 ) ) ;
#14687=CARTESIAN_POINT ( 'NONE',  ( 70.42775326414512449, -140.0375196470091055, 247.0014259009493856 ) ) ;
#14695=( NAMED_UNIT ( * ) PLANE_ANGLE_UNIT ( ) SI_UNIT ( $, .RADIAN. ) );
#14708=CARTESIAN_POINT ( 'NONE',  ( 127.4058501689331280, -122.7870702624433221, 250.2178068554179902 ) ) ;
#14727=LINE ( 'NONE', #42400, #73663 ) ;
#14730=FACE_OUTER_BOUND ( 'NONE', #77515, .T. ) ;
#14736=LINE ( 'NONE', #63319, #25128 ) ;
#14738=ORIENTED_EDGE ( 'NONE', *, *, #85717, .F. ) ;
#14739=VERTEX_POINT ( 'NONE', #21905 ) ;
#14748=ADVANCED_FACE ( 'NONE', ( #8267 ), #27356, .T. ) ;
#14750=AXIS2_PLACEMENT_3D ( 'NONE', #53626, #88201, #66833 ) ;
#14751=DIRECTION ( 'NONE',  ( 7.076552332833900719E-16, -1.000000000000000000, 3.100000000000000044E-14 ) ) ;
#14753=CARTESIAN_POINT ( 'NONE',  ( 67.20685546831352042, -68.01262586362689433, 246.2275592078436546 ) ) ;
#14758=EDGE_CURVE ( 'NONE', #86303, #37134, #930, .T. ) ;
#14759=ORIENTED_EDGE ( 'NONE', *, *, #35705, .T. ) ;
#14761=LINE ( 'NONE', #42876, #79534 ) ;
#14772=CARTESIAN_POINT ( 'NONE',  ( 107.9747653995834327, -87.30271670975442078, -11.78219314458253741 ) ) ;
#14796=CARTESIAN_POINT ( 'NONE',  ( 147.0667039024469886, -67.87844715994090450, 222.2178068554179902 ) ) ;
#14806=ORIENTED_EDGE ( 'NONE', *, *, #8903, .T. ) ;
#14810=CARTESIAN_POINT ( 'NONE',  ( 107.0667039024470313, -104.2784471599420897, -20.48315503890502143 ) ) ;
#14811=CARTESIAN_POINT ( 'NONE',  ( 107.0667039024470313, -104.2784471599409102, 17.71780685541799016 ) ) ;
#14829=DIRECTION ( 'NONE',  ( 1.000000000000000000, 9.408669700213195533E-16, 0.000000000000000000 ) ) ;
#14834=CARTESIAN_POINT ( 'NONE',  ( 144.0667039004811443, -140.6784471619068029, 245.4415720117440003 ) ) ;
#14851=ORIENTED_EDGE ( 'NONE', *, *, #60535, .F. ) ;
#14875=CYLINDRICAL_SURFACE ( 'NONE', #39752, 1.999999999999995781 ) ;
#14912=CARTESIAN_POINT ( 'NONE',  ( 108.0667039024470171, -87.35579742913164125, -19.26696060647653397 ) ) ;
#14923=ORIENTED_EDGE ( 'NONE', *, *, #9101, .F. ) ;
#14924=PLANE ( 'NONE',  #82471 ) ;
#14937=ADVANCED_FACE ( 'NONE', ( #87251 ), #73606, .T. ) ;
#14944=DIRECTION ( 'NONE',  ( 3.100000000000000258E-29, -3.100000000000000044E-14, -1.000000000000000000 ) ) ;
#14946=ADVANCED_FACE ( 'NONE', ( #4575 ), #25914, .T. ) ;
#14974=DIRECTION ( 'NONE',  ( -0.8660254037844382635, -0.5000000000000008882, 1.550000000000000022E-14 ) ) ;
#14986=CARTESIAN_POINT ( 'NONE',  ( 68.87418703512655327, -69.52506677730903561, 247.4937269829859758 ) ) ;
#15006=PLANE ( 'NONE',  #26830 ) ;
#15031=CARTESIAN_POINT ( 'NONE',  ( 68.23087527387866658, -137.6857029198856992, 247.4029867184769955 ) ) ;
#15034=ORIENTED_EDGE ( 'NONE', *, *, #59782, .T. ) ;
#15058=EDGE_CURVE ( 'NONE', #9292, #82261, #35393, .T. ) ;
#15067=DIRECTION ( 'NONE',  ( -1.000000000000000000, -1.541976423090496028E-15, 0.000000000000000000 ) ) ;
#15075=VECTOR ( 'NONE', #78075, 999.9999999999998863 ) ;
#15127=CARTESIAN_POINT ( 'NONE',  ( 70.74335932947460037, -139.3331411919284619, 247.4266426818775244 ) ) ;
#15138=SURFACE_STYLE_USAGE ( .BOTH. , #61475 ) ;
#15147=DIRECTION ( 'NONE',  ( 1.000000000000000000, 0.000000000000000000, 0.000000000000000000 ) ) ;
#15149=CARTESIAN_POINT ( 'NONE',  ( 97.06670390244703128, -109.9573555057410772, 19.21780685541815714 ) ) ;
#15152=CARTESIAN_POINT ( 'NONE',  ( 119.9305508289311888, -128.6589936823970106, 250.2178068554180470 ) ) ;
#15157=LINE ( 'NONE', #78294, #2927 ) ;
#15171=CARTESIAN_POINT ( 'NONE',  ( 104.0667030381801936, -67.87844715994094713, 173.2178086137559774 ) ) ;
#15189=CARTESIAN_POINT ( 'NONE',  ( 67.06824679800834588, -67.87939406239482310, 245.5735631681239397 ) ) ;
#15205=DIRECTION ( 'NONE',  ( -1.000000000000000078E-15, 1.000000000000000000, 0.000000000000000000 ) ) ;
#15213=ORIENTED_EDGE ( 'NONE', *, *, #41855, .T. ) ;
#15221=VERTEX_POINT ( 'NONE', #77204 ) ;
#15247=ORIENTED_EDGE ( 'NONE', *, *, #78270, .T. ) ;
#15251=EDGE_CURVE ( 'NONE', #42066, #23612, #50364, .T. ) ;
#15257=PLANE ( 'NONE',  #37952 ) ;
#15301=DIRECTION ( 'NONE',  ( -3.100000000000000258E-29, 3.100000000000000044E-14, 1.000000000000000000 ) ) ;
#15318=PLANE ( 'NONE',  #57194 ) ;
#15323=VERTEX_POINT ( 'NONE', #22244 ) ;
#15330=ORIENTED_EDGE ( 'NONE', *, *, #48704, .F. ) ;
#15332=AXIS2_PLACEMENT_3D ( 'NONE', #36069, #49681, #21102 ) ;
#15337=VECTOR ( 'NONE', #15722, 1000.000000000000000 ) ;
#15400=CARTESIAN_POINT ( 'NONE',  ( 107.0667039024470313, -104.2784471599418197, -11.78219314458200984 ) ) ;
#15404=VERTEX_POINT ( 'NONE', #45769 ) ;
#15431=ORIENTED_EDGE ( 'NONE', *, *, #87474, .F. ) ;
#15435=CARTESIAN_POINT ( 'NONE',  ( 74.06670390244704549, -118.2784471599409812, 51.21780685541800437 ) ) ;
#15440=CARTESIAN_POINT ( 'NONE',  ( 68.86273219497338971, -69.51591775960335440, 247.4919776621595418 ) ) ;
#15441=ADVANCED_FACE ( 'NONE', ( #33507, #20343 ), #20782, .T. ) ;
#15445=DIRECTION ( 'NONE',  ( 3.100000000000000258E-29, -3.100000000000000044E-14, -1.000000000000000000 ) ) ;
#15462=ORIENTED_EDGE ( 'NONE', *, *, #31086, .F. ) ;
#15465=AXIS2_PLACEMENT_3D ( 'NONE', #15888, #72638, #86260 ) ;
#15491=CARTESIAN_POINT ( 'NONE',  ( 67.36333724445186988, -137.6828925929944774, 246.8602380403289942 ) ) ;
#15493=DIRECTION ( 'NONE',  ( -0.5000000000000015543, 0.8660254037844377084, -2.688821387764056676E-14 ) ) ;
#15498=CARTESIAN_POINT ( 'NONE',  ( 103.3797721312301405, -102.7271463785358492, -19.78219314458207378 ) ) ;
#15502=CARTESIAN_POINT ( 'NONE',  ( 93.91125933621933086, -96.68314769832107913, -11.78219314458223188 ) ) ;
#15506=ADVANCED_FACE ( 'NONE', ( #50717 ), #50260, .T. ) ;
#15507=DIRECTION ( 'NONE',  ( -3.100000000000000258E-29, 3.100000000000000044E-14, 1.000000000000000000 ) ) ;
#15515=PLANE ( 'NONE',  #22292 ) ;
#15516=DIRECTION ( 'NONE',  ( -3.100000000000000258E-29, 3.100000000000000044E-14, 1.000000000000000000 ) ) ;
#15539=ORIENTED_EDGE ( 'NONE', *, *, #72068, .T. ) ;
#15544=VECTOR ( 'NONE', #62428, 1000.000000000000000 ) ;
#15550=VERTEX_POINT ( 'NONE', #8049 ) ;
#15583=DIRECTION ( 'NONE',  ( 3.100000000000000258E-29, -3.100000000000000044E-14, -1.000000000000000000 ) ) ;
#15597=CARTESIAN_POINT ( 'NONE',  ( 68.69838760978726100, -139.2979692165780818, 245.8480134095270557 ) ) ;
#15607=CARTESIAN_POINT ( 'NONE',  ( 114.6154092934514495, -130.7908339518063769, 250.2178068554180470 ) ) ;
#15611=VECTOR ( 'NONE', #41679, 999.9999999999998863 ) ;
#15620=ORIENTED_EDGE ( 'NONE', *, *, #87795, .T. ) ;
#15626=DIRECTION ( 'NONE',  ( -1.000000000000000000, -1.000000000000000078E-15, 0.000000000000000000 ) ) ;
#15629=CARTESIAN_POINT ( 'NONE',  ( 144.7726661055232853, -137.4541655641505145, 247.5777877757870158 ) ) ;
#15636=ADVANCED_FACE ( 'NONE', ( #4809 ), #60192, .F. ) ;
#15637=DIRECTION ( 'NONE',  ( -1.000000000000000000, -1.541976423090496028E-15, 0.000000000000000000 ) ) ;
#15642=CARTESIAN_POINT ( 'NONE',  ( 144.0667039024470455, -124.7784471599409102, 55.21780685541800437 ) ) ;
#15660=EDGE_CURVE ( 'NONE', #20369, #80721, #65597, .T. ) ;
#15665=ORIENTED_EDGE ( 'NONE', *, *, #25606, .F. ) ;
#15677=LINE ( 'NONE', #58761, #53135 ) ;
#15703=DIRECTION ( 'NONE',  ( -3.100000000000000258E-29, 3.100000000000000044E-14, 1.000000000000000000 ) ) ;
#15722=DIRECTION ( 'NONE',  ( 1.000000000000000078E-15, -1.000000000000000000, 0.000000000000000000 ) ) ;
#15729=ADVANCED_FACE ( 'NONE', ( #65681 ), #17106, .T. ) ;
#15731=ORIENTED_EDGE ( 'NONE', *, *, #36963, .T. ) ;
#15760=VECTOR ( 'NONE', #81793, 1000.000000000000000 ) ;
#15779=AXIS2_PLACEMENT_3D ( 'NONE', #38643, #19100, #46785 ) ;
#15844=EDGE_LOOP ( 'NONE', ( #51855, #87941, #47340, #61937, #19238 ) ) ;
#15884=CARTESIAN_POINT ( 'NONE',  ( 114.6444261855607891, -91.15344715994180547, -11.78219314458242550 ) ) ;
#15888=CARTESIAN_POINT ( 'NONE',  ( 107.0667039024470171, -89.08784823670062281, -21.78219314458248945 ) ) ;
#15905=AXIS2_PLACEMENT_3D ( 'NONE', #55887, #83636, #29114 ) ;
#15946=DIRECTION ( 'NONE',  ( -0.4999999999999989453, -0.8660254037844392627, 2.684678751731760294E-14 ) ) ;
#15952=ORIENTED_EDGE ( 'NONE', *, *, #9927, .T. ) ;
#15964=CARTESIAN_POINT ( 'NONE',  ( 70.56670390244700286, -68.87844715994098976, 222.2178068554179902 ) ) ;
#15973=ADVANCED_FACE ( 'NONE', ( #54713 ), #29173, .F. ) ;
#15978=DIRECTION ( 'NONE',  ( 1.000000000000000078E-15, -1.000000000000000000, 0.000000000000000000 ) ) ;
#15979=VECTOR ( 'NONE', #58225, 1000.000000000000000 ) ;
#15980=FACE_OUTER_BOUND ( 'NONE', #38316, .T. ) ;
#15982=DIRECTION ( 'NONE',  ( 1.000000000000000000, 1.000000000000000078E-15, 0.000000000000000000 ) ) ;
#15986=CARTESIAN_POINT ( 'NONE',  ( 122.2189888861420286, -96.57077177932983147, -11.78219314458225853 ) ) ;
#15994=CARTESIAN_POINT ( 'NONE',  ( 122.2221484686747459, -111.8737466215628729, -21.78219314458179667 ) ) ;
#16005=CYLINDRICAL_SURFACE ( 'NONE', #14653, 4.500000000000003553 ) ;
#16078=EDGE_CURVE ( 'NONE', #45292, #58396, #59866, .T. ) ;
#16087=CARTESIAN_POINT ( 'NONE',  ( 116.3167039024470029, -67.87844715994093292, 222.2178068554179902 ) ) ;
#16088=CARTESIAN_POINT ( 'NONE',  ( 108.0667039024470171, -87.35579742913164125, -19.26696060647653397 ) ) ;
#16120=ORIENTED_EDGE ( 'NONE', *, *, #74615, .F. ) ;
#16127=EDGE_LOOP ( 'NONE', ( #44050, #58211, #73365 ) ) ;
#16129=ADVANCED_FACE ( 'NONE', ( #71854 ), #37777, .T. ) ;
#16137=FACE_OUTER_BOUND ( 'NONE', #16234, .T. ) ;
#16138=CARTESIAN_POINT ( 'NONE',  ( 85.44094044773511598, -87.19737211520767062, 250.2190963482990185 ) ) ;
#16150=CARTESIAN_POINT ( 'NONE',  ( 147.0665874381622018, -67.87844715994090450, 245.5130140176639770 ) ) ;
#16160=CARTESIAN_POINT ( 'NONE',  ( 146.3069282193933986, -137.2669017349363685, 247.0814054964307616 ) ) ;
#16161=AXIS2_PLACEMENT_3D ( 'NONE', #66555, #81564, #32926 ) ;
#16187=VECTOR ( 'NONE', #22085, 999.9999999999998863 ) ;
#16209=CARTESIAN_POINT ( 'NONE',  ( 82.02983075842483629, -115.7792181415380668, 250.2178068554180470 ) ) ;
#16217=ORIENTED_EDGE ( 'NONE', *, *, #18842, .F. ) ;
#16218=EDGE_LOOP ( 'NONE', ( #52284, #21553, #20591, #73108 ) ) ;
#16219=AXIS2_PLACEMENT_3D ( 'NONE', #34035, #73716, #56550 ) ;
#16231=AXIS2_PLACEMENT_3D ( 'NONE', #25397, #67177, #80833 ) ;
#16234=EDGE_LOOP ( 'NONE', ( #3955, #12132, #26248, #16328, #81672, #67220, #80584, #59459, #19538, #12196, #19407, #50809 ) ) ;
#16247=EDGE_LOOP ( 'NONE', ( #39045, #54599 ) ) ;
#16248=LINE ( 'NONE', #76678, #22878 ) ;
#16275=ORIENTED_EDGE ( 'NONE', *, *, #76357, .F. ) ;
#16286=CARTESIAN_POINT ( 'NONE',  ( 71.47170404114027065, -139.6113389983086961, 247.4111996305669834 ) ) ;
#16290=AXIS2_PLACEMENT_3D ( 'NONE', #38938, #3981, #18954 ) ;
#16294=CARTESIAN_POINT ( 'NONE',  ( 118.5667039024470313, -104.2784471599411376, 0.2178068554180012661 ) ) ;
#16301=EDGE_CURVE ( 'NONE', #4381, #63654, #58397, .T. ) ;
#16319=ORIENTED_EDGE ( 'NONE', *, *, #9309, .F. ) ;
#16325=DIRECTION ( 'NONE',  ( 3.100000000000000258E-29, -3.100000000000000044E-14, -1.000000000000000000 ) ) ;
#16328=ORIENTED_EDGE ( 'NONE', *, *, #20803, .T. ) ;
#16335=VERTEX_POINT ( 'NONE', #31837 ) ;
#16342=CARTESIAN_POINT ( 'NONE',  ( 143.5625297611475730, -139.4754646311774877, 247.4327973477450087 ) ) ;
#16346=CARTESIAN_POINT ( 'NONE',  ( 121.2542802781108406, -113.5872461203042292, -19.23816774841974464 ) ) ;
#16371=LINE ( 'NONE', #30887, #52735 ) ;
#16404=EDGE_CURVE ( 'NONE', #35731, #75012, #55840, .T. ) ;
#16416=CIRCLE ( 'NONE', #52606, 11.49999999999999645 ) ;
#16417=CARTESIAN_POINT ( 'NONE',  ( 140.0667039024470171, -90.27844715994091018, 45.21780685541799727 ) ) ;
#16425=CARTESIAN_POINT ( 'NONE',  ( 120.2221484686747317, -96.68314769832136335, -21.78219314458224076 ) ) ;
#16430=DIRECTION ( 'NONE',  ( 1.000000000000000078E-15, -1.000000000000000000, 0.000000000000000000 ) ) ;
#16444=DIRECTION ( 'NONE',  ( 0.000000000000000000, 0.000000000000000000, 1.000000000000000000 ) ) ;
#16457=CARTESIAN_POINT ( 'NONE',  ( 59.56670390244699576, -67.87844715994098976, 120.2178068554179902 ) ) ;
#16464=DIRECTION ( 'NONE',  ( 1.000000000000000000, 1.000000000000000078E-15, -0.000000000000000000 ) ) ;
#16485=CARTESIAN_POINT ( 'NONE',  ( 69.37738364949149172, -138.6267510924388944, 247.3762624300263155 ) ) ;
#16514=DIRECTION ( 'NONE',  ( -1.000000000000000078E-15, 1.000000000000000000, 0.000000000000000000 ) ) ;
#16515=EDGE_CURVE ( 'NONE', #35035, #85102, #22711, .T. ) ;
#16536=DIRECTION ( 'NONE',  ( 1.000000000000000000, 1.000000000000000078E-15, 0.000000000000000000 ) ) ;
#16581=EDGE_CURVE ( 'NONE', #27442, #78823, #40778, .T. ) ;
#16582=ORIENTED_EDGE ( 'NONE', *, *, #60901, .F. ) ;
#16588=DIRECTION ( 'NONE',  ( -1.000000000000000000, -8.163404592832032979E-16, 0.000000000000000000 ) ) ;
#16589=DIRECTION ( 'NONE',  ( -1.000000000000000000, 0.000000000000000000, 0.000000000000000000 ) ) ;
#16617=EDGE_LOOP ( 'NONE', ( #1369, #24263, #19534, #70022 ) ) ;
#16624=DIRECTION ( 'NONE',  ( -1.000000000000000078E-15, 1.000000000000000000, 0.000000000000000000 ) ) ;
#16625=ADVANCED_FACE ( 'NONE', ( #20795 ), #69844, .F. ) ;
#16647=DIRECTION ( 'NONE',  ( -0.000000000000000000, -0.000000000000000000, -1.000000000000000000 ) ) ;
#16661=CARTESIAN_POINT ( 'NONE',  ( 147.0667039024457665, -137.6758868153238780, 245.5072646551060132 ) ) ;
#16671=ORIENTED_EDGE ( 'NONE', *, *, #86852, .T. ) ;
#16686=ORIENTED_EDGE ( 'NONE', *, *, #71571, .F. ) ;
#16693=CARTESIAN_POINT ( 'NONE',  ( 132.2857443282839824, -83.77844715994092439, 55.21780685541800437 ) ) ;
#16701=DIRECTION ( 'NONE',  ( 0.000000000000000000, 0.000000000000000000, -1.000000000000000000 ) ) ;
#16706=AXIS2_PLACEMENT_3D ( 'NONE', #50698, #36645, #62986 ) ;
#16731=EDGE_CURVE ( 'NONE', #12987, #48763, #12491, .T. ) ;
#16739=DIRECTION ( 'NONE',  ( -1.000000000000000000, -1.734723475976808672E-15, 0.000000000000000000 ) ) ;
#16746=DIRECTION ( 'NONE',  ( -0.000000000000000000, -0.000000000000000000, 1.000000000000000000 ) ) ;
#16782=ORIENTED_EDGE ( 'NONE', *, *, #70207, .F. ) ;
#16787=CARTESIAN_POINT ( 'NONE',  ( 143.7322224575774783, -140.5784730598227839, 246.8085536723579878 ) ) ;
#16788=CARTESIAN_POINT ( 'NONE',  ( 106.5667039024470313, -100.3098201933445068, 2.217806855417892020 ) ) ;
#16796=VERTEX_POINT ( 'NONE', #32916 ) ;
#16801=AXIS2_PLACEMENT_3D ( 'NONE', #86156, #51163, #66130 ) ;
#16832=ORIENTED_EDGE ( 'NONE', *, *, #77825, .T. ) ;
#16847=ORIENTED_EDGE ( 'NONE', *, *, #88739, .T. ) ;
#16866=ORIENTED_EDGE ( 'NONE', *, *, #13032, .T. ) ;
#16873=EDGE_CURVE ( 'NONE', #71994, #77969, #57035, .T. ) ;
#16876=CARTESIAN_POINT ( 'NONE',  ( 114.6444261855608744, -117.4034471599418055, -11.78219314458159239 ) ) ;
#16883=VERTEX_POINT ( 'NONE', #34260 ) ;
#16898=DIRECTION ( 'NONE',  ( 1.000000000000000078E-15, -1.000000000000000000, 0.000000000000000000 ) ) ;
#16915=FACE_OUTER_BOUND ( 'NONE', #33808, .T. ) ;
#16917=EDGE_CURVE ( 'NONE', #14173, #47689, #14736, .T. ) ;
#16920=LINE ( 'NONE', #85972, #7278 ) ;
#16931=CARTESIAN_POINT ( 'NONE',  ( 68.86296241111062955, -139.1369832984686354, 246.6149457656773052 ) ) ;
#16960=CARTESIAN_POINT ( 'NONE',  ( 146.9537589533094888, -137.3494371116456989, 246.8018929578719849 ) ) ;
#16964=ORIENTED_EDGE ( 'NONE', *, *, #19038, .T. ) ;
#16987=CARTESIAN_POINT ( 'NONE',  ( 107.0667039024470313, -104.2784471599420755, -19.78219314458201694 ) ) ;
#17000=DIRECTION ( 'NONE',  ( -1.000000000000000078E-15, 1.000000000000000000, 0.000000000000000000 ) ) ;
#17015=EDGE_LOOP ( 'NONE', ( #24708, #77608, #40015, #80000, #222, #58409 ) ) ;
#17022=LINE ( 'NONE', #31082, #26869 ) ;
#17023=CARTESIAN_POINT ( 'NONE',  ( 68.20286926358554069, -119.2990514172772833, 247.4783998280180128 ) ) ;
#17030=ADVANCED_FACE ( 'NONE', ( #4023 ), #3143, .T. ) ;
#17037=CARTESIAN_POINT ( 'NONE',  ( 143.4594029887166471, -139.4935159556384860, 247.3653129605272056 ) ) ;
#17044=CARTESIAN_POINT ( 'NONE',  ( 67.06670403371455791, -137.6620872545493341, 245.7334057579663238 ) ) ;
#17058=PLANE ( 'NONE',  #1616 ) ;
#17066=VERTEX_POINT ( 'NONE', #4479 ) ;
#17071=AXIS2_PLACEMENT_3D ( 'NONE', #26400, #47272, #38235 ) ;
#17073=VERTEX_POINT ( 'NONE', #51708 ) ;
#17085=ADVANCED_FACE ( 'NONE', ( #18542 ), #59423, .F. ) ;
#17100=ADVANCED_FACE ( 'NONE', ( #25811 ), #61126, .F. ) ;
#17105=EDGE_LOOP ( 'NONE', ( #35930, #23139 ) ) ;
#17106=CYLINDRICAL_SURFACE ( 'NONE', #83061, 2.000000000000001776 ) ;
#17107=ORIENTED_EDGE ( 'NONE', *, *, #70642, .F. ) ;
#17125=CARTESIAN_POINT ( 'NONE',  ( 70.06968321367156705, -140.6784088069870222, 245.5331728854790185 ) ) ;
#17136=VERTEX_POINT ( 'NONE', #27599 ) ;
#17159=ORIENTED_EDGE ( 'NONE', *, *, #80759, .T. ) ;
#17163=AXIS2_PLACEMENT_3D ( 'NONE', #69482, #69033, #21332 ) ;
#17170=EDGE_CURVE ( 'NONE', #56556, #83896, #74413, .T. ) ;
#17172=VERTEX_POINT ( 'NONE', #88940 ) ;
#17177=DIRECTION ( 'NONE',  ( 3.100000000000000258E-29, -3.100000000000000044E-14, -1.000000000000000000 ) ) ;
#17196=ORIENTED_EDGE ( 'NONE', *, *, #24315, .F. ) ;
#17251=DIRECTION ( 'NONE',  ( 3.100000000000000258E-29, -3.100000000000000044E-14, -1.000000000000000000 ) ) ;
#17260=VERTEX_POINT ( 'NONE', #18999 ) ;
#17266=DIRECTION ( 'NONE',  ( -1.000000000000000078E-15, 1.000000000000000000, -3.100000000000000044E-14 ) ) ;
#17286=FACE_OUTER_BOUND ( 'NONE', #5378, .T. ) ;
#17296=LINE ( 'NONE', #44975, #45781 ) ;
#17304=FACE_OUTER_BOUND ( 'NONE', #66015, .T. ) ;
#17316=DIRECTION ( 'NONE',  ( 3.100000000000000258E-29, -3.100000000000000044E-14, -1.000000000000000000 ) ) ;
#17328=CIRCLE ( 'NONE', #40525, 11.49999999999999645 ) ;
#17358=ORIENTED_EDGE ( 'NONE', *, *, #27290, .T. ) ;
#17367=EDGE_CURVE ( 'NONE', #17066, #14490, #31059, .T. ) ;
#17371=CARTESIAN_POINT ( 'NONE',  ( 69.20747379336683025, -138.7952845549384904, 247.2071845478467083 ) ) ;
#17389=EDGE_CURVE ( 'NONE', #44246, #75012, #87579, .T. ) ;
#17405=CARTESIAN_POINT ( 'NONE',  ( 145.3708670603641622, -136.8623670038712987, 247.4903216359130056 ) ) ;
#17429=CARTESIAN_POINT ( 'NONE',  ( 146.7254745405287224, -68.20551812416188397, 246.6136140996082702 ) ) ;
#17436=ORIENTED_EDGE ( 'NONE', *, *, #87304, .T. ) ;
#17441=DIRECTION ( 'NONE',  ( -1.000000000000000000, -1.000000000000000078E-15, 0.000000000000000000 ) ) ;
#17451=EDGE_LOOP ( 'NONE', ( #57177, #1723, #942, #79560, #48969, #129 ) ) ;
#17469=EDGE_LOOP ( 'NONE', ( #51203, #28483 ) ) ;
#17473=LINE ( 'NONE', #22189, #43387 ) ;
#17477=CARTESIAN_POINT ( 'NONE',  ( 70.06670390244703128, -96.32844715994099261, 222.2178068554179902 ) ) ;
#17485=CARTESIAN_POINT ( 'NONE',  ( 68.48770573954575980, -136.9758359881863896, 247.4278779589974135 ) ) ;
#17497=DIRECTION ( 'NONE',  ( 1.000000000000000000, 1.000000000000000078E-15, 0.000000000000000000 ) ) ;
#17505=ORIENTED_EDGE ( 'NONE', *, *, #60540, .F. ) ;
#17522=EDGE_LOOP ( 'NONE', ( #53775, #76330 ) ) ;
#17528=CARTESIAN_POINT ( 'NONE',  ( 115.0439452383991892, -99.09543445804915507, 2.217806855417836509 ) ) ;
#17535=EDGE_LOOP ( 'NONE', ( #9638, #44247 ) ) ;
#17546=ORIENTED_EDGE ( 'NONE', *, *, #55940, .T. ) ;
#17565=CARTESIAN_POINT ( 'NONE',  ( 112.3521431160374675, -140.6784471599409301, 245.8674624188659834 ) ) ;
#17572=AXIS2_PLACEMENT_3D ( 'NONE', #74724, #61084, #40184 ) ;
#17577=AXIS2_PLACEMENT_3D ( 'NONE', #13137, #34453, #27647 ) ;
#17580=DIRECTION ( 'NONE',  ( 1.000000000000000000, 0.000000000000000000, 0.000000000000000000 ) ) ;
#17583=EDGE_CURVE ( 'NONE', #56759, #61997, #78696, .T. ) ;
#17592=ORIENTED_EDGE ( 'NONE', *, *, #20803, .F. ) ;
#17598=VECTOR ( 'NONE', #78935, 1000.000000000000000 ) ;
#17599=EDGE_CURVE ( 'NONE', #21095, #78359, #50944, .T. ) ;
#17609=DIRECTION ( 'NONE',  ( -0.000000000000000000, -0.000000000000000000, -1.000000000000000000 ) ) ;
#17637=VECTOR ( 'NONE', #18296, 1000.000000000000000 ) ;
#17640=ORIENTED_EDGE ( 'NONE', *, *, #62, .F. ) ;
#17644=AXIS2_PLACEMENT_3D ( 'NONE', #12919, #18827, #32894 ) ;
#17647=CIRCLE ( 'NONE', #85888, 24.50000000000000711 ) ;
#17650=LINE ( 'NONE', #66223, #76955 ) ;
#17662=CARTESIAN_POINT ( 'NONE',  ( 74.67462176122349149, -68.26729679194136224, 247.0134555675329864 ) ) ;
#17665=ORIENTED_EDGE ( 'NONE', *, *, #9983, .T. ) ;
#17681=CARTESIAN_POINT ( 'NONE',  ( 107.0667036193247696, -67.87844715994094713, 90.21780599115064092 ) ) ;
#17698=EDGE_LOOP ( 'NONE', ( #32069, #70301, #73547, #29112, #75800 ) ) ;
#17716=ADVANCED_FACE ( 'NONE', ( #30959 ), #16005, .F. ) ;
#17725=CARTESIAN_POINT ( 'NONE',  ( 107.0667039024470313, -104.2784471599420755, -19.78219314458201694 ) ) ;
#17767=CARTESIAN_POINT ( 'NONE',  ( 82.56670390244703128, -104.2784471599409670, 24.21780685541800082 ) ) ;
#17795=ORIENTED_EDGE ( 'NONE', *, *, #83860, .F. ) ;
#17803=VERTEX_POINT ( 'NONE', #18669 ) ;
#17814=CARTESIAN_POINT ( 'NONE',  ( 68.96386331618904819, -139.0368364878925718, 246.8410557163890076 ) ) ;
#17820=FACE_BOUND ( 'NONE', #72094, .T. ) ;
#17828=AXIS2_PLACEMENT_3D ( 'NONE', #50306, #1738, #55319 ) ;
#17832=VECTOR ( 'NONE', #12454, 1000.000000000000000 ) ;
#17836=CARTESIAN_POINT ( 'NONE',  ( 107.0667039024470313, -104.2784471599409528, 25.71780685541800437 ) ) ;
#17838=DIRECTION ( 'NONE',  ( -1.000000000000000000, -8.163404592832032979E-16, 0.000000000000000000 ) ) ;
#17847=ADVANCED_FACE ( 'NONE', ( #11863 ), #39556, .F. ) ;
#17853=CARTESIAN_POINT ( 'NONE',  ( 59.56670390244700997, -79.67844715994098692, 85.21780685541799016 ) ) ;
#17855=EDGE_CURVE ( 'NONE', #52976, #14490, #54052, .T. ) ;
#17863=VERTEX_POINT ( 'NONE', #46798 ) ;
#17864=CARTESIAN_POINT ( 'NONE',  ( 110.4543776057972053, -75.92700761993931735, 250.2201230397200220 ) ) ;
#17865=CARTESIAN_POINT ( 'NONE',  ( 146.4725015627529103, -68.45085798094062568, 246.9176224039437386 ) ) ;
#17867=CARTESIAN_POINT ( 'NONE',  ( 92.81932083335591699, -95.00417761012948858, -11.78219314458228695 ) ) ;
#17875=ORIENTED_EDGE ( 'NONE', *, *, #37377, .T. ) ;
#17913=CARTESIAN_POINT ( 'NONE',  ( 127.0667052882549797, -71.37844715994091871, 55.21780685541800437 ) ) ;
#17920=CARTESIAN_POINT ( 'NONE',  ( 67.90006995966258785, -137.2348498917707218, 247.1319224459439852 ) ) ;
#17922=CARTESIAN_POINT ( 'NONE',  ( 90.06670420047026937, -131.9777253117771636, 55.21780685541800437 ) ) ;
#17935=LINE ( 'NONE', #66530, #32489 ) ;
#17938=EDGE_LOOP ( 'NONE', ( #78958, #17505, #66065, #56078, #48089, #39248, #24614, #31806, #20654, #31676, #4538, #69752 ) ) ;
#17945=CARTESIAN_POINT ( 'NONE',  ( 144.0667039024470739, -137.6784471599409017, 55.21780685541800437 ) ) ;
#17953=DIRECTION ( 'NONE',  ( -0.5000000000000069944, 0.8660254037844344888, -2.684678751731748934E-14 ) ) ;
#17968=CARTESIAN_POINT ( 'NONE',  ( 80.80881079632693798, -95.93364041391161834, 250.2178068554180470 ) ) ;
#17973=LINE ( 'NONE', #59745, #56149 ) ;
#17985=CARTESIAN_POINT ( 'NONE',  ( 122.2221484686747743, -98.95301919085950715, -21.02845593540943270 ) ) ;
#17998=DIRECTION ( 'NONE',  ( -3.100000000000000258E-29, 3.100000000000000044E-14, 1.000000000000000000 ) ) ;
#18018=FACE_OUTER_BOUND ( 'NONE', #67178, .T. ) ;
#18043=AXIS2_PLACEMENT_3D ( 'NONE', #21008, #26922, #13744 ) ;
#18050=ORIENTED_EDGE ( 'NONE', *, *, #58987, .F. ) ;
#18051=CARTESIAN_POINT ( 'NONE',  ( 107.0667039024470313, -104.2784471599409528, 55.21780685541800437 ) ) ;
#18053=DIRECTION ( 'NONE',  ( 1.000000000000000000, 1.000000000000000078E-15, 0.000000000000000000 ) ) ;
#18054=CARTESIAN_POINT ( 'NONE',  ( 144.0637627337163735, -140.6784471599286235, 245.5331643397809671 ) ) ;
#18079=ORIENTED_EDGE ( 'NONE', *, *, #22138, .F. ) ;
#18080=FACE_BOUND ( 'NONE', #69293, .T. ) ;
#18095=ADVANCED_FACE ( 'NONE', ( #70870 ), #4540, .F. ) ;
#18104=EDGE_LOOP ( 'NONE', ( #54063, #62998, #16847, #11360, #10470, #70484 ) ) ;
#18116=LINE ( 'NONE', #73980, #23568 ) ;
#18121=CARTESIAN_POINT ( 'NONE',  ( 78.56670390244704549, -118.2784471599409812, 45.21780685541799727 ) ) ;
#18134=ORIENTED_EDGE ( 'NONE', *, *, #61640, .F. ) ;
#18142=ORIENTED_EDGE ( 'NONE', *, *, #87828, .F. ) ;
#18148=EDGE_LOOP ( 'NONE', ( #42222, #83624, #41113, #5619 ) ) ;
#18154=ORIENTED_EDGE ( 'NONE', *, *, #75028, .F. ) ;
#18160=DIRECTION ( 'NONE',  ( 1.000000000000000000, 1.000000000000000078E-15, 0.000000000000000000 ) ) ;
#18165=VECTOR ( 'NONE', #32346, 1000.000000000000000 ) ;
#18216=ORIENTED_EDGE ( 'NONE', *, *, #30299, .F. ) ;
#18229=VERTEX_POINT ( 'NONE', #40788 ) ;
#18230=AXIS2_PLACEMENT_3D ( 'NONE', #25004, #5004, #45420 ) ;
#18245=DIRECTION ( 'NONE',  ( 1.000000000000000000, 1.132880637372608296E-15, 0.000000000000000000 ) ) ;
#18263=EDGE_CURVE ( 'NONE', #20018, #61103, #31644, .T. ) ;
#18276=VERTEX_POINT ( 'NONE', #7181 ) ;
#18281=CARTESIAN_POINT ( 'NONE',  ( 108.0015324895207129, -121.2375264746780488, -19.21046202161247152 ) ) ;
#18296=DIRECTION ( 'NONE',  ( -3.100000000000000258E-29, 3.100000000000000044E-14, 1.000000000000000000 ) ) ;
#18308=LINE ( 'NONE', #51044, #76399 ) ;
#18309=CARTESIAN_POINT ( 'NONE',  ( 147.0048854145641144, -67.93494677174348340, 245.9788996868301751 ) ) ;
#18311=CARTESIAN_POINT ( 'NONE',  ( 100.6318841171118379, -87.59835267194286246, -9.274842254011147702 ) ) ;
#18348=AXIS2_PLACEMENT_3D ( 'NONE', #85766, #23973, #55877 ) ;
#18351=AXIS2_PLACEMENT_3D ( 'NONE', #80665, #11620, #87472 ) ;
#18357=DIRECTION ( 'NONE',  ( 1.000000000000000000, 1.000000000000000078E-15, 0.000000000000000000 ) ) ;
#18359=DIRECTION ( 'NONE',  ( 1.000000000000000000, 0.000000000000000000, 0.000000000000000000 ) ) ;
#18368=ORIENTED_EDGE ( 'NONE', *, *, #45683, .T. ) ;
#18379=LINE ( 'NONE', #11586, #35511 ) ;
#18389=CARTESIAN_POINT ( 'NONE',  ( 91.91125933621933086, -101.0284471599423739, -21.78219314458213063 ) ) ;
#18397=VERTEX_POINT ( 'NONE', #78474 ) ;
#18402=PLANE ( 'NONE',  #17572 ) ;
#18419=VECTOR ( 'NONE', #63116, 1000.000000000000000 ) ;
#18425=DIRECTION ( 'NONE',  ( 1.000000000000000078E-15, -1.000000000000000000, 0.000000000000000000 ) ) ;
#18430=DIRECTION ( 'NONE',  ( -3.100000000000000258E-29, 3.100000000000000044E-14, 1.000000000000000000 ) ) ;
#18452=ORIENTED_EDGE ( 'NONE', *, *, #45751, .F. ) ;
#18462=ADVANCED_FACE ( 'NONE', ( #85291 ), #42560, .T. ) ;
#18481=CARTESIAN_POINT ( 'NONE',  ( 144.0667052733537901, -83.77844715994089597, 55.21780685541800437 ) ) ;
#18490=ORIENTED_EDGE ( 'NONE', *, *, #42090, .F. ) ;
#18496=LINE ( 'NONE', #80743, #73026 ) ;
#18502=CARTESIAN_POINT ( 'NONE',  ( 69.38289674479436542, -139.5561639417483946, 246.9828236755479907 ) ) ;
#18513=CARTESIAN_POINT ( 'NONE',  ( 122.2221484686747317, -96.64604508066639710, -19.23816774842027044 ) ) ;
#18536=EDGE_CURVE ( 'NONE', #65691, #60056, #39343, .T. ) ;
#18542=FACE_OUTER_BOUND ( 'NONE', #4420, .T. ) ;
#18545=ORIENTED_EDGE ( 'NONE', *, *, #80377, .T. ) ;
#18548=ORIENTED_EDGE ( 'NONE', *, *, #31423, .F. ) ;
#18596=AXIS2_PLACEMENT_3D ( 'NONE', #51127, #78867, #81551 ) ;
#18600=EDGE_CURVE ( 'NONE', #67104, #37337, #77436, .T. ) ;
#18622=EDGE_CURVE ( 'NONE', #67362, #61554, #86168, .T. ) ;
#18626=AXIS2_PLACEMENT_3D ( 'NONE', #30059, #57754, #45002 ) ;
#18634=CYLINDRICAL_SURFACE ( 'NONE', #22594, 3.500000000000003109 ) ;
#18644=ORIENTED_EDGE ( 'NONE', *, *, #53180, .T. ) ;
#18657=EDGE_CURVE ( 'NONE', #17073, #22233, #78098, .T. ) ;
#18660=CYLINDRICAL_SURFACE ( 'NONE', #10838, 4.500000000000003553 ) ;
#18664=ORIENTED_EDGE ( 'NONE', *, *, #17367, .F. ) ;
#18666=VERTEX_POINT ( 'NONE', #59770 ) ;
#18669=CARTESIAN_POINT ( 'NONE',  ( 103.3797721312301547, -105.8297479413476196, 2.217806855418058554 ) ) ;
#18684=DIRECTION ( 'NONE',  ( 3.100000000000000258E-29, -3.100000000000000044E-14, -1.000000000000000000 ) ) ;
#18693=AXIS2_PLACEMENT_3D ( 'NONE', #36530, #64230, #2001 ) ;
#18694=FACE_OUTER_BOUND ( 'NONE', #10293, .T. ) ;
#18714=CARTESIAN_POINT ( 'NONE',  ( 145.8009859422575119, -77.83856765075479700, 247.4449540823549967 ) ) ;
#18736=EDGE_CURVE ( 'NONE', #34428, #37855, #82049, .T. ) ;
#18738=CARTESIAN_POINT ( 'NONE',  ( 107.0667039024470313, -104.2784471599420755, -19.78219314458201694 ) ) ;
#18740=ORIENTED_EDGE ( 'NONE', *, *, #21390, .T. ) ;
#18752=CARTESIAN_POINT ( 'NONE',  ( 120.2221484686747317, -111.8737466215628871, -21.78219314458179667 ) ) ;
#18779=CARTESIAN_POINT ( 'NONE',  ( 127.0667052882550365, -78.66107132697010229, 222.2178068554179902 ) ) ;
#18786=ORIENTED_EDGE ( 'NONE', *, *, #13023, .F. ) ;
#18816=ADVANCED_FACE ( 'NONE', ( #85186 ), #14341, .F. ) ;
#18825=ORIENTED_EDGE ( 'NONE', *, *, #41989, .F. ) ;
#18827=DIRECTION ( 'NONE',  ( 3.100000000000000258E-29, -3.100000000000000044E-14, -1.000000000000000000 ) ) ;
#18842=EDGE_CURVE ( 'NONE', #65875, #11800, #37014, .T. ) ;
#18851=LINE ( 'NONE', #26555, #4132 ) ;
#18866=CARTESIAN_POINT ( 'NONE',  ( 107.0667039024470313, -104.2784471599409528, 24.21780685541800082 ) ) ;
#18879=ORIENTED_EDGE ( 'NONE', *, *, #47208, .F. ) ;
#18880=CIRCLE ( 'NONE', #36269, 24.50000000000000711 ) ;
#18890=DIRECTION ( 'NONE',  ( 1.000000000000000000, 9.408669700213195533E-16, 0.000000000000000000 ) ) ;
#18902=DIRECTION ( 'NONE',  ( 0.5000000000000015543, 0.8660254037844377084, -2.602085213965216006E-14 ) ) ;
#18907=ORIENTED_EDGE ( 'NONE', *, *, #74700, .F. ) ;
#18925=CARTESIAN_POINT ( 'NONE',  ( 116.3167039024470029, -67.87844715994093292, 55.21780685541800437 ) ) ;
#18937=EDGE_CURVE ( 'NONE', #15221, #2107, #51068, .T. ) ;
#18954=DIRECTION ( 'NONE',  ( -1.000000000000000000, 0.000000000000000000, 0.000000000000000000 ) ) ;
#18959=DIRECTION ( 'NONE',  ( -3.100000000000000258E-29, 3.100000000000000044E-14, 1.000000000000000000 ) ) ;
#18981=AXIS2_PLACEMENT_3D ( 'NONE', #45019, #65037, #23720 ) ;
#18999=CARTESIAN_POINT ( 'NONE',  ( 71.06670390244701707, -90.27844715994098124, 51.21780685541800437 ) ) ;
#19032=PLANE ( 'NONE',  #81542 ) ;
#19038=EDGE_CURVE ( 'NONE', #68139, #41462, #71392, .T. ) ;
#19062=PLANE ( 'NONE',  #87967 ) ;
#19067=LINE ( 'NONE', #27220, #56340 ) ;
#19078=DIRECTION ( 'NONE',  ( 1.000000000000000078E-15, -1.000000000000000000, 0.000000000000000000 ) ) ;
#19094=ORIENTED_EDGE ( 'NONE', *, *, #38245, .F. ) ;
#19100=DIRECTION ( 'NONE',  ( -0.5000000000000012212, 0.8660254037844379305, -2.684678751731759663E-14 ) ) ;
#19123=CARTESIAN_POINT ( 'NONE',  ( 90.06670420047024095, -102.7784471599409670, 55.21780685541800437 ) ) ;
#19137=FACE_OUTER_BOUND ( 'NONE', #35719, .T. ) ;
#19140=DIRECTION ( 'NONE',  ( 0.8660254037844389297, -0.4999999999999993894, 1.550000000000000968E-14 ) ) ;
#19152=AXIS2_PLACEMENT_3D ( 'NONE', #72077, #85719, #8966 ) ;
#19155=CARTESIAN_POINT ( 'NONE',  ( 133.3464018318852595, -128.1369193926091157, 249.3173333679100097 ) ) ;
#19156=LINE ( 'NONE', #12797, #8392 ) ;
#19176=VECTOR ( 'NONE', #78066, 1000.000000000000000 ) ;
#19181=CARTESIAN_POINT ( 'NONE',  ( 133.3763347640258417, -80.31065270615032148, 249.3055338466990065 ) ) ;
#19182=ORIENTED_EDGE ( 'NONE', *, *, #40334, .T. ) ;
#19189=CARTESIAN_POINT ( 'NONE',  ( 67.06670390244707392, -140.6784471599409869, 247.2178068554179902 ) ) ;
#19212=ORIENTED_EDGE ( 'NONE', *, *, #73254, .F. ) ;
#19237=CARTESIAN_POINT ( 'NONE',  ( 121.3178890780284434, -113.5468731908974291, -21.78219314458173983 ) ) ;
#19238=ORIENTED_EDGE ( 'NONE', *, *, #88478, .F. ) ;
#19243=ORIENTED_EDGE ( 'NONE', *, *, #63985, .T. ) ;
#19252=CARTESIAN_POINT ( 'NONE',  ( 140.0667039024470455, -118.2784471599408960, 51.21780685541800437 ) ) ;
#19265=DIRECTION ( 'NONE',  ( 0.000000000000000000, 0.000000000000000000, 1.000000000000000000 ) ) ;
#19290=DIRECTION ( 'NONE',  ( 1.000000000000000000, 0.000000000000000000, 0.000000000000000000 ) ) ;
#19328=EDGE_CURVE ( 'NONE', #36508, #24432, #64507, .T. ) ;
#19334=ADVANCED_FACE ( 'NONE', ( #51739 ), #50411, .T. ) ;
#19372=CARTESIAN_POINT ( 'NONE',  ( 123.4403675665762705, -98.97427844173840583, -10.56397404668093998 ) ) ;
#19397=ORIENTED_EDGE ( 'NONE', *, *, #58122, .F. ) ;
#19407=ORIENTED_EDGE ( 'NONE', *, *, #922, .T. ) ;
#19440=EDGE_CURVE ( 'NONE', #23818, #24431, #67621, .T. ) ;
#19444=DIRECTION ( 'NONE',  ( -4.440892098500319985E-16, -3.100000000000000044E-14, -1.000000000000000000 ) ) ;
#19453=EDGE_CURVE ( 'NONE', #34012, #42178, #70990, .T. ) ;
#19467=FACE_OUTER_BOUND ( 'NONE', #34851, .T. ) ;
#19483=VERTEX_POINT ( 'NONE', #4951 ) ;
#19501=ORIENTED_EDGE ( 'NONE', *, *, #20765, .T. ) ;
#19523=CARTESIAN_POINT ( 'NONE',  ( 110.0667047667142953, -67.87844715994094713, 93.21780685541800437 ) ) ;
#19525=VERTEX_POINT ( 'NONE', #45809 ) ;
#19530=CONICAL_SURFACE ( 'NONE', #64482, 16.25000000000000000, 0.5235987755982992597 ) ;
#19534=ORIENTED_EDGE ( 'NONE', *, *, #71378, .F. ) ;
#19538=ORIENTED_EDGE ( 'NONE', *, *, #18937, .T. ) ;
#19570=ORIENTED_EDGE ( 'NONE', *, *, #29193, .F. ) ;
#19602=CARTESIAN_POINT ( 'NONE',  ( 107.0667039024470313, -104.2784471599420755, -19.78219314458201694 ) ) ;
#19618=CIRCLE ( 'NONE', #82022, 3.000000864267354572 ) ;
#19629=EDGE_CURVE ( 'NONE', #43244, #79697, #68525, .T. ) ;
#19652=ORIENTED_EDGE ( 'NONE', *, *, #63569, .F. ) ;
#19654=CARTESIAN_POINT ( 'NONE',  ( 107.0667039024470313, -104.2784471599421323, -21.78219314458201694 ) ) ;
#19667=ADVANCED_FACE ( 'NONE', ( #27182 ), #60776, .T. ) ;
#19694=DIRECTION ( 'NONE',  ( 0.000000000000000000, 0.000000000000000000, 1.000000000000000000 ) ) ;
#19710=CARTESIAN_POINT ( 'NONE',  ( 92.84712468462734591, -113.5675721218997865, -19.21046202161272376 ) ) ;
#19711=DIRECTION ( 'NONE',  ( -3.100000000000000258E-29, 3.100000000000000044E-14, 1.000000000000000000 ) ) ;
#19731=EDGE_CURVE ( 'NONE', #25758, #54218, #82621, .T. ) ;
#19738=DIRECTION ( 'NONE',  ( -0.7396053187813123042, -0.6730408400909958511, 0.000000000000000000 ) ) ;
#19746=PLANE ( 'NONE',  #28791 ) ;
#19754=EDGE_CURVE ( 'NONE', #56065, #87130, #30327, .T. ) ;
#19755=CARTESIAN_POINT ( 'NONE',  ( 145.4513818679876920, -123.8420284488499306, 247.5435765132629626 ) ) ;
#19766=ORIENTED_EDGE ( 'NONE', *, *, #16581, .T. ) ;
#19767=ORIENTED_EDGE ( 'NONE', *, *, #49788, .F. ) ;
#19769=ORIENTED_EDGE ( 'NONE', *, *, #50297, .T. ) ;
#19789=AXIS2_PLACEMENT_3D ( 'NONE', #11386, #4122, #39080 ) ;
#19796=ORIENTED_EDGE ( 'NONE', *, *, #53717, .T. ) ;
#19802=B_SPLINE_SURFACE_WITH_KNOTS ( 'NONE', 3, 3, ( 
 ( #33674, #39580, #19155, #40925 ),
 ( #89093, #54531, #46828, #75468 ),
 ( #67286, #13238, #68648, #6414 ),
 ( #34106, #61812, #75908, #13676 ),
 ( #4627, #74556, #40029, #32311 ),
 ( #62268, #72116, #3077, #35006 ),
 ( #41808, #51648, #21398, #79391 ) ),
 .UNSPECIFIED., .F., .F., .F.,
 ( 4, 1, 1, 1, 4 ),
 ( 4, 4 ),
 ( -0.0008599663877943859985, 0.2857142857142860315, 0.5714285714285709528, 0.8571428571428569843, 1.000859966387789957 ),
 ( 0.09780657971653439198, 1.000859966387789957 ),
 .UNSPECIFIED. ) ;
#19811=DIRECTION ( 'NONE',  ( 0.000000000000000000, 0.000000000000000000, 1.000000000000000000 ) ) ;
#19818=LINE ( 'NONE', #20277, #46434 ) ;
#19851=CARTESIAN_POINT ( 'NONE',  ( 129.9817983987124705, -140.4109954690793245, 246.9195128019829895 ) ) ;
#19869=EDGE_CURVE ( 'NONE', #87491, #1864, #2298, .T. ) ;
#19890=CARTESIAN_POINT ( 'NONE',  ( 99.08946256649485917, -109.4614598618336174, 2.217806855418169576 ) ) ;
#19896=AXIS2_PLACEMENT_3D ( 'NONE', #83735, #41921, #77817 ) ;
#19903=DIRECTION ( 'NONE',  ( 0.4999999999999989453, 0.8660254037844392627, -2.684678751731760294E-14 ) ) ;
#19904=ORIENTED_EDGE ( 'NONE', *, *, #64878, .F. ) ;
#19914=CIRCLE ( 'NONE', #64855, 29.49999999999998579 ) ;
#19925=AXIS2_PLACEMENT_3D ( 'NONE', #49251, #62447, #20229 ) ;
#19931=LINE ( 'NONE', #74895, #30627 ) ;
#19935=EDGE_LOOP ( 'NONE', ( #51596, #56197, #56446, #87269 ) ) ;
#19949=FACE_OUTER_BOUND ( 'NONE', #62014, .T. ) ;
#19973=EDGE_CURVE ( 'NONE', #42178, #36122, #25281, .T. ) ;
#19974=CARTESIAN_POINT ( 'NONE',  ( 147.0667039024469886, -67.87844715994090450, 222.2178068554179902 ) ) ;
#19978=CARTESIAN_POINT ( 'NONE',  ( 69.95705417202927379, -138.0482284146212635, 247.6588381008699855 ) ) ;
#19982=AXIS2_PLACEMENT_3D ( 'NONE', #28744, #47029, #61128 ) ;
#20007=AXIS2_PLACEMENT_3D ( 'NONE', #38241, #80946, #18245 ) ;
#20018=VERTEX_POINT ( 'NONE', #11668 ) ;
#20019=ORIENTED_EDGE ( 'NONE', *, *, #5285, .F. ) ;
#20027=ORIENTED_EDGE ( 'NONE', *, *, #48704, .T. ) ;
#20031=ORIENTED_EDGE ( 'NONE', *, *, #46827, .F. ) ;
#20036=ORIENTED_EDGE ( 'NONE', *, *, #30363, .F. ) ;
#20038=CARTESIAN_POINT ( 'NONE',  ( 67.06670390244704549, -104.2784471599409812, 234.7178068554179902 ) ) ;
#20044=CARTESIAN_POINT ( 'NONE',  ( 107.5667039024470313, -102.2941336766436251, -19.78219314458207378 ) ) ;
#20060=CARTESIAN_POINT ( 'NONE',  ( 99.08946256649485917, -109.4614598618343138, -19.78219314458184996 ) ) ;
#20063=EDGE_LOOP ( 'NONE', ( #67385, #68428, #18664, #71091 ) ) ;
#20077=DIRECTION ( 'NONE',  ( 1.000000000000000000, 0.000000000000000000, 0.000000000000000000 ) ) ;
#20092=CARTESIAN_POINT ( 'NONE',  ( 74.19170390244705970, -127.9034471599409812, 45.21780685541799727 ) ) ;
#20113=DIRECTION ( 'NONE',  ( 0.000000000000000000, 0.000000000000000000, 1.000000000000000000 ) ) ;
#20120=VECTOR ( 'NONE', #67807, 1000.000000000000114 ) ;
#20131=AXIS2_PLACEMENT_3D ( 'NONE', #29938, #16746, #58071 ) ;
#20140=EDGE_CURVE ( 'NONE', #85724, #78112, #13452, .T. ) ;
#20149=LINE ( 'NONE', #81050, #65000 ) ;
#20155=VERTEX_POINT ( 'NONE', #48384 ) ;
#20195=VECTOR ( 'NONE', #40890, 1000.000000000000000 ) ;
#20219=DIRECTION ( 'NONE',  ( -1.000000000000000000, -1.181088324069315053E-15, 0.000000000000000000 ) ) ;
#20229=DIRECTION ( 'NONE',  ( -1.000000000000000000, -1.541976423090496028E-15, 0.000000000000000000 ) ) ;
#20264=EDGE_CURVE ( 'NONE', #69134, #34414, #19818, .T. ) ;
#20270=EDGE_CURVE ( 'NONE', #56526, #13876, #65344, .T. ) ;
#20277=CARTESIAN_POINT ( 'NONE',  ( 99.08946256649487339, -99.09543445804918349, 2.217806855417836509 ) ) ;
#20283=DIRECTION ( 'NONE',  ( 1.000000000000000078E-15, -1.000000000000000000, 0.000000000000000000 ) ) ;
#20333=FACE_OUTER_BOUND ( 'NONE', #18148, .T. ) ;
#20343=FACE_OUTER_BOUND ( 'NONE', #62895, .T. ) ;
#20346=VERTEX_POINT ( 'NONE', #16150 ) ;
#20347=CARTESIAN_POINT ( 'NONE',  ( 145.2378574334098005, -69.54310811732223385, 247.4968681563179871 ) ) ;
#20353=EDGE_LOOP ( 'NONE', ( #35288, #87052, #24323, #67711 ) ) ;
#20355=VERTEX_POINT ( 'NONE', #57910 ) ;
#20357=EDGE_CURVE ( 'NONE', #3053, #36009, #10156, .T. ) ;
#20358=EDGE_CURVE ( 'NONE', #54044, #71630, #44267, .T. ) ;
#20369=VERTEX_POINT ( 'NONE', #24732 ) ;
#20370=CARTESIAN_POINT ( 'NONE',  ( 90.06670390244703128, -104.2784471599414644, 0.2178068554180012661 ) ) ;
#20380=DIRECTION ( 'NONE',  ( -1.000000000000000000, 0.000000000000000000, 0.000000000000000000 ) ) ;
#20397=EDGE_CURVE ( 'NONE', #62972, #47787, #41, .T. ) ;
#20406=ORIENTED_EDGE ( 'NONE', *, *, #84582, .F. ) ;
#20418=DIRECTION ( 'NONE',  ( -3.100000000000000258E-29, 3.100000000000000044E-14, 1.000000000000000000 ) ) ;
#20428=CIRCLE ( 'NONE', #50699, 7.999999999999992895 ) ;
#20471=AXIS2_PLACEMENT_3D ( 'NONE', #70467, #49544, #28671 ) ;
#20476=CARTESIAN_POINT ( 'NONE',  ( 132.2857443282839824, -83.77844715994092439, 45.21780685541799727 ) ) ;
#20491=VERTEX_POINT ( 'NONE', #86971 ) ;
#20505=VECTOR ( 'NONE', #77409, 1000.000000000000000 ) ;
#20518=CARTESIAN_POINT ( 'NONE',  ( 68.70120400217622603, -127.1654454912769836, 247.5297809874748793 ) ) ;
#20531=CARTESIAN_POINT ( 'NONE',  ( 142.4374377537056660, -108.6105248799684233, 248.3919668373590071 ) ) ;
#20532=ORIENTED_EDGE ( 'NONE', *, *, #11625, .T. ) ;
#20542=CARTESIAN_POINT ( 'NONE',  ( 68.24270753389627941, -138.8544507913902066, 245.5998607319569942 ) ) ;
#20561=ORIENTED_EDGE ( 'NONE', *, *, #36965, .T. ) ;
#20583=DIRECTION ( 'NONE',  ( -1.000000000000000078E-15, 1.000000000000000000, 0.000000000000000000 ) ) ;
#20591=ORIENTED_EDGE ( 'NONE', *, *, #45770, .F. ) ;
#20608=CARTESIAN_POINT ( 'NONE',  ( 124.0667039024470313, -104.2784471599417202, 0.2178068554180012661 ) ) ;
#20632=CIRCLE ( 'NONE', #34936, 11.49999999999999645 ) ;
#20639=MANIFOLD_SOLID_BREP ( 'Stock-Rail and drilling-1', #21310 ) ;
#20654=ORIENTED_EDGE ( 'NONE', *, *, #26154, .F. ) ;
#20660=LINE ( 'NONE', #89712, #15544 ) ;
#20663=CARTESIAN_POINT ( 'NONE',  ( 67.09903452484594766, -67.90769682686300257, 245.8492538885293186 ) ) ;
#20671=CARTESIAN_POINT ( 'NONE',  ( 118.5667039024470313, -104.2784471599411376, 19.21780685541799016 ) ) ;
#20704=CARTESIAN_POINT ( 'NONE',  ( 107.0667039024470313, -104.2784471599418197, -11.78219314458200984 ) ) ;
#20706=ORIENTED_EDGE ( 'NONE', *, *, #50808, .F. ) ;
#20728=ORIENTED_EDGE ( 'NONE', *, *, #44628, .F. ) ;
#20748=CARTESIAN_POINT ( 'NONE',  ( 145.4217101158483842, -139.2854844008623445, 245.9863971430950187 ) ) ;
#20754=ORIENTED_EDGE ( 'NONE', *, *, #29707, .T. ) ;
#20758=DIRECTION ( 'NONE',  ( 1.000000000000000078E-15, -1.000000000000000000, 0.000000000000000000 ) ) ;
#20760=DIRECTION ( 'NONE',  ( 1.000000000000000000, 0.000000000000000000, 0.000000000000000000 ) ) ;
#20765=EDGE_CURVE ( 'NONE', #33950, #17073, #23341, .T. ) ;
#20782=PLANE ( 'NONE',  #58554 ) ;
#20784=ORIENTED_EDGE ( 'NONE', *, *, #80759, .F. ) ;
#20787=EDGE_CURVE ( 'NONE', #81489, #24432, #70855, .T. ) ;
#20795=FACE_OUTER_BOUND ( 'NONE', #26395, .T. ) ;
#20796=ORIENTED_EDGE ( 'NONE', *, *, #36586, .F. ) ;
#20803=EDGE_CURVE ( 'NONE', #65259, #69797, #7714, .T. ) ;
#20814=AXIS2_PLACEMENT_3D ( 'NONE', #12568, #38913, #73439 ) ;
#20829=FACE_OUTER_BOUND ( 'NONE', #70398, .T. ) ;
#20835=EDGE_LOOP ( 'NONE', ( #38625, #83523, #59184, #79105 ) ) ;
#20838=CARTESIAN_POINT ( 'NONE',  ( 70.88111044991026688, -139.0101909505960691, 247.5112285516309782 ) ) ;
#20846=ORIENTED_EDGE ( 'NONE', *, *, #83155, .T. ) ;
#20853=CARTESIAN_POINT ( 'NONE',  ( 147.0667039024469886, -67.87844715994090450, 222.2178068554179902 ) ) ;
#20873=EDGE_CURVE ( 'NONE', #40469, #13431, #44002, .T. ) ;
#20889=EDGE_LOOP ( 'NONE', ( #25129, #42965, #21541, #52933 ) ) ;
#20893=EDGE_CURVE ( 'NONE', #71132, #64360, #23842, .T. ) ;
#20900=EDGE_CURVE ( 'NONE', #70808, #11319, #78123, .T. ) ;
#20905=EDGE_LOOP ( 'NONE', ( #71215, #52244, #63093, #24713 ) ) ;
#20911=EDGE_LOOP ( 'NONE', ( #38548, #39768, #27936 ) ) ;
#20940=ORIENTED_EDGE ( 'NONE', *, *, #36965, .F. ) ;
#20943=CARTESIAN_POINT ( 'NONE',  ( 67.06670390244700286, -67.87641945813885513, 245.9001325644979659 ) ) ;
#20963=EDGE_CURVE ( 'NONE', #75262, #25396, #62459, .T. ) ;
#20969=CARTESIAN_POINT ( 'NONE',  ( 67.06673837846007302, -137.6758525980020806, 245.5072637273240161 ) ) ;
#20974=EDGE_LOOP ( 'NONE', ( #41322, #18545, #1289, #74943 ) ) ;
#20981=CARTESIAN_POINT ( 'NONE',  ( 92.53858863555680614, -80.85146542362646471, 250.2178068554180470 ) ) ;
#20997=CARTESIAN_POINT ( 'NONE',  ( 107.0667039024470313, -104.2784471599409528, 25.71780685541800437 ) ) ;
#21008=CARTESIAN_POINT ( 'NONE',  ( 107.0667039024470313, -119.4690460831836276, -21.78219314458154798 ) ) ;
#21027=CIRCLE ( 'NONE', #84850, 2.000000000000007550 ) ;
#21044=CARTESIAN_POINT ( 'NONE',  ( 92.91125933621933086, -94.95109689075242443, -19.26696060647628528 ) ) ;
#21045=CARTESIAN_POINT ( 'NONE',  ( 70.06968321367156705, -140.6784088069870222, 245.5331728854790185 ) ) ;
#21046=VECTOR ( 'NONE', #75495, 1000.000000000000000 ) ;
#21053=DIRECTION ( 'NONE',  ( -1.000000000000000000, 0.000000000000000000, 0.000000000000000000 ) ) ;
#21061=PLANE ( 'NONE',  #60010 ) ;
#21065=DIRECTION ( 'NONE',  ( 1.000000000000000078E-15, -1.000000000000000000, 0.000000000000000000 ) ) ;
#21083=CARTESIAN_POINT ( 'NONE',  ( 91.91125933621933086, -96.68314769832132072, -19.26696060647622843 ) ) ;
#21085=DIRECTION ( 'NONE',  ( -3.100000000000000258E-29, 3.100000000000000044E-14, 1.000000000000000000 ) ) ;
#21089=CARTESIAN_POINT ( 'NONE',  ( 70.96339109104607701, -139.0938916433960912, 247.5000110694289788 ) ) ;
#21095=VERTEX_POINT ( 'NONE', #35190 ) ;
#21098=AXIS2_PLACEMENT_3D ( 'NONE', #18738, #39179, #73706 ) ;
#21101=AXIS2_PLACEMENT_3D ( 'NONE', #15171, #1990, #35599 ) ;
#21102=DIRECTION ( 'NONE',  ( -9.437404618277395057E-08, 0.000000000000000000, -0.9999999999999955591 ) ) ;
#21105=PLANE ( 'NONE',  #81102 ) ;
#21106=CARTESIAN_POINT ( 'NONE',  ( 70.56670390244700286, -67.87844715994098976, 222.2178068554179902 ) ) ;
#21111=CARTESIAN_POINT ( 'NONE',  ( 67.84300328633237598, -68.62291849891890649, 247.0791910793475381 ) ) ;
#21118=CARTESIAN_POINT ( 'NONE',  ( 145.6879805935534478, -69.19066990707743514, 247.4001512595007739 ) ) ;
#21119=DIRECTION ( 'NONE',  ( -3.100000000000000258E-29, 3.100000000000000044E-14, 1.000000000000000000 ) ) ;
#21127=ORIENTED_EDGE ( 'NONE', *, *, #31423, .T. ) ;
#21140=ORIENTED_EDGE ( 'NONE', *, *, #63109, .T. ) ;
#21157=ORIENTED_EDGE ( 'NONE', *, *, #53457, .T. ) ;
#21158=ORIENTED_EDGE ( 'NONE', *, *, #24792, .F. ) ;
#21162=EDGE_CURVE ( 'NONE', #61542, #63618, #40108, .T. ) ;
#21176=B_SPLINE_CURVE_WITH_KNOTS ( 'NONE', 3,
 ( #67950, #87953, #47931, #75671 ),
 .UNSPECIFIED., .F., .F.,
 ( 4, 4 ),
 ( -0.6035999334370389935, -0.5903216970416030884 ),
 .UNSPECIFIED. ) ;
#21178=CARTESIAN_POINT ( 'NONE',  ( 91.91441891875214765, -111.9861225405538505, -11.78219314458175937 ) ) ;
#21201=CARTESIAN_POINT ( 'NONE',  ( 107.0667039024470313, -104.2784471599413791, 2.217806855418003043 ) ) ;
#21203=FACE_OUTER_BOUND ( 'NONE', #6442, .T. ) ;
#21249=EDGE_CURVE ( 'NONE', #7062, #38828, #8875, .T. ) ;
#21255=DIRECTION ( 'NONE',  ( -3.100000000000000258E-29, 3.100000000000000044E-14, 1.000000000000000000 ) ) ;
#21267=CARTESIAN_POINT ( 'NONE',  ( 77.61670390244702844, -103.2284471599409841, 222.2178068554179902 ) ) ;
#21287=VECTOR ( 'NONE', #31504, 1000.000000000000000 ) ;
#21290=LINE ( 'NONE', #9019, #19176 ) ;
#21291=ORIENTED_EDGE ( 'NONE', *, *, #50205, .T. ) ;
#21292=AXIS2_PLACEMENT_3D ( 'NONE', #31994, #3412, #52844 ) ;
#21302=EDGE_CURVE ( 'NONE', #44089, #4100, #14634, .T. ) ;
#21310=CLOSED_SHELL ( 'NONE', ( #62528, #16625, #46388, #49679, #26784, #65133, #28374, #8925, #8821, #57060, #56557, #12619, #87231, #55910, #15973, #77797, #60844, #26322, #74973, #80867, #166, #45363, #79765, #86219, #33513, #49715, #83428, #67112, #13417, #25822, #88826, #62442, #50114, #61870, #23559, #36703, #28665, #10064, #84486, #59842, #73894, #42376, #58587, #18095, #53777, #42535, #82466, #51897, #17100, #39934, #64276, #17030, #82470, #9204, #8048, #42579, #79785, #25644, #25836, #26602, #72259, #17085, #80890, #13620, #55416, #24873, #38217, #15636, #48020, #22908, #46075, #58694, #48636, #13737, #47270, #50460, #87018, #30207, #73782, #42472, #64761, #60557, #10733, #29291, #26295, #75945, #67540, #4137, #82738, #4359, #37053, #29837, #70201, #70105, #47337, #59036, #33056, #64779, #69400, #35065, #41109, #58490, #72889, #1573, #34814, #54959, #17716, #5825, #34402, #87656, #74839, #14559, #74380, #65211, #82533, #66998, #53645, #15441, #15506, #51506, #72474, #44778, #66243, #70004, #45167, #18462, #88502, #14748, #50148, #38530, #38295, #34284, #82967, #39333, #27225, #13177, #88554, #75402, #56573, #23551, #78843, #10585, #12887, #11450, #82751, #13577, #47287, #23040, #82858, #77907, #32146, #56562, #48519, #28537, #70877, #10335, #58854, #30321, #26959, #5848, #45062, #57326, #53828, #68661, #19334, #18816, #7637, #45453, #11955, #30349, #29832, #56883, #30806, #76175, #17847, #13595, #57264, #77823, #65880, #43859, #19667, #61728, #39810, #62092, #26049, #6928, #53354, #7545, #43958, #36576, #15729, #38210, #34640, #12134, #11956, #10562, #12354, #14937, #11308, #4008, #55301, #56868, #75663, #42031, #44035, #79644, #75154, #46925, #40144, #16129, #63764, #61744, #54182, #79971, #65742, #80456, #8577, #86077, #51312, #54152, #3367, #71152, #6729, #14946, #78053, #84477, #87069, #80909, #71855, #44138, #68654, #83526, #46448, #49719, #87028 ) ) ;
#21312=CARTESIAN_POINT ( 'NONE',  ( 107.0667039024470313, -104.2784471599420755, -19.78219314458201694 ) ) ;
#21322=DIRECTION ( 'NONE',  ( 0.000000000000000000, 0.000000000000000000, 1.000000000000000000 ) ) ;
#21332=DIRECTION ( 'NONE',  ( -0.7967329428042217998, 0.6043315462976631691, -1.908195823574488750E-14 ) ) ;
#21360=ORIENTED_EDGE ( 'NONE', *, *, #31742, .T. ) ;
#21373=AXIS2_PLACEMENT_3D ( 'NONE', #8083, #817, #71218 ) ;
#21390=EDGE_CURVE ( 'NONE', #16883, #64854, #88621, .T. ) ;
#21395=DIRECTION ( 'NONE',  ( -3.100000000000000258E-29, 3.100000000000000044E-14, 1.000000000000000000 ) ) ;
#21398=CARTESIAN_POINT ( 'NONE',  ( 80.78702870777534883, -128.1369015726494922, 249.3173333679100097 ) ) ;
#21405=( NAMED_UNIT ( * ) PLANE_ANGLE_UNIT ( ) SI_UNIT ( $, .RADIAN. ) );
#21409=FACE_OUTER_BOUND ( 'NONE', #8796, .T. ) ;
#21423=APPLICATION_CONTEXT ( 'automotive_design' ) ;
#21424=VECTOR ( 'NONE', #78307, 1000.000000000000000 ) ;
#21427=DIRECTION ( 'NONE',  ( -3.100000000000000258E-29, 3.100000000000000044E-14, 1.000000000000000000 ) ) ;
#21456=EDGE_LOOP ( 'NONE', ( #83881, #70150 ) ) ;
#21475=ORIENTED_EDGE ( 'NONE', *, *, #50674, .T. ) ;
#21501=AXIS2_PLACEMENT_3D ( 'NONE', #47939, #61139, #75680 ) ;
#21502=CARTESIAN_POINT ( 'NONE',  ( 107.0667039024470313, -104.2784471599420755, -19.78219314458201694 ) ) ;
#21503=CARTESIAN_POINT ( 'NONE',  ( 70.44731575448797400, -139.9957943335142545, 247.0389897592665989 ) ) ;
#21508=ORIENTED_EDGE ( 'NONE', *, *, #78168, .F. ) ;
#21515=CARTESIAN_POINT ( 'NONE',  ( 68.70199213936925275, -139.2946332222375361, 245.8922333760937136 ) ) ;
#21527=DIRECTION ( 'NONE',  ( 1.000000000000000078E-15, -1.000000000000000000, 0.000000000000000000 ) ) ;
#21534=CARTESIAN_POINT ( 'NONE',  ( 117.4590087478601248, -92.77844715994211811, -21.78219314458237932 ) ) ;
#21541=ORIENTED_EDGE ( 'NONE', *, *, #23708, .F. ) ;
#21552=ORIENTED_EDGE ( 'NONE', *, *, #16731, .T. ) ;
#21553=ORIENTED_EDGE ( 'NONE', *, *, #42090, .T. ) ;
#21554=ORIENTED_EDGE ( 'NONE', *, *, #59519, .T. ) ;
#21565=CARTESIAN_POINT ( 'NONE',  ( 68.06662902182972630, -68.83619408334048728, 247.2278077909978151 ) ) ;
#21568=ORIENTED_EDGE ( 'NONE', *, *, #5499, .F. ) ;
#21615=CIRCLE ( 'NONE', #76714, 3.000000000000002665 ) ;
#21625=CARTESIAN_POINT ( 'NONE',  ( 92.81551872686561921, -95.01002112898683549, -21.78219314458229405 ) ) ;
#21630=DIRECTION ( 'NONE',  ( -1.000000000000000078E-15, 1.000000000000000000, 0.000000000000000000 ) ) ;
#21635=VECTOR ( 'NONE', #62688, 1000.000000000000000 ) ;
#21653=ORIENTED_EDGE ( 'NONE', *, *, #5798, .F. ) ;
#21676=CARTESIAN_POINT ( 'NONE',  ( 85.06670390244703128, -80.35669973212958439, 55.21780685541800437 ) ) ;
#21701=CARTESIAN_POINT ( 'NONE',  ( 106.5667039024470455, -113.7784471599420613, -19.78219314458171141 ) ) ;
#21707=CARTESIAN_POINT ( 'NONE',  ( 144.0667039004811443, -140.6784471619068029, 245.4415720117440003 ) ) ;
#21713=DIRECTION ( 'NONE',  ( -1.000000000000000000, -1.181088324069315053E-15, 0.000000000000000000 ) ) ;
#21722=EDGE_LOOP ( 'NONE', ( #9831, #61514, #9794, #77707 ) ) ;
#21736=CARTESIAN_POINT ( 'NONE',  ( 91.00420390244700286, -68.87844715994096134, 55.21780685541800437 ) ) ;
#21740=DIRECTION ( 'NONE',  ( -1.000000000000000000, -1.734723475976808672E-15, 0.000000000000000000 ) ) ;
#21757=AXIS2_PLACEMENT_3D ( 'NONE', #49149, #14666, #29185 ) ;
#21758=ORIENTED_EDGE ( 'NONE', *, *, #71952, .F. ) ;
#21763=PRODUCT_DEFINITION_FORMATION_WITH_SPECIFIED_SOURCE ( 'ANY', '', #60378, .NOT_KNOWN. ) ;
#21766=DIRECTION ( 'NONE',  ( -3.100000000000000258E-29, 3.100000000000000044E-14, 1.000000000000000000 ) ) ;
#21776=COLOUR_RGB ( '', 0.66274510, 0.83137255, 0.94901961) ;
#21783=ORIENTED_EDGE ( 'NONE', *, *, #38100, .T. ) ;
#21799=ORIENTED_EDGE ( 'NONE', *, *, #5922, .T. ) ;
#21808=CARTESIAN_POINT ( 'NONE',  ( 68.77377604071689632, -69.45229246467815187, 247.4784000562319761 ) ) ;
#21813=DIRECTION ( 'NONE',  ( -1.000000000000000000, -8.163404592832032979E-16, 0.000000000000000000 ) ) ;
#21820=VECTOR ( 'NONE', #46802, 1000.000000000000000 ) ;
#21828=CARTESIAN_POINT ( 'NONE',  ( 121.3178890780284434, -113.5468731908973439, -19.18411693322874356 ) ) ;
#21857=VECTOR ( 'NONE', #663, 999.9999999999998863 ) ;
#21887=LINE ( 'NONE', #75943, #79019 ) ;
#21888=CARTESIAN_POINT ( 'NONE',  ( 67.65446888119937796, -138.2662121386932768, 245.5138901987639883 ) ) ;
#21905=CARTESIAN_POINT ( 'NONE',  ( 63.06670390244699576, -67.87844715994098976, 190.2178068554179902 ) ) ;
#21921=VERTEX_POINT ( 'NONE', #54061 ) ;
#21942=VERTEX_POINT ( 'NONE', #78596 ) ;
#21955=EDGE_LOOP ( 'NONE', ( #20027, #85567, #14759, #14645, #72315 ) ) ;
#21959=CARTESIAN_POINT ( 'NONE',  ( 70.36520983569781151, -140.1685435066830223, 246.8677938034485635 ) ) ;
#21974=VECTOR ( 'NONE', #41830, 1000.000000000000000 ) ;
#21985=CIRCLE ( 'NONE', #23479, 1.999999999999995781 ) ;
#21986=DIRECTION ( 'NONE',  ( 1.000000000000000000, 1.000000000000000078E-15, 0.000000000000000000 ) ) ;
#21990=ORIENTED_EDGE ( 'NONE', *, *, #80777, .F. ) ;
#21999=DIRECTION ( 'NONE',  ( 1.157009245868378063E-15, -1.000000000000000000, 3.100000000000000044E-14 ) ) ;
#22015=CARTESIAN_POINT ( 'NONE',  ( 127.0667052882550081, -78.66107132697013071, 55.21780685541800437 ) ) ;
#22041=CARTESIAN_POINT ( 'NONE',  ( 106.5667039024470171, -94.77844715994206126, -19.78219314458232247 ) ) ;
#22053=ORIENTED_EDGE ( 'NONE', *, *, #6806, .T. ) ;
#22065=DIRECTION ( 'NONE',  ( -8.953411488912552682E-16, 1.000000000000000000, 0.000000000000000000 ) ) ;
#22085=DIRECTION ( 'NONE',  ( -0.8660254037844380415, -0.5000000000000012212, 1.550000000000001284E-14 ) ) ;
#22091=CARTESIAN_POINT ( 'NONE',  ( 146.4958942568945588, -137.3566279360900921, 246.9078157516118779 ) ) ;
#22103=CARTESIAN_POINT ( 'NONE',  ( 98.58946256649487339, -99.96145986183429955, -19.78219314458215550 ) ) ;
#22112=DIRECTION ( 'NONE',  ( 1.000000000000000000, 1.000000000000000078E-15, 0.000000000000000000 ) ) ;
#22115=AXIS2_PLACEMENT_3D ( 'NONE', #82544, #13926, #61604 ) ;
#22122=ORIENTED_EDGE ( 'NONE', *, *, #49003, .F. ) ;
#22138=EDGE_CURVE ( 'NONE', #64928, #41501, #34590, .T. ) ;
#22139=DIRECTION ( 'NONE',  ( 0.000000000000000000, 0.000000000000000000, 1.000000000000000000 ) ) ;
#22151=ORIENTED_EDGE ( 'NONE', *, *, #50337, .F. ) ;
#22188=FACE_OUTER_BOUND ( 'NONE', #43252, .T. ) ;
#22189=CARTESIAN_POINT ( 'NONE',  ( 98.58946256649485917, -108.5954344580498514, -19.78219314458187839 ) ) ;
#22194=ORIENTED_EDGE ( 'NONE', *, *, #45770, .T. ) ;
#22207=CARTESIAN_POINT ( 'NONE',  ( 107.0667039024470313, -104.2784471599412086, 7.717806855417980394 ) ) ;
#22213=FACE_OUTER_BOUND ( 'NONE', #55576, .T. ) ;
#22221=DIRECTION ( 'NONE',  ( 0.8660254037844382635, 0.5000000000000008882, -1.550000000000000022E-14 ) ) ;
#22226=EDGE_CURVE ( 'NONE', #27286, #40899, #67159, .T. ) ;
#22233=VERTEX_POINT ( 'NONE', #10861 ) ;
#22244=CARTESIAN_POINT ( 'NONE',  ( 107.5667039024470171, -94.77844715994137914, 2.217806855417697953 ) ) ;
#22259=CARTESIAN_POINT ( 'NONE',  ( 107.0667039024470313, -104.2784471599420471, -19.18411693322902423 ) ) ;
#22270=CARTESIAN_POINT ( 'NONE',  ( 140.0167039024470910, -144.7284471599409414, 55.21780685541800437 ) ) ;
#22292=AXIS2_PLACEMENT_3D ( 'NONE', #22326, #56372, #58176 ) ;
#22302=EDGE_CURVE ( 'NONE', #54218, #15323, #33975, .T. ) ;
#22304=SURFACE_STYLE_FILL_AREA ( #56345 ) ;
#22310=CARTESIAN_POINT ( 'NONE',  ( 127.4058501689331280, -122.7870702624433221, 250.2178068554179902 ) ) ;
#22318=VERTEX_POINT ( 'NONE', #60791 ) ;
#22323=DIRECTION ( 'NONE',  ( 1.000000000000000078E-15, -1.000000000000000000, 0.000000000000000000 ) ) ;
#22326=CARTESIAN_POINT ( 'NONE',  ( 74.06670390244704549, -118.2784471599409812, 51.21780685541800437 ) ) ;
#22333=ORIENTED_EDGE ( 'NONE', *, *, #65864, .F. ) ;
#22348=CARTESIAN_POINT ( 'NONE',  ( 107.0667039024470313, -104.2784471599418197, -11.78219314458200984 ) ) ;
#22363=CARTESIAN_POINT ( 'NONE',  ( 107.0667039024469886, -67.87844715994094713, 93.21780685541800437 ) ) ;
#22392=CARTESIAN_POINT ( 'NONE',  ( 70.06670390244705970, -124.7784471599409812, 55.21780685541800437 ) ) ;
#22411=DIRECTION ( 'NONE',  ( -0.8660254037844392627, 0.4999999999999990008, -1.549999999999999706E-14 ) ) ;
#22412=CIRCLE ( 'NONE', #2121, 4.500000000000003553 ) ;
#22417=LINE ( 'NONE', #15149, #11506 ) ;
#22418=DIRECTION ( 'NONE',  ( 0.000000000000000000, 0.000000000000000000, -1.000000000000000000 ) ) ;
#22438=CARTESIAN_POINT ( 'NONE',  ( 154.5667039024469886, -67.87844715994090450, 120.2178068554179902 ) ) ;
#22440=DIRECTION ( 'NONE',  ( 3.100000000000000258E-29, -3.100000000000000044E-14, -1.000000000000000000 ) ) ;
#22448=CARTESIAN_POINT ( 'NONE',  ( 127.4058501689330996, -85.76982405743852667, 250.2178068554179902 ) ) ;
#22451=AXIS2_PLACEMENT_3D ( 'NONE', #6750, #7650, #54869 ) ;
#22452=DIRECTION ( 'NONE',  ( -1.000000000000000078E-15, 1.000000000000000000, 0.000000000000000000 ) ) ;
#22453=CARTESIAN_POINT ( 'NONE',  ( 115.0439452383991892, -99.09543445804983719, -19.78219314458218392 ) ) ;
#22457=CARTESIAN_POINT ( 'NONE',  ( 67.07017578645290712, -67.88084389459083923, 245.6085276058775264 ) ) ;
#22463=EDGE_CURVE ( 'NONE', #16335, #85940, #28504, .T. ) ;
#22468=DIRECTION ( 'NONE',  ( -3.100000000000000258E-29, 3.100000000000000044E-14, 1.000000000000000000 ) ) ;
#22476=ORIENTED_EDGE ( 'NONE', *, *, #10807, .F. ) ;
#22486=CYLINDRICAL_SURFACE ( 'NONE', #8665, 3.000000000000002665 ) ;
#22487=VERTEX_POINT ( 'NONE', #36688 ) ;
#22506=VERTEX_POINT ( 'NONE', #22614 ) ;
#22509=ORIENTED_EDGE ( 'NONE', *, *, #47771, .T. ) ;
#22512=DIRECTION ( 'NONE',  ( 1.000000000000000000, 1.000000000000000078E-15, 0.000000000000000000 ) ) ;
#22540=CARTESIAN_POINT ( 'NONE',  ( 144.0646911277377740, -140.6784471599409017, 245.5179332673170052 ) ) ;
#22546=CIRCLE ( 'NONE', #13764, 8.999999999999994671 ) ;
#22555=FACE_OUTER_BOUND ( 'NONE', #42315, .T. ) ;
#22568=DIRECTION ( 'NONE',  ( -3.100000000000000258E-29, 3.100000000000000044E-14, 1.000000000000000000 ) ) ;
#22569=AXIS2_PLACEMENT_3D ( 'NONE', #6986, #69214, #41046 ) ;
#22576=EDGE_CURVE ( 'NONE', #24886, #5965, #10612, .T. ) ;
#22577=LINE ( 'NONE', #84366, #63701 ) ;
#22585=ORIENTED_EDGE ( 'NONE', *, *, #67509, .T. ) ;
#22589=VERTEX_POINT ( 'NONE', #72975 ) ;
#22594=AXIS2_PLACEMENT_3D ( 'NONE', #74043, #19078, #79991 ) ;
#22611=AXIS2_PLACEMENT_3D ( 'NONE', #3829, #22959, #37907 ) ;
#22614=CARTESIAN_POINT ( 'NONE',  ( 56.06670390244699576, -67.87844715994098976, 155.2178068554179902 ) ) ;
#22635=LINE ( 'NONE', #3399, #2951 ) ;
#22636=CARTESIAN_POINT ( 'NONE',  ( 106.5667039024470455, -113.7784471599413791, 2.217806855418308132 ) ) ;
#22638=EDGE_CURVE ( 'NONE', #86558, #75555, #52060, .T. ) ;
#22646=LINE ( 'NONE', #71684, #31642 ) ;
#22655=EDGE_LOOP ( 'NONE', ( #84941, #77389, #46020, #34007, #85246, #66623 ) ) ;
#22691=ORIENTED_EDGE ( 'NONE', *, *, #7351, .T. ) ;
#22694=ORIENTED_EDGE ( 'NONE', *, *, #41800, .T. ) ;
#22709=ORIENTED_EDGE ( 'NONE', *, *, #62653, .F. ) ;
#22711=LINE ( 'NONE', #72640, #35250 ) ;
#22722=ORIENTED_EDGE ( 'NONE', *, *, #29449, .F. ) ;
#22736=CARTESIAN_POINT ( 'NONE',  ( 131.5667039024470455, -104.2784471599409244, 22.21780685541800082 ) ) ;
#22769=PLANE ( 'NONE',  #10991 ) ;
#22774=VECTOR ( 'NONE', #51419, 1000.000000000000000 ) ;
#22778=CARTESIAN_POINT ( 'NONE',  ( 67.06670390244705970, -127.7048251178302678, 245.5588921750969860 ) ) ;
#22783=CARTESIAN_POINT ( 'NONE',  ( 108.9744791726666051, -76.77844715994095282, 250.2178068554179902 ) ) ;
#22786=VECTOR ( 'NONE', #51239, 1000.000000000000000 ) ;
#22811=AXIS2_PLACEMENT_3D ( 'NONE', #76966, #35618, #7918 ) ;
#22816=ORIENTED_EDGE ( 'NONE', *, *, #78270, .F. ) ;
#22822=CARTESIAN_POINT ( 'NONE',  ( 68.77377604071689632, -69.45229246467815187, 247.4784000562319761 ) ) ;
#22823=CARTESIAN_POINT ( 'NONE',  ( 107.0667039024470313, -104.2784471599409528, 22.21780685541800082 ) ) ;
#22858=CIRCLE ( 'NONE', #19925, 8.999999999999994671 ) ;
#22866=EDGE_CURVE ( 'NONE', #68825, #23110, #70538, .T. ) ;
#22871=CARTESIAN_POINT ( 'NONE',  ( 144.5667039024470455, -118.2784471599408960, 51.21780685541800437 ) ) ;
#22878=VECTOR ( 'NONE', #43024, 1000.000000000000000 ) ;
#22881=FACE_OUTER_BOUND ( 'NONE', #52691, .T. ) ;
#22903=CARTESIAN_POINT ( 'NONE',  ( 128.5446125969797606, -87.02121134100629263, 250.2178068554179902 ) ) ;
#22908=ADVANCED_FACE ( 'NONE', ( #16915 ), #58665, .F. ) ;
#22909=PLANE ( 'NONE',  #5426 ) ;
#22924=CARTESIAN_POINT ( 'NONE',  ( 107.0667039024470313, -104.2784471599413791, 2.217806855418003043 ) ) ;
#22942=VECTOR ( 'NONE', #23146, 1000.000000000000000 ) ;
#22959=DIRECTION ( 'NONE',  ( 3.100000000000000258E-29, -3.100000000000000044E-14, -1.000000000000000000 ) ) ;
#22961=CARTESIAN_POINT ( 'NONE',  ( 68.66208373768751017, -72.70246804406471597, 247.4783998280180128 ) ) ;
#22962=EDGE_LOOP ( 'NONE', ( #38669, #57424, #84165, #11719, #82926, #33879 ) ) ;
#22986=CARTESIAN_POINT ( 'NONE',  ( 74.19170390244700286, -80.65344715994098124, 55.21780685541800437 ) ) ;
#22995=CARTESIAN_POINT ( 'NONE',  ( 97.81670390244700286, -67.87844715994096134, 96.96780685541800437 ) ) ;
#22997=CARTESIAN_POINT ( 'NONE',  ( 52.06670390244700286, -77.67844715994100113, 222.2178068554179902 ) ) ;
#22999=VECTOR ( 'NONE', #63062, 999.9999999999998863 ) ;
#23003=CIRCLE ( 'NONE', #41820, 30.99999999999998579 ) ;
#23040=ADVANCED_FACE ( 'NONE', ( #80044 ), #88648, .F. ) ;
#23057=ORIENTED_EDGE ( 'NONE', *, *, #13813, .T. ) ;
#23067=CARTESIAN_POINT ( 'NONE',  ( 107.0667039024470313, -104.2784471599420755, -19.78219314458201694 ) ) ;
#23084=DIRECTION ( 'NONE',  ( 0.000000000000000000, 0.000000000000000000, 1.000000000000000000 ) ) ;
#23097=ORIENTED_EDGE ( 'NONE', *, *, #53013, .F. ) ;
#23110=VERTEX_POINT ( 'NONE', #69090 ) ;
#23139=ORIENTED_EDGE ( 'NONE', *, *, #69065, .F. ) ;
#23145=CIRCLE ( 'NONE', #48656, 4.500000000000003553 ) ;
#23146=DIRECTION ( 'NONE',  ( -0.8660254037844392627, 0.4999999999999990008, -1.549999999999999706E-14 ) ) ;
#23150=DIRECTION ( 'NONE',  ( 1.000000000000000000, 0.000000000000000000, 0.000000000000000000 ) ) ;
#23187=CARTESIAN_POINT ( 'NONE',  ( 107.0667039024470313, -104.2784471599409528, 45.21780685541799727 ) ) ;
#23231=EDGE_CURVE ( 'NONE', #26317, #11051, #16371, .T. ) ;
#23291=CYLINDRICAL_SURFACE ( 'NONE', #21757, 11.49999999999999645 ) ;
#23320=DIRECTION ( 'NONE',  ( -0.7071067811865463515, -0.7071067811865487940, 0.000000000000000000 ) ) ;
#23321=CARTESIAN_POINT ( 'NONE',  ( 68.80903792918766726, -139.1904132598590422, 246.4625416178163562 ) ) ;
#23325=AXIS2_PLACEMENT_3D ( 'NONE', #32182, #4498, #72649 ) ;
#23326=DIRECTION ( 'NONE',  ( 0.000000000000000000, 0.000000000000000000, 1.000000000000000000 ) ) ;
#23338=EDGE_LOOP ( 'NONE', ( #89717, #14738 ) ) ;
#23339=FACE_OUTER_BOUND ( 'NONE', #17451, .T. ) ;
#23341=CIRCLE ( 'NONE', #34911, 17.00000000000000000 ) ;
#23372=ORIENTED_EDGE ( 'NONE', *, *, #83865, .F. ) ;
#23425=LINE ( 'NONE', #17477, #88270 ) ;
#23444=DIRECTION ( 'NONE',  ( -1.000000000000000078E-15, 1.000000000000000000, -3.100000000000000044E-14 ) ) ;
#23449=LINE ( 'NONE', #37944, #45613 ) ;
#23458=AXIS2_PLACEMENT_3D ( 'NONE', #36139, #1177, #57015 ) ;
#23459=LINE ( 'NONE', #17945, #47129 ) ;
#23475=EDGE_CURVE ( 'NONE', #78082, #59268, #28076, .T. ) ;
#23479=AXIS2_PLACEMENT_3D ( 'NONE', #69995, #85443, #15493 ) ;
#23495=FACE_OUTER_BOUND ( 'NONE', #45661, .T. ) ;
#23501=AXIS2_PLACEMENT_3D ( 'NONE', #80502, #60021, #11454 ) ;
#23525=LINE ( 'NONE', #16693, #2577 ) ;
#23528=DIRECTION ( 'NONE',  ( 1.000000000000000000, 1.000000000000000078E-15, 0.000000000000000000 ) ) ;
#23537=CARTESIAN_POINT ( 'NONE',  ( 144.0667052733537901, -71.37844715994090450, 55.21780685541800437 ) ) ;
#23538=CARTESIAN_POINT ( 'NONE',  ( 59.56670390244700997, -79.67844715994098692, 85.21780685541799016 ) ) ;
#23551=ADVANCED_FACE ( 'NONE', ( #42150 ), #68981, .F. ) ;
#23559=ADVANCED_FACE ( 'NONE', ( #61699 ), #381, .F. ) ;
#23564=EDGE_LOOP ( 'NONE', ( #3543, #62723, #66241, #71716, #11106, #57535 ) ) ;
#23568=VECTOR ( 'NONE', #61237, 999.9999999999998863 ) ;
#23571=EDGE_CURVE ( 'NONE', #33311, #56525, #64530, .T. ) ;
#23594=EDGE_CURVE ( 'NONE', #63455, #34012, #78050, .T. ) ;
#23602=CARTESIAN_POINT ( 'NONE',  ( 68.91422814837490307, -69.55937875643057566, 247.4998451774034152 ) ) ;
#23606=AXIS2_PLACEMENT_3D ( 'NONE', #22363, #50037, #77776 ) ;
#23611=ORIENTED_EDGE ( 'NONE', *, *, #80991, .F. ) ;
#23612=VERTEX_POINT ( 'NONE', #22636 ) ;
#23627=DIRECTION ( 'NONE',  ( 1.000000000000000000, 0.000000000000000000, 0.000000000000000000 ) ) ;
#23636=LINE ( 'NONE', #9108, #49471 ) ;
#23655=EDGE_CURVE ( 'NONE', #65590, #17260, #646, .T. ) ;
#23685=ORIENTED_EDGE ( 'NONE', *, *, #18622, .F. ) ;
#23686=ORIENTED_EDGE ( 'NONE', *, *, #26800, .T. ) ;
#23699=ORIENTED_EDGE ( 'NONE', *, *, #49367, .T. ) ;
#23701=CARTESIAN_POINT ( 'NONE',  ( 121.2221484686747317, -94.95109689075218284, -11.78219314458228695 ) ) ;
#23703=EDGE_CURVE ( 'NONE', #61554, #25758, #7914, .T. ) ;
#23708=EDGE_CURVE ( 'NONE', #2107, #4290, #9006, .T. ) ;
#23720=DIRECTION ( 'NONE',  ( 1.000000000000000000, 0.000000000000000000, 0.000000000000000000 ) ) ;
#23723=FACE_OUTER_BOUND ( 'NONE', #3465, .T. ) ;
#23738=ORIENTED_EDGE ( 'NONE', *, *, #31742, .F. ) ;
#23740=ORIENTED_EDGE ( 'NONE', *, *, #75622, .F. ) ;
#23754=CARTESIAN_POINT ( 'NONE',  ( 68.77810336616866493, -139.2209757805153174, 246.3536556105786417 ) ) ;
#23761=FACE_OUTER_BOUND ( 'NONE', #80325, .T. ) ;
#23771=EDGE_CURVE ( 'NONE', #11533, #51807, #38022, .T. ) ;
#23781=AXIS2_PLACEMENT_3D ( 'NONE', #70711, #22568, #20760 ) ;
#23786=CARTESIAN_POINT ( 'NONE',  ( 132.2857443282840393, -124.7784471599409102, 222.2178068554179902 ) ) ;
#23789=CARTESIAN_POINT ( 'NONE',  ( 145.7566936099118777, -137.2574666318677998, 247.4285154401919726 ) ) ;
#23799=DIRECTION ( 'NONE',  ( 1.000000000000000000, 1.000000000000000078E-15, 0.000000000000000000 ) ) ;
#23806=ORIENTED_EDGE ( 'NONE', *, *, #53457, .F. ) ;
#23808=CARTESIAN_POINT ( 'NONE',  ( 146.9552639810710559, -67.98257152991943997, 246.1456466833680281 ) ) ;
#23811=EDGE_CURVE ( 'NONE', #83896, #65511, #11213, .T. ) ;
#23818=VERTEX_POINT ( 'NONE', #4855 ) ;
#23842=B_SPLINE_CURVE_WITH_KNOTS ( 'NONE', 3,
 ( #21808, #49478, #79003, #15440, #14986, #64917, #57189, #2702, #36321, #64031, #8168, #23602, #1809, #29507 ),
 .UNSPECIFIED., .F., .F.,
 ( 4, 2, 2, 2, 2, 2, 4 ),
 ( 0.000000000000000000, 0.4999999999997828404, 0.7499999999996677102, 0.8749999999996868061, 0.9374999999997890576, 0.9687499999998945288, 1.000000000000000000 ),
 .UNSPECIFIED. ) ;
#23846=CARTESIAN_POINT ( 'NONE',  ( 80.75702474444096879, -128.2461948925749766, 249.3055308415380011 ) ) ;
#23855=CARTESIAN_POINT ( 'NONE',  ( 143.4979113519680993, -139.5802913934610103, 247.3215535119185517 ) ) ;
#23863=EDGE_CURVE ( 'NONE', #44698, #75678, #12117, .T. ) ;
#23864=CARTESIAN_POINT ( 'NONE',  ( 67.54744102787780946, -137.3996135046812412, 246.8082721997937767 ) ) ;
#23885=VERTEX_POINT ( 'NONE', #31207 ) ;
#23888=DIRECTION ( 'NONE',  ( -1.150535366796005147E-15, 1.000000000000000000, -3.100000000000000044E-14 ) ) ;
#23891=CARTESIAN_POINT ( 'NONE',  ( 122.2221484686747459, -104.2784471599418055, -11.78219314458200984 ) ) ;
#23909=PLANE ( 'NONE',  #82271 ) ;
#23914=DIRECTION ( 'NONE',  ( -0.7071067811865496822, 0.7071067811865453523, 0.000000000000000000 ) ) ;
#23922=ORIENTED_EDGE ( 'NONE', *, *, #37978, .F. ) ;
#23934=CIRCLE ( 'NONE', #57305, 173.3227045126509722 ) ;
#23950=CARTESIAN_POINT ( 'NONE',  ( 147.0667039024470455, -124.3811607159765060, 245.5761019086199894 ) ) ;
#23951=ORIENTED_EDGE ( 'NONE', *, *, #41903, .F. ) ;
#23955=AXIS2_PLACEMENT_3D ( 'NONE', #6137, #32469, #39299 ) ;
#23973=DIRECTION ( 'NONE',  ( -3.100000000000000258E-29, 3.100000000000000044E-14, 1.000000000000000000 ) ) ;
#23987=VECTOR ( 'NONE', #22418, 1000.000000000000000 ) ;
#24017=AXIS2_PLACEMENT_3D ( 'NONE', #19523, #40852, #21322 ) ;
#24026=ORIENTED_EDGE ( 'NONE', *, *, #34586, .T. ) ;
#24028=DIRECTION ( 'NONE',  ( -3.100000000000000258E-29, 3.100000000000000044E-14, 1.000000000000000000 ) ) ;
#24037=DIRECTION ( 'NONE',  ( -1.000000000000000000, 0.000000000000000000, 0.000000000000000000 ) ) ;
#24038=CARTESIAN_POINT ( 'NONE',  ( 131.8339555767850015, -67.87837171461835339, 246.1340590712410119 ) ) ;
#24043=FACE_OUTER_BOUND ( 'NONE', #60038, .T. ) ;
#24051=DIRECTION ( 'NONE',  ( 1.000000000000000000, 0.000000000000000000, 0.000000000000000000 ) ) ;
#24085=VERTEX_POINT ( 'NONE', #21178 ) ;
#24098=ORIENTED_EDGE ( 'NONE', *, *, #22302, .F. ) ;
#24101=EDGE_CURVE ( 'NONE', #63455, #35252, #68873, .T. ) ;
#24120=CARTESIAN_POINT ( 'NONE',  ( 132.2857443282839824, -83.77844715994092439, 222.2178068554179902 ) ) ;
#24128=CARTESIAN_POINT ( 'NONE',  ( 143.0667039024470171, -83.77844715994091018, 45.21780685541799727 ) ) ;
#24130=ORIENTED_EDGE ( 'NONE', *, *, #86056, .T. ) ;
#24131=FACE_OUTER_BOUND ( 'NONE', #84087, .T. ) ;
#24156=FACE_OUTER_BOUND ( 'NONE', #26292, .T. ) ;
#24160=EDGE_CURVE ( 'NONE', #51228, #51923, #23934, .T. ) ;
#24166=ORIENTED_EDGE ( 'NONE', *, *, #4372, .T. ) ;
#24196=CARTESIAN_POINT ( 'NONE',  ( 91.91125933621943034, -104.2784471599418339, -11.78219314458200984 ) ) ;
#24210=VECTOR ( 'NONE', #43544, 1000.000000000000000 ) ;
#24217=DIRECTION ( 'NONE',  ( 0.7071067811865536790, -0.7071067811865414665, 0.000000000000000000 ) ) ;
#24222=CARTESIAN_POINT ( 'NONE',  ( 121.2221484686747317, -94.95109689075241022, -19.26696060647628528 ) ) ;
#24233=LINE ( 'NONE', #16087, #82528 ) ;
#24243=CARTESIAN_POINT ( 'NONE',  ( 74.81190481564590300, -74.97944988200733007, 248.4067532124560103 ) ) ;
#24244=CARTESIAN_POINT ( 'NONE',  ( 145.9361736036992454, -68.96302025968714133, 247.2980205078839333 ) ) ;
#24258=FACE_OUTER_BOUND ( 'NONE', #51007, .T. ) ;
#24263=ORIENTED_EDGE ( 'NONE', *, *, #13023, .T. ) ;
#24299=DIRECTION ( 'NONE',  ( -1.000000000000000078E-15, 1.000000000000000000, 0.000000000000000000 ) ) ;
#24302=CARTESIAN_POINT ( 'NONE',  ( 59.56670390244699576, -67.87844715994098976, 190.2178068554179902 ) ) ;
#24305=CARTESIAN_POINT ( 'NONE',  ( 68.18421604846717798, -137.1080028910827480, 247.3042482208074944 ) ) ;
#24315=EDGE_CURVE ( 'NONE', #62435, #38828, #86405, .T. ) ;
#24316=CARTESIAN_POINT ( 'NONE',  ( 81.84766347661003749, -124.7784471599409670, 45.21780685541799727 ) ) ;
#24323=ORIENTED_EDGE ( 'NONE', *, *, #53717, .F. ) ;
#24329=CARTESIAN_POINT ( 'NONE',  ( 122.2221484686747317, -96.68314769832106492, -11.78219314458223188 ) ) ;
#24356=CIRCLE ( 'NONE', #20007, 24.50000000000000711 ) ;
#24357=CARTESIAN_POINT ( 'NONE',  ( 84.56587091301777548, -120.1789271773121186, 250.2178068554179902 ) ) ;
#24371=DIRECTION ( 'NONE',  ( -3.100000000000000258E-29, 3.100000000000000044E-14, 1.000000000000000000 ) ) ;
#24383=B_SPLINE_CURVE_WITH_KNOTS ( 'NONE', 3,
 ( #37579, #44820, #66152, #52500 ),
 .UNSPECIFIED., .F., .F.,
 ( 4, 4 ),
 ( -0.6035999334370359959, -0.5903216970416040876 ),
 .UNSPECIFIED. ) ;
#24394=ORIENTED_EDGE ( 'NONE', *, *, #40348, .F. ) ;
#24399=CARTESIAN_POINT ( 'NONE',  ( 143.5667039024469886, -67.87844715994090450, 222.2178068554179902 ) ) ;
#24405=CARTESIAN_POINT ( 'NONE',  ( 104.0667030381801936, -67.87844715994094713, 173.2178086137559774 ) ) ;
#24419=ORIENTED_EDGE ( 'NONE', *, *, #45751, .T. ) ;
#24431=VERTEX_POINT ( 'NONE', #40601 ) ;
#24432=VERTEX_POINT ( 'NONE', #81963 ) ;
#24457=CARTESIAN_POINT ( 'NONE',  ( 99.08946256649487339, -99.09543445804918349, 2.217806855417836509 ) ) ;
#24467=VERTEX_POINT ( 'NONE', #76020 ) ;
#24469=CIRCLE ( 'NONE', #81094, 3.000000864267343026 ) ;
#24472=ORIENTED_EDGE ( 'NONE', *, *, #51404, .F. ) ;
#24477=CIRCLE ( 'NONE', #47660, 17.00000000000000000 ) ;
#24515=ORIENTED_EDGE ( 'NONE', *, *, #62653, .T. ) ;
#24521=AXIS2_PLACEMENT_3D ( 'NONE', #44161, #23320, #65516 ) ;
#24527=EDGE_CURVE ( 'NONE', #76266, #49377, #81071, .T. ) ;
#24528=AXIS2_PLACEMENT_3D ( 'NONE', #21312, #76724, #16739 ) ;
#24561=CARTESIAN_POINT ( 'NONE',  ( 97.06670390244703128, -104.2784471599412228, 7.717806855417980394 ) ) ;
#24565=CARTESIAN_POINT ( 'NONE',  ( 115.5439452383991892, -99.96145986183358900, 2.217806855417864043 ) ) ;
#24570=CYLINDRICAL_SURFACE ( 'NONE', #46382, 2.999999999999988898 ) ;
#24580=FACE_OUTER_BOUND ( 'NONE', #12825, .T. ) ;
#24583=VECTOR ( 'NONE', #71448, 1000.000000000000000 ) ;
#24600=ORIENTED_EDGE ( 'NONE', *, *, #63577, .F. ) ;
#24607=ORIENTED_EDGE ( 'NONE', *, *, #8, .T. ) ;
#24609=FACE_OUTER_BOUND ( 'NONE', #55725, .T. ) ;
#24614=ORIENTED_EDGE ( 'NONE', *, *, #9677, .T. ) ;
#24617=DIRECTION ( 'NONE',  ( 3.114895971316861016E-16, -1.000000000000000000, 0.000000000000000000 ) ) ;
#24619=DIRECTION ( 'NONE',  ( 1.000000000000000000, 1.000000000000000078E-15, 0.000000000000000000 ) ) ;
#24621=LINE ( 'NONE', #30546, #28675 ) ;
#24622=DIRECTION ( 'NONE',  ( 1.000000000000000000, 0.000000000000000000, 0.000000000000000000 ) ) ;
#24648=CIRCLE ( 'NONE', #78369, 3.499999999999996003 ) ;
#24673=CARTESIAN_POINT ( 'NONE',  ( 115.5439452383991892, -99.96145986183358900, 2.217806855417864043 ) ) ;
#24683=CARTESIAN_POINT ( 'NONE',  ( 85.12238035501010813, -78.13364596806115969, 249.3134381260879877 ) ) ;
#24684=CARTESIAN_POINT ( 'NONE',  ( 145.9495235048387940, -68.95052383084446035, 247.2914646300089885 ) ) ;
#24708=ORIENTED_EDGE ( 'NONE', *, *, #79981, .T. ) ;
#24713=ORIENTED_EDGE ( 'NONE', *, *, #10978, .F. ) ;
#24719=CARTESIAN_POINT ( 'NONE',  ( 107.0667039024470313, -104.2784471599412086, 7.717806855417980394 ) ) ;
#24728=ORIENTED_EDGE ( 'NONE', *, *, #25147, .F. ) ;
#24732=CARTESIAN_POINT ( 'NONE',  ( 81.84766347661003749, -124.7784471599409670, 222.2178068554179902 ) ) ;
#24733=CARTESIAN_POINT ( 'NONE',  ( 143.9462412624536398, -140.5180570844704278, 246.3267910350913610 ) ) ;
#24739=VECTOR ( 'NONE', #63121, 1000.000000000000000 ) ;
#24741=CARTESIAN_POINT ( 'NONE',  ( 68.27270054217888173, -137.0689115924293446, 247.3475429858000894 ) ) ;
#24752=CARTESIAN_POINT ( 'NONE',  ( 107.0667039024470313, -104.2784471599414502, 0.2178068554180012661 ) ) ;
#24760=ORIENTED_EDGE ( 'NONE', *, *, #27758, .F. ) ;
#24763=CARTESIAN_POINT ( 'NONE',  ( 78.56670390244704549, -118.2784471599409812, 45.21780685541799727 ) ) ;
#24775=ORIENTED_EDGE ( 'NONE', *, *, #61975, .F. ) ;
#24792=EDGE_CURVE ( 'NONE', #33837, #28990, #79962, .T. ) ;
#24800=CARTESIAN_POINT ( 'NONE',  ( 106.0667039024470171, -87.35579742913172652, -21.78219314458254630 ) ) ;
#24815=CARTESIAN_POINT ( 'NONE',  ( 107.0667039024470455, -135.2784471599409528, 25.71780685541800437 ) ) ;
#24817=ORIENTED_EDGE ( 'NONE', *, *, #20787, .T. ) ;
#24826=LINE ( 'NONE', #9863, #89562 ) ;
#24834=CARTESIAN_POINT ( 'NONE',  ( 67.06670390244700286, -67.87844715994098976, 222.2178068554179902 ) ) ;
#24848=CARTESIAN_POINT ( 'NONE',  ( 125.5177273812784762, -137.6784471599409301, 55.21780685541800437 ) ) ;
#24873=ADVANCED_FACE ( 'NONE', ( #50726 ), #42228, .F. ) ;
#24877=CARTESIAN_POINT ( 'NONE',  ( 107.0667039024470313, -104.2784471599409528, 249.2178068554179902 ) ) ;
#24882=CIRCLE ( 'NONE', #72734, 3.500000000000003109 ) ;
#24884=ORIENTED_EDGE ( 'NONE', *, *, #61975, .T. ) ;
#24886=VERTEX_POINT ( 'NONE', #16661 ) ;
#24889=CARTESIAN_POINT ( 'NONE',  ( 116.3167039024470029, -67.87844715994093292, 180.4678068554179902 ) ) ;
#24920=FACE_OUTER_BOUND ( 'NONE', #59970, .T. ) ;
#24941=DIRECTION ( 'NONE',  ( -1.000000000000000000, 0.000000000000000000, 0.000000000000000000 ) ) ;
#24942=ORIENTED_EDGE ( 'NONE', *, *, #29560, .T. ) ;
#24944=PLANE ( 'NONE',  #77922 ) ;
#24991=EDGE_CURVE ( 'NONE', #55038, #11706, #61113, .T. ) ;
#24995=EDGE_CURVE ( 'NONE', #31404, #56720, #80236, .T. ) ;
#25004=CARTESIAN_POINT ( 'NONE',  ( 115.0439452383992318, -109.4614598618342853, -19.78219314458184996 ) ) ;
#25035=ORIENTED_EDGE ( 'NONE', *, *, #46560, .T. ) ;
#25071=DIRECTION ( 'NONE',  ( -3.100000000000000258E-29, 3.100000000000000044E-14, 1.000000000000000000 ) ) ;
#25072=DIRECTION ( 'NONE',  ( -0.1250000000000000278, -0.9921567416492215186, 3.035766082959410522E-14 ) ) ;
#25078=CARTESIAN_POINT ( 'NONE',  ( 145.3505076167853076, -67.86861087870649101, 247.4717563792629846 ) ) ;
#25091=AXIS2_PLACEMENT_3D ( 'NONE', #88506, #33521, #26259 ) ;
#25101=PLANE ( 'NONE',  #793 ) ;
#25117=CIRCLE ( 'NONE', #68699, 17.00000000000000000 ) ;
#25124=CARTESIAN_POINT ( 'NONE',  ( 125.9429424436864196, -84.18539835298642515, 250.2201230397200220 ) ) ;
#25128=VECTOR ( 'NONE', #62416, 1000.000000000000000 ) ;
#25129=ORIENTED_EDGE ( 'NONE', *, *, #88602, .F. ) ;
#25147=EDGE_CURVE ( 'NONE', #11800, #9965, #79190, .T. ) ;
#25167=DIRECTION ( 'NONE',  ( 1.000000000000000000, 1.132880637372608296E-15, 0.000000000000000000 ) ) ;
#25184=CARTESIAN_POINT ( 'NONE',  ( 107.0667039024470313, -104.2784471599418197, -11.78219314458200984 ) ) ;
#25205=PLANE ( 'NONE',  #65696 ) ;
#25233=AXIS2_PLACEMENT_3D ( 'NONE', #74954, #46773, #39531 ) ;
#25238=VERTEX_POINT ( 'NONE', #45569 ) ;
#25246=DIRECTION ( 'NONE',  ( 1.000000000000000078E-15, -1.000000000000000000, 0.000000000000000000 ) ) ;
#25248=VERTEX_POINT ( 'NONE', #11987 ) ;
#25252=ORIENTED_EDGE ( 'NONE', *, *, #6806, .F. ) ;
#25255=EDGE_CURVE ( 'NONE', #4284, #20155, #25601, .T. ) ;
#25267=EDGE_CURVE ( 'NONE', #63618, #78225, #88302, .T. ) ;
#25280=EDGE_CURVE ( 'NONE', #77074, #76783, #67834, .T. ) ;
#25281=LINE ( 'NONE', #24405, #75387 ) ;
#25311=EDGE_LOOP ( 'NONE', ( #20406, #8930, #19570, #16120 ) ) ;
#25369=LINE ( 'NONE', #12646, #83285 ) ;
#25373=CARTESIAN_POINT ( 'NONE',  ( 122.2221484686745470, -111.9799080603168022, -11.78219314458175937 ) ) ;
#25390=EDGE_CURVE ( 'NONE', #89450, #44698, #57055, .T. ) ;
#25396=VERTEX_POINT ( 'NONE', #34653 ) ;
#25397=CARTESIAN_POINT ( 'NONE',  ( 107.0667039024470313, -104.2784471599418197, -11.78219314458200984 ) ) ;
#25422=FACE_OUTER_BOUND ( 'NONE', #45293, .T. ) ;
#25444=CARTESIAN_POINT ( 'NONE',  ( 122.2189888861419433, -111.9861225405541347, -21.78219314458176825 ) ) ;
#25470=DIRECTION ( 'NONE',  ( 0.7759704746411385523, -0.6307692307692301936, 0.000000000000000000 ) ) ;
#25471=ORIENTED_EDGE ( 'NONE', *, *, #17389, .F. ) ;
#25496=ORIENTED_EDGE ( 'NONE', *, *, #5174, .F. ) ;
#25504=CARTESIAN_POINT ( 'NONE',  ( 68.36158985427030643, -82.61730200034398308, 247.4783998280180128 ) ) ;
#25508=PLANE ( 'NONE',  #1141 ) ;
#25509=ORIENTED_EDGE ( 'NONE', *, *, #8692, .T. ) ;
#25510=FACE_OUTER_BOUND ( 'NONE', #80749, .T. ) ;
#25546=AXIS2_PLACEMENT_3D ( 'NONE', #9513, #38543, #36774 ) ;
#25559=CARTESIAN_POINT ( 'NONE',  ( 143.0667039024470455, -124.7784471599409102, 55.21780685541800437 ) ) ;
#25563=CARTESIAN_POINT ( 'NONE',  ( 144.5667039024470455, -123.2784471599409102, 55.21780685541800437 ) ) ;
#25565=B_SPLINE_SURFACE_WITH_KNOTS ( 'NONE', 3, 3, ( 
 ( #13262, #26439, #19181, #5560 ),
 ( #75037, #40950, #6441, #34135 ),
 ( #48646, #89569, #62291, #55456 ),
 ( #27328, #20531, #48199, #75932 ),
 ( #33252, #13704, #41391, #6885 ),
 ( #12824, #12363, #34587, #77 ),
 ( #27775, #83209, #76378, #14157 ) ),
 .UNSPECIFIED., .F., .F., .F.,
 ( 4, 1, 1, 1, 4 ),
 ( 4, 4 ),
 ( -0.0004313335404373049866, 0.2857142857142860315, 0.5714285714285709528, 0.8571428571428569843, 1.000431333540440004 ),
 ( 0.08686432420026919676, 1.000431333540440004 ),
 .UNSPECIFIED. ) ;
#25597=ORIENTED_EDGE ( 'NONE', *, *, #19629, .F. ) ;
#25601=LINE ( 'NONE', #31074, #63216 ) ;
#25606=EDGE_CURVE ( 'NONE', #34621, #87491, #41034, .T. ) ;
#25632=FACE_OUTER_BOUND ( 'NONE', #22655, .T. ) ;
#25634=EDGE_LOOP ( 'NONE', ( #77671, #46340, #86048, #3528 ) ) ;
#25644=ADVANCED_FACE ( 'NONE', ( #85962 ), #2834, .F. ) ;
#25649=EDGE_LOOP ( 'NONE', ( #69163, #15952, #58158, #38879, #8570 ) ) ;
#25650=ORIENTED_EDGE ( 'NONE', *, *, #47951, .T. ) ;
#25699=CIRCLE ( 'NONE', #3918, 4.500000000000003553 ) ;
#25715=CARTESIAN_POINT ( 'NONE',  ( 106.5667039024470171, -94.77844715994206126, -19.78219314458232247 ) ) ;
#25724=ORIENTED_EDGE ( 'NONE', *, *, #10017, .F. ) ;
#25726=LINE ( 'NONE', #62033, #59148 ) ;
#25736=LINE ( 'NONE', #18925, #83023 ) ;
#25750=DIRECTION ( 'NONE',  ( 3.100000000000000258E-29, -3.100000000000000044E-14, -1.000000000000000000 ) ) ;
#25753=AXIS2_PLACEMENT_3D ( 'NONE', #17725, #87215, #38163 ) ;
#25757=ORIENTED_EDGE ( 'NONE', *, *, #6429, .T. ) ;
#25758=VERTEX_POINT ( 'NONE', #45914 ) ;
#25762=CARTESIAN_POINT ( 'NONE',  ( 118.2946795739112957, -118.1912118068161703, -9.274842254010202680 ) ) ;
#25789=DIRECTION ( 'NONE',  ( 0.7071067811865453523, 0.7071067811865496822, 0.000000000000000000 ) ) ;
#25811=FACE_OUTER_BOUND ( 'NONE', #74228, .T. ) ;
#25814=VERTEX_POINT ( 'NONE', #6846 ) ;
#25821=ORIENTED_EDGE ( 'NONE', *, *, #60881, .F. ) ;
#25822=ADVANCED_FACE ( 'NONE', ( #68187 ), #40910, .T. ) ;
#25836=ADVANCED_FACE ( 'NONE', ( #19137 ), #41346, .F. ) ;
#25837=AXIS2_PLACEMENT_3D ( 'NONE', #67283, #74111, #11892 ) ;
#25840=DIRECTION ( 'NONE',  ( -1.000000000000000000, -1.181088324069315053E-15, 0.000000000000000000 ) ) ;
#25844=DIRECTION ( 'NONE',  ( -0.8660254037844392627, 0.4999999999999990008, -1.549999999999999706E-14 ) ) ;
#25845=CARTESIAN_POINT ( 'NONE',  ( 121.3178890780284291, -95.01002112898673602, -19.18411693322930134 ) ) ;
#25847=CARTESIAN_POINT ( 'NONE',  ( 107.0667039024470313, -119.4690460831833150, -11.78219314458153733 ) ) ;
#25865=CIRCLE ( 'NONE', #18596, 3.499999999999996003 ) ;
#25867=ORIENTED_EDGE ( 'NONE', *, *, #48383, .T. ) ;
#25871=EDGE_LOOP ( 'NONE', ( #84897, #56928, #6234, #2203 ) ) ;
#25883=VECTOR ( 'NONE', #47520, 1000.000000000000000 ) ;
#25886=EDGE_CURVE ( 'NONE', #82398, #43244, #54069, .T. ) ;
#25890=AXIS2_PLACEMENT_3D ( 'NONE', #14320, #672, #2030 ) ;
#25895=CIRCLE ( 'NONE', #76672, 11.49999999999999645 ) ;
#25908=EDGE_CURVE ( 'NONE', #35863, #88126, #62252, .T. ) ;
#25914=PLANE ( 'NONE',  #25233 ) ;
#25923=CARTESIAN_POINT ( 'NONE',  ( 92.91125933621934507, -113.6057974291317691, -21.78219314458173983 ) ) ;
#25959=CARTESIAN_POINT ( 'NONE',  ( 68.54895288615315962, -132.5647336068149684, 247.4783998280180128 ) ) ;
#25970=EDGE_CURVE ( 'NONE', #49424, #71630, #44012, .T. ) ;
#25981=CARTESIAN_POINT ( 'NONE',  ( 146.6607710079033779, -137.6835511433035037, 246.9874215757600098 ) ) ;
#26023=CARTESIAN_POINT ( 'NONE',  ( 144.5667039024470171, -90.27844715994091018, 45.21780685541799727 ) ) ;
#26035=CARTESIAN_POINT ( 'NONE',  ( 67.06681736700808472, -67.87844715931913697, 245.5130139978070076 ) ) ;
#26049=ADVANCED_FACE ( 'NONE', ( #69977 ), #77428, .T. ) ;
#26062=CIRCLE ( 'NONE', #8704, 3.499999999999996003 ) ;
#26066=DIRECTION ( 'NONE',  ( 1.000000000000000078E-15, -1.000000000000000000, 0.000000000000000000 ) ) ;
#26102=FACE_OUTER_BOUND ( 'NONE', #44851, .T. ) ;
#26122=AXIS2_PLACEMENT_3D ( 'NONE', #16425, #72284, #10492 ) ;
#26127=CARTESIAN_POINT ( 'NONE',  ( 107.0667039024470313, -104.2784471599420755, -19.78219314458201694 ) ) ;
#26138=ORIENTED_EDGE ( 'NONE', *, *, #18842, .T. ) ;
#26154=EDGE_CURVE ( 'NONE', #48853, #47787, #44481, .T. ) ;
#26156=DIRECTION ( 'NONE',  ( 0.000000000000000000, 0.000000000000000000, 1.000000000000000000 ) ) ;
#26169=PLANE ( 'NONE',  #19982 ) ;
#26174=ORIENTED_EDGE ( 'NONE', *, *, #7930, .T. ) ;
#26181=DIRECTION ( 'NONE',  ( -1.000000000000000078E-15, 1.000000000000000000, 0.000000000000000000 ) ) ;
#26186=DIRECTION ( 'NONE',  ( 0.8660254037844392627, -0.4999999999999990008, 1.549999999999999706E-14 ) ) ;
#26192=CARTESIAN_POINT ( 'NONE',  ( 146.0667039024470171, -86.77844715994089597, 45.21780685541799727 ) ) ;
#26215=CARTESIAN_POINT ( 'NONE',  ( 145.4416927396864878, -139.3034583227001804, 245.6607614918409865 ) ) ;
#26222=PLANE ( 'NONE',  #66009 ) ;
#26230=VECTOR ( 'NONE', #81976, 1000.000000000000000 ) ;
#26234=VECTOR ( 'NONE', #80295, 1000.000000000000000 ) ;
#26236=VERTEX_POINT ( 'NONE', #58994 ) ;
#26248=ORIENTED_EDGE ( 'NONE', *, *, #77603, .T. ) ;
#26252=AXIS2_PLACEMENT_3D ( 'NONE', #18051, #73915, #58485 ) ;
#26259=DIRECTION ( 'NONE',  ( -0.1250000000000000278, -0.9921567416492215186, 3.035766082959410522E-14 ) ) ;
#26284=LINE ( 'NONE', #74889, #83747 ) ;
#26292=EDGE_LOOP ( 'NONE', ( #32056, #55291, #5115, #55409 ) ) ;
#26293=DIRECTION ( 'NONE',  ( -1.000000000000000000, -1.000000000000000078E-15, 0.000000000000000000 ) ) ;
#26295=ADVANCED_FACE ( 'NONE', ( #85859 ), #58125, .F. ) ;
#26299=CARTESIAN_POINT ( 'NONE',  ( 107.0667039024470313, -104.2784471599420755, -19.78219314458201694 ) ) ;
#26302=EDGE_CURVE ( 'NONE', #83222, #84863, #80372, .T. ) ;
#26317=VERTEX_POINT ( 'NONE', #40800 ) ;
#26322=ADVANCED_FACE ( 'NONE', ( #60795 ), #46708, .F. ) ;
#26325=DIRECTION ( 'NONE',  ( 0.000000000000000000, 0.000000000000000000, 1.000000000000000000 ) ) ;
#26340=VECTOR ( 'NONE', #70667, 1000.000000000000000 ) ;
#26346=VERTEX_POINT ( 'NONE', #83063 ) ;
#26353=VECTOR ( 'NONE', #79063, 1000.000000000000000 ) ;
#26367=DIRECTION ( 'NONE',  ( -1.000000000000000000, -8.163404592832032979E-16, 0.000000000000000000 ) ) ;
#26380=CARTESIAN_POINT ( 'NONE',  ( 143.0667039024470455, -124.7784471599409102, 45.21780685541799727 ) ) ;
#26395=EDGE_LOOP ( 'NONE', ( #153, #76034, #4927, #20796 ) ) ;
#26400=CARTESIAN_POINT ( 'NONE',  ( 107.5667039024470171, -94.77844715994206126, -19.78219314458232247 ) ) ;
#26431=DIRECTION ( 'NONE',  ( 3.114895971316861016E-16, -1.000000000000000000, 0.000000000000000000 ) ) ;
#26439=CARTESIAN_POINT ( 'NONE',  ( 139.3670900352978208, -74.85671702932823734, 248.3919668373590071 ) ) ;
#26514=CARTESIAN_POINT ( 'NONE',  ( 78.56670390244704549, -118.2784471599409812, 51.21780685541800437 ) ) ;
#26524=DIRECTION ( 'NONE',  ( -3.100000000000000258E-29, 3.100000000000000044E-14, 1.000000000000000000 ) ) ;
#26527=CIRCLE ( 'NONE', #6242, 32.50000000000001421 ) ;
#26539=CARTESIAN_POINT ( 'NONE',  ( 106.5667039024470171, -94.77844715994206126, -19.78219314458232247 ) ) ;
#26542=CARTESIAN_POINT ( 'NONE',  ( 107.0667039024470313, -104.2784471599413791, 2.217806855418003043 ) ) ;
#26555=CARTESIAN_POINT ( 'NONE',  ( 151.0667039024469886, -67.87844715994090450, 155.2178068554179902 ) ) ;
#26556=DIRECTION ( 'NONE',  ( -3.100000000000000258E-29, 3.100000000000000044E-14, 1.000000000000000000 ) ) ;
#26570=DIRECTION ( 'NONE',  ( -0.7118375500353263385, -0.7021341844407537058, 0.01717234402817945094 ) ) ;
#26588=CARTESIAN_POINT ( 'NONE',  ( 144.1851062731161619, -138.0565978134347063, 247.6574394623689841 ) ) ;
#26591=CARTESIAN_POINT ( 'NONE',  ( 108.0667039024470455, -121.2010968907525239, -21.78219314458149114 ) ) ;
#26597=LINE ( 'NONE', #37675, #27513 ) ;
#26602=ADVANCED_FACE ( 'NONE', ( #66157 ), #78927, .F. ) ;
#26621=CARTESIAN_POINT ( 'NONE',  ( 53.06670390244699576, -67.87844715994100397, 55.21780685541800437 ) ) ;
#26645=CARTESIAN_POINT ( 'NONE',  ( 77.06670390244701707, -90.27844715994098124, 51.21780685541800437 ) ) ;
#26657=CARTESIAN_POINT ( 'NONE',  ( 77.10147176826316695, -139.5747906685508894, 247.4459311921649771 ) ) ;
#26685=ORIENTED_EDGE ( 'NONE', *, *, #33713, .T. ) ;
#26687=VERTEX_POINT ( 'NONE', #46601 ) ;
#26698=DIRECTION ( 'NONE',  ( -0.000000000000000000, -0.000000000000000000, -1.000000000000000000 ) ) ;
#26701=ORIENTED_EDGE ( 'NONE', *, *, #77192, .T. ) ;
#26704=ORIENTED_EDGE ( 'NONE', *, *, #32436, .T. ) ;
#26709=EDGE_CURVE ( 'NONE', #25248, #74974, #79787, .T. ) ;
#26736=DIRECTION ( 'NONE',  ( -3.100000000000000258E-29, 3.100000000000000044E-14, 1.000000000000000000 ) ) ;
#26749=CARTESIAN_POINT ( 'NONE',  ( 107.0667039024470313, -104.2784471599412086, 7.717806855417980394 ) ) ;
#26771=FACE_OUTER_BOUND ( 'NONE', #86126, .T. ) ;
#26784=ADVANCED_FACE ( 'NONE', ( #46149 ), #43255, .T. ) ;
#26798=ORIENTED_EDGE ( 'NONE', *, *, #64525, .F. ) ;
#26800=EDGE_CURVE ( 'NONE', #75315, #17260, #71447, .T. ) ;
#26803=CARTESIAN_POINT ( 'NONE',  ( 97.81670390244700286, -68.87844715994096134, 222.2178068554179902 ) ) ;
#26818=CARTESIAN_POINT ( 'NONE',  ( 151.0667039024469886, -79.67844715994088745, 85.21780685541799016 ) ) ;
#26830=AXIS2_PLACEMENT_3D ( 'NONE', #84518, #35429, #36343 ) ;
#26843=EDGE_CURVE ( 'NONE', #18276, #29468, #29209, .T. ) ;
#26857=CIRCLE ( 'NONE', #32620, 8.999999999999994671 ) ;
#26866=ORIENTED_EDGE ( 'NONE', *, *, #20264, .F. ) ;
#26869=VECTOR ( 'NONE', #44705, 1000.000000000000000 ) ;
#26872=ORIENTED_EDGE ( 'NONE', *, *, #55739, .T. ) ;
#26878=( BOUNDED_CURVE ( )  B_SPLINE_CURVE ( 2, ( #66579, #17985, #4373 ),
 .UNSPECIFIED., .F., .F. ) 
 B_SPLINE_CURVE_WITH_KNOTS ( ( 3, 3 ),
 ( 0.01169420784674130021, 0.5170228498526558969 ),
 .UNSPECIFIED. ) 
 CURVE ( )  GEOMETRIC_REPRESENTATION_ITEM ( )  RATIONAL_B_SPLINE_CURVE ( ( 1.000420656333759872, 1.009299002520659849, 1.000000000000000000 ) ) 
 REPRESENTATION_ITEM ( '' )  );
#26882=EDGE_CURVE ( 'NONE', #36478, #33876, #16920, .T. ) ;
#26891=CARTESIAN_POINT ( 'NONE',  ( 114.2313622454167046, -107.8376143137176655, -19.78219314458190681 ) ) ;
#26905=DIRECTION ( 'NONE',  ( -1.000000000000000000, -1.000000000000000078E-15, 0.000000000000000000 ) ) ;
#26922=DIRECTION ( 'NONE',  ( -3.100000000000000258E-29, 3.100000000000000044E-14, 1.000000000000000000 ) ) ;
#26949=ORIENTED_EDGE ( 'NONE', *, *, #56646, .T. ) ;
#26959=ADVANCED_FACE ( 'NONE', ( #25510 ), #51850, .F. ) ;
#26985=EDGE_LOOP ( 'NONE', ( #18079, #38546 ) ) ;
#26991=AXIS2_PLACEMENT_3D ( 'NONE', #58973, #66238, #51265 ) ;
#27015=ORIENTED_EDGE ( 'NONE', *, *, #47530, .F. ) ;
#27018=DIRECTION ( 'NONE',  ( 0.1250000000000000278, 0.9921567416492215186, -3.035766082959410522E-14 ) ) ;
#27024=CARTESIAN_POINT ( 'NONE',  ( 122.2221484686747459, -111.8737466215628729, -21.78219314458179667 ) ) ;
#27034=DIRECTION ( 'NONE',  ( 0.000000000000000000, 0.000000000000000000, -1.000000000000000000 ) ) ;
#27045=EDGE_LOOP ( 'NONE', ( #55891, #24515, #43715, #8853 ) ) ;
#27050=CIRCLE ( 'NONE', #73465, 3.999999999999998224 ) ;
#27066=CARTESIAN_POINT ( 'NONE',  ( 147.0667039024469886, -67.87844715994090450, 247.2178068554179902 ) ) ;
#27071=ORIENTED_EDGE ( 'NONE', *, *, #19328, .T. ) ;
#27073=DIRECTION ( 'NONE',  ( 1.000000000000000078E-15, -1.000000000000000000, 0.000000000000000000 ) ) ;
#27087=CYLINDRICAL_SURFACE ( 'NONE', #11945, 3.500000000000003109 ) ;
#27108=EDGE_CURVE ( 'NONE', #59214, #17803, #30547, .T. ) ;
#27114=CARTESIAN_POINT ( 'NONE',  ( 107.9747653995834753, -121.2541776101292186, -11.78219314458148226 ) ) ;
#27115=CARTESIAN_POINT ( 'NONE',  ( 145.3811004230890376, -139.2461875257762358, 246.2327794654912907 ) ) ;
#27119=ORIENTED_EDGE ( 'NONE', *, *, #9983, .F. ) ;
#27151=DIRECTION ( 'NONE',  ( -3.100000000000000258E-29, 3.100000000000000044E-14, 1.000000000000000000 ) ) ;
#27176=CARTESIAN_POINT ( 'NONE',  ( 115.0439452383991892, -99.09543445804983719, -19.78219314458218392 ) ) ;
#27182=FACE_OUTER_BOUND ( 'NONE', #54685, .T. ) ;
#27214=LINE ( 'NONE', #41276, #51480 ) ;
#27218=ORIENTED_EDGE ( 'NONE', *, *, #29582, .T. ) ;
#27220=CARTESIAN_POINT ( 'NONE',  ( 71.06670390244705970, -124.7784471599409812, 55.21780685541800437 ) ) ;
#27225=ADVANCED_FACE ( 'NONE', ( #49070 ), #42263, .F. ) ;
#27238=CYLINDRICAL_SURFACE ( 'NONE', #70575, 2.999999999999975131 ) ;
#27255=CARTESIAN_POINT ( 'NONE',  ( 106.0667039024470455, -121.2010968907522113, -11.78219314458148226 ) ) ;
#27260=DIRECTION ( 'NONE',  ( -3.100000000000000258E-29, 3.100000000000000044E-14, 1.000000000000000000 ) ) ;
#27266=CARTESIAN_POINT ( 'NONE',  ( 121.2221484686747459, -113.6057974291317549, -21.78219314458173983 ) ) ;
#27286=VERTEX_POINT ( 'NONE', #35451 ) ;
#27290=EDGE_CURVE ( 'NONE', #18666, #65691, #63167, .T. ) ;
#27296=ORIENTED_EDGE ( 'NONE', *, *, #16301, .F. ) ;
#27318=CARTESIAN_POINT ( 'NONE',  ( 160.0667039024470171, -79.67844715994088745, 55.21780685541800437 ) ) ;
#27327=CARTESIAN_POINT ( 'NONE',  ( 107.0667039024470313, -104.2784471599413934, 2.217806855418003043 ) ) ;
#27328=CARTESIAN_POINT ( 'NONE',  ( 146.0392919387902282, -109.2859103858200029, 247.4783998280190076 ) ) ;
#27356=PLANE ( 'NONE',  #3834 ) ;
#27367=AXIS2_PLACEMENT_3D ( 'NONE', #76827, #43635, #56365 ) ;
#27390=AXIS2_PLACEMENT_3D ( 'NONE', #32636, #53503, #24941 ) ;
#27404=EDGE_CURVE ( 'NONE', #86337, #11051, #53721, .T. ) ;
#27419=CARTESIAN_POINT ( 'NONE',  ( 147.0667039024470171, -79.67844715994090166, 222.2178068554179902 ) ) ;
#27441=CARTESIAN_POINT ( 'NONE',  ( 147.0667039024469886, -67.87844715994090450, 222.2178068554179902 ) ) ;
#27442=VERTEX_POINT ( 'NONE', #3194 ) ;
#27459=CARTESIAN_POINT ( 'NONE',  ( 71.06670390244705970, -118.2784471599409812, 222.2178068554179902 ) ) ;
#27461=AXIS2_PLACEMENT_3D ( 'NONE', #79489, #17251, #78155 ) ;
#27466=EDGE_CURVE ( 'NONE', #59958, #44336, #65414, .T. ) ;
#27478=LINE ( 'NONE', #33399, #30106 ) ;
#27481=EDGE_LOOP ( 'NONE', ( #35706, #29732, #39933, #28410 ) ) ;
#27488=AXIS2_PLACEMENT_3D ( 'NONE', #40493, #25071, #33682 ) ;
#27494=AXIS2_PLACEMENT_3D ( 'NONE', #82483, #11632, #81136 ) ;
#27513=VECTOR ( 'NONE', #86271, 1000.000000000000000 ) ;
#27517=VECTOR ( 'NONE', #46859, 1000.000000000000114 ) ;
#27520=DIRECTION ( 'NONE',  ( -0.4999999999999931166, -0.8660254037844425934, 2.684678751731770391E-14 ) ) ;
#27521=CARTESIAN_POINT ( 'NONE',  ( 99.06670390244704549, -104.2784471599421181, -19.78219314458201694 ) ) ;
#27523=PLANE ( 'NONE',  #56534 ) ;
#27524=DIRECTION ( 'NONE',  ( -1.000000000000000000, -1.541976423090496028E-15, 0.000000000000000000 ) ) ;
#27551=EDGE_CURVE ( 'NONE', #66630, #34986, #59018, .T. ) ;
#27559=CARTESIAN_POINT ( 'NONE',  ( 92.81551872686561921, -95.01002112898652285, -11.78219314458228695 ) ) ;
#27571=CARTESIAN_POINT ( 'NONE',  ( 70.56670390244700286, -67.87844715994098976, 222.2178068554179902 ) ) ;
#27599=CARTESIAN_POINT ( 'NONE',  ( 97.06670390244703128, -109.9573555057414609, 7.717806855418146483 ) ) ;
#27647=DIRECTION ( 'NONE',  ( -1.000000000000000000, -8.163404592832032979E-16, 0.000000000000000000 ) ) ;
#27652=PLANE ( 'NONE',  #77155 ) ;
#27658=VECTOR ( 'NONE', #75656, 1000.000000000000000 ) ;
#27660=VECTOR ( 'NONE', #66980, 1000.000000000000000 ) ;
#27671=CIRCLE ( 'NONE', #78462, 3.499999999999996003 ) ;
#27673=VERTEX_POINT ( 'NONE', #5425 ) ;
#27685=VERTEX_POINT ( 'NONE', #5878 ) ;
#27693=DIRECTION ( 'NONE',  ( -1.000000000000000000, -8.163404592832032979E-16, 0.000000000000000000 ) ) ;
#27714=CARTESIAN_POINT ( 'NONE',  ( 70.06670417066790435, -71.37844715994097555, 222.2178068554179902 ) ) ;
#27715=ORIENTED_EDGE ( 'NONE', *, *, #39623, .T. ) ;
#27723=CARTESIAN_POINT ( 'NONE',  ( 106.5667039024470171, -96.29408744860641889, -19.78219314458226563 ) ) ;
#27729=ORIENTED_EDGE ( 'NONE', *, *, #58094, .F. ) ;
#27734=AXIS2_PLACEMENT_3D ( 'NONE', #5043, #32741, #86826 ) ;
#27740=EDGE_CURVE ( 'NONE', #32183, #638, #56727, .T. ) ;
#27747=ORIENTED_EDGE ( 'NONE', *, *, #20963, .T. ) ;
#27748=VECTOR ( 'NONE', #37964, 1000.000000000000000 ) ;
#27758=EDGE_CURVE ( 'NONE', #26346, #31292, #14018, .T. ) ;
#27775=CARTESIAN_POINT ( 'NONE',  ( 145.3578527754884533, -139.1541231917475727, 247.4783998280190076 ) ) ;
#27808=CARTESIAN_POINT ( 'NONE',  ( 116.0667040365575104, -83.77844715994093860, 222.2178068554179902 ) ) ;
#27830=DIRECTION ( 'NONE',  ( -0.7759704746411383303, 0.6307692307692303046, 0.000000000000000000 ) ) ;
#27846=ORIENTED_EDGE ( 'NONE', *, *, #8590, .T. ) ;
#27877=PLANE ( 'NONE',  #49332 ) ;
#27879=DIRECTION ( 'NONE',  ( -1.000000000000000000, -1.541976423090496028E-15, 0.000000000000000000 ) ) ;
#27880=VECTOR ( 'NONE', #49881, 1000.000000000000000 ) ;
#27883=VERTEX_POINT ( 'NONE', #64856 ) ;
#27886=AXIS2_PLACEMENT_3D ( 'NONE', #75242, #88429, #5756 ) ;
#27900=ORIENTED_EDGE ( 'NONE', *, *, #47771, .F. ) ;
#27901=ORIENTED_EDGE ( 'NONE', *, *, #46886, .T. ) ;
#27912=CARTESIAN_POINT ( 'NONE',  ( 68.47164110671278081, -69.21472957910711443, 247.4213243805862987 ) ) ;
#27927=ORIENTED_EDGE ( 'NONE', *, *, #89170, .T. ) ;
#27936=ORIENTED_EDGE ( 'NONE', *, *, #71159, .F. ) ;
#27940=ORIENTED_EDGE ( 'NONE', *, *, #78168, .T. ) ;
#27956=EDGE_LOOP ( 'NONE', ( #83127, #57518, #17546, #41129 ) ) ;
#28001=CARTESIAN_POINT ( 'NONE',  ( 145.1692508678690103, -139.0365492197044546, 246.8416124795636222 ) ) ;
#28036=CARTESIAN_POINT ( 'NONE',  ( 103.8797721312301405, -101.8611209747514010, -19.78219314458209865 ) ) ;
#28038=EDGE_CURVE ( 'NONE', #78082, #78823, #48025, .T. ) ;
#28069=CARTESIAN_POINT ( 'NONE',  ( 115.5439452383992176, -108.5954344580491551, 2.217806855418142042 ) ) ;
#28076=LINE ( 'NONE', #76238, #80476 ) ;
#28081=VERTEX_POINT ( 'NONE', #67983 ) ;
#28086=DIRECTION ( 'NONE',  ( -1.000000000000000000, -1.541976423090496028E-15, 0.000000000000000000 ) ) ;
#28125=CARTESIAN_POINT ( 'NONE',  ( 92.91125933621933086, -94.95109689075242443, -19.26696060647628528 ) ) ;
#28129=EDGE_CURVE ( 'NONE', #67885, #14739, #46598, .T. ) ;
#28160=LINE ( 'NONE', #42234, #32622 ) ;
#28194=( BOUNDED_CURVE ( )  B_SPLINE_CURVE ( 3, ( #53564, #81333, #28464, #77526 ),
 .UNSPECIFIED., .F., .T. ) 
 B_SPLINE_CURVE_WITH_KNOTS ( ( 4, 4 ),
 ( 0.2392026736790540120, 0.2483601390811745191 ),
 .UNSPECIFIED. ) 
 CURVE ( )  GEOMETRIC_REPRESENTATION_ITEM ( )  RATIONAL_B_SPLINE_CURVE ( ( 1.000000000000000000, 0.9999930117478262881, 0.9999930117478262881, 1.000000000000000000 ) ) 
 REPRESENTATION_ITEM ( '' )  );
#28195=VECTOR ( 'NONE', #63501, 1000.000000000000000 ) ;
#28196=DIRECTION ( 'NONE',  ( -1.000000000000000000, -1.000000000000000078E-15, 0.000000000000000000 ) ) ;
#28213=VECTOR ( 'NONE', #4445, 1000.000000000000000 ) ;
#28215=CARTESIAN_POINT ( 'NONE',  ( 59.56670390244699576, -67.87844715994098976, 120.2178068554179902 ) ) ;
#28226=PLANE ( 'NONE',  #31748 ) ;
#28238=LINE ( 'NONE', #998, #12747 ) ;
#28247=EDGE_CURVE ( 'NONE', #12987, #74492, #14374, .T. ) ;
#28266=DIRECTION ( 'NONE',  ( 0.000000000000000000, 0.000000000000000000, -1.000000000000000000 ) ) ;
#28269=VECTOR ( 'NONE', #79756, 1000.000000000000000 ) ;
#28276=AXIS2_PLACEMENT_3D ( 'NONE', #22823, #36883, #79576 ) ;
#28279=AXIS2_PLACEMENT_3D ( 'NONE', #9903, #47523, #68443 ) ;
#28307=CARTESIAN_POINT ( 'NONE',  ( 107.9678037105606450, -121.2545485715091047, -11.78219314458148226 ) ) ;
#28309=CARTESIAN_POINT ( 'NONE',  ( 105.1589286322275143, -131.7784471599410097, 250.2178068554179902 ) ) ;
#28313=CARTESIAN_POINT ( 'NONE',  ( 78.56670390244701707, -90.27844715994098124, 45.21780685541799727 ) ) ;
#28317=CIRCLE ( 'NONE', #39926, 17.00000000000000000 ) ;
#28342=CARTESIAN_POINT ( 'NONE',  ( 134.4101120871804653, -107.6623471058698414, 250.2178068554180470 ) ) ;
#28348=DIRECTION ( 'NONE',  ( -3.100000000000000258E-29, 3.100000000000000044E-14, 1.000000000000000000 ) ) ;
#28352=CARTESIAN_POINT ( 'NONE',  ( 119.2563820928105400, -114.7407331754008055, -21.02845593540893532 ) ) ;
#28354=CARTESIAN_POINT ( 'NONE',  ( 67.06888395500608624, -67.87985678217047791, 245.5863101313805146 ) ) ;
#28360=TOROIDAL_SURFACE ( 'NONE', #811, 29.50000000000000000, 1.500000000000000000 ) ;
#28364=CARTESIAN_POINT ( 'NONE',  ( 144.0667039024470455, -124.7784471599409102, 55.21780685541800437 ) ) ;
#28371=VERTEX_POINT ( 'NONE', #57024 ) ;
#28374=ADVANCED_FACE ( 'NONE', ( #62506 ), #65632, .F. ) ;
#28377=ORIENTED_EDGE ( 'NONE', *, *, #29802, .F. ) ;
#28382=CARTESIAN_POINT ( 'NONE',  ( 132.2857443282840393, -124.7784471599409102, 45.21780685541799727 ) ) ;
#28399=DIRECTION ( 'NONE',  ( 0.000000000000000000, 0.000000000000000000, -1.000000000000000000 ) ) ;
#28410=ORIENTED_EDGE ( 'NONE', *, *, #84667, .F. ) ;
#28418=DIRECTION ( 'NONE',  ( -3.100000000000000258E-29, 3.100000000000000044E-14, 1.000000000000000000 ) ) ;
#28421=DIRECTION ( 'NONE',  ( 0.000000000000000000, 0.000000000000000000, -1.000000000000000000 ) ) ;
#28424=DIRECTION ( 'NONE',  ( 1.000000000000000000, 1.000000000000000078E-15, 0.000000000000000000 ) ) ;
#28434=DIRECTION ( 'NONE',  ( -1.000000000000000000, -1.734723475976808672E-15, 0.000000000000000000 ) ) ;
#28464=CARTESIAN_POINT ( 'NONE',  ( 147.0666650806933262, -67.87844715994090450, 245.5060119364703439 ) ) ;
#28483=ORIENTED_EDGE ( 'NONE', *, *, #69511, .F. ) ;
#28484=EDGE_LOOP ( 'NONE', ( #21799, #12269, #84271, #20784 ) ) ;
#28504=LINE ( 'NONE', #1722, #7049 ) ;
#28537=ADVANCED_FACE ( 'NONE', ( #12020 ), #33796, .F. ) ;
#28553=CARTESIAN_POINT ( 'NONE',  ( 121.3178890780284291, -95.01002112898679286, -21.78219314458229405 ) ) ;
#28560=AXIS2_PLACEMENT_3D ( 'NONE', #88863, #19811, #4838 ) ;
#28603=ORIENTED_EDGE ( 'NONE', *, *, #134, .F. ) ;
#28611=EDGE_LOOP ( 'NONE', ( #62909, #69008, #9365, #72642, #21291, #48648 ) ) ;
#28639=ORIENTED_EDGE ( 'NONE', *, *, #22302, .T. ) ;
#28646=DIRECTION ( 'NONE',  ( 3.100000000000000258E-29, -3.100000000000000044E-14, -1.000000000000000000 ) ) ;
#28661=EDGE_CURVE ( 'NONE', #48200, #88900, #3197, .T. ) ;
#28662=CARTESIAN_POINT ( 'NONE',  ( 151.0667039024469886, -67.87844715994090450, 120.2178068554179902 ) ) ;
#28664=PLANE ( 'NONE',  #69031 ) ;
#28665=ADVANCED_FACE ( 'NONE', ( #36496 ), #62391, .T. ) ;
#28671=DIRECTION ( 'NONE',  ( -1.000000000000000000, -1.181088324069315053E-15, 0.000000000000000000 ) ) ;
#28675=VECTOR ( 'NONE', #2399, 999.9999999999998863 ) ;
#28679=CARTESIAN_POINT ( 'NONE',  ( 52.06670390244699576, -67.87844715994100397, 222.2178068554179902 ) ) ;
#28687=EDGE_CURVE ( 'NONE', #74740, #61361, #35932, .T. ) ;
#28715=EDGE_CURVE ( 'NONE', #34986, #49377, #85103, .T. ) ;
#28744=CARTESIAN_POINT ( 'NONE',  ( 116.3167039024470029, -67.87844715994093292, 222.2178068554179902 ) ) ;
#28755=DIRECTION ( 'NONE',  ( 1.000000000000000000, 1.000000000000000078E-15, 0.000000000000000000 ) ) ;
#28766=PRESENTATION_STYLE_ASSIGNMENT (( #15138 ) ) ;
#28770=CARTESIAN_POINT ( 'NONE',  ( 68.73724395117878316, -139.2608654268313728, 246.1571707801609250 ) ) ;
#28786=DIRECTION ( 'NONE',  ( 0.000000000000000000, 0.000000000000000000, 1.000000000000000000 ) ) ;
#28791=AXIS2_PLACEMENT_3D ( 'NONE', #87895, #80644, #81989 ) ;
#28815=CARTESIAN_POINT ( 'NONE',  ( 129.5675368918763581, -120.1789271773120333, 250.2178068554180470 ) ) ;
#28819=DIRECTION ( 'NONE',  ( -1.000000000000000000, -1.541976423090496028E-15, 0.000000000000000000 ) ) ;
#28823=CARTESIAN_POINT ( 'NONE',  ( 67.49017891634400712, -68.28604453786587669, 246.7253416711091631 ) ) ;
#28827=ORIENTED_EDGE ( 'NONE', *, *, #23703, .T. ) ;
#28833=EDGE_CURVE ( 'NONE', #21942, #29924, #1769, .T. ) ;
#28863=CARTESIAN_POINT ( 'NONE',  ( 161.0667039024469886, -67.87844715994089029, 222.2178068554179902 ) ) ;
#28900=CARTESIAN_POINT ( 'NONE',  ( 125.5177273812784762, -137.6784471599409301, 55.21780685541800437 ) ) ;
#28905=CARTESIAN_POINT ( 'NONE',  ( 69.95929469538076262, -138.0461895383713795, 247.6591799766680140 ) ) ;
#28907=ORIENTED_EDGE ( 'NONE', *, *, #25908, .F. ) ;
#28916=FACE_OUTER_BOUND ( 'NONE', #10478, .T. ) ;
#28920=ORIENTED_EDGE ( 'NONE', *, *, #21249, .T. ) ;
#28925=CARTESIAN_POINT ( 'NONE',  ( 107.0667039024470313, -104.2784471599413934, 2.217806855418003043 ) ) ;
#28944=DIRECTION ( 'NONE',  ( -3.100000000000000258E-29, 3.100000000000000044E-14, 1.000000000000000000 ) ) ;
#28952=MECHANICAL_DESIGN_GEOMETRIC_PRESENTATION_REPRESENTATION('',(#36206),#79729);
#28982=CARTESIAN_POINT ( 'NONE',  ( 108.0015156553065054, -87.31935934938634603, -19.21044887263853695 ) ) ;
#28990=VERTEX_POINT ( 'NONE', #62626 ) ;
#29003=CARTESIAN_POINT ( 'NONE',  ( 143.2522959336310748, -139.0102598546870922, 247.5112310255240118 ) ) ;
#29007=EDGE_LOOP ( 'NONE', ( #44279, #85190, #26866, #18879 ) ) ;
#29010=VERTEX_POINT ( 'NONE', #75371 ) ;
#29018=DIRECTION ( 'NONE',  ( 0.000000000000000000, 0.000000000000000000, 1.000000000000000000 ) ) ;
#29025=EDGE_LOOP ( 'NONE', ( #17107, #16671, #79533, #15247, #8632, #36162, #61950, #87600, #60836, #10087, #77111, #49341, #29456, #60644, #47829, #2011, #62405, #42914, #12058, #53098, #2010, #35767 ) ) ;
#29026=CARTESIAN_POINT ( 'NONE',  ( 95.56670390244703128, -104.2784471599411660, 17.71780685541799016 ) ) ;
#29029=( GEOMETRIC_REPRESENTATION_CONTEXT ( 3 ) GLOBAL_UNCERTAINTY_ASSIGNED_CONTEXT ( ( #44153 ) ) GLOBAL_UNIT_ASSIGNED_CONTEXT ( ( #50535, #14695, #63281 ) ) REPRESENTATION_CONTEXT ( 'NONE', 'WORKASPACE' ) );
#29049=LINE ( 'NONE', #37204, #58149 ) ;
#29076=CARTESIAN_POINT ( 'NONE',  ( 147.0667039024470739, -137.6784471599409017, 55.21780685541800437 ) ) ;
#29081=FACE_BOUND ( 'NONE', #48757, .T. ) ;
#29082=EDGE_LOOP ( 'NONE', ( #5040, #34309, #60953, #62619, #55673 ) ) ;
#29090=CARTESIAN_POINT ( 'NONE',  ( 107.0667039024470313, -104.2784471599420471, -19.18411693322902423 ) ) ;
#29111=CARTESIAN_POINT ( 'NONE',  ( 154.5667039024470171, -79.67844715994088745, 155.2178068554179902 ) ) ;
#29112=ORIENTED_EDGE ( 'NONE', *, *, #7776, .T. ) ;
#29114=DIRECTION ( 'NONE',  ( 0.000000000000000000, 0.000000000000000000, -1.000000000000000000 ) ) ;
#29131=AXIS2_PLACEMENT_3D ( 'NONE', #32310, #67285, #24619 ) ;
#29132=EDGE_LOOP ( 'NONE', ( #69508, #13170 ) ) ;
#29151=CARTESIAN_POINT ( 'NONE',  ( 147.0667039024470739, -137.6784471599409017, 245.4361138694860074 ) ) ;
#29168=DIRECTION ( 'NONE',  ( -0.4999999999999985567, -0.8660254037844395958, 2.602085213965200860E-14 ) ) ;
#29173=CYLINDRICAL_SURFACE ( 'NONE', #23606, 3.000000864267367895 ) ;
#29176=ORIENTED_EDGE ( 'NONE', *, *, #12782, .F. ) ;
#29180=DIRECTION ( 'NONE',  ( -3.100000000000000258E-29, 3.100000000000000044E-14, 1.000000000000000000 ) ) ;
#29185=DIRECTION ( 'NONE',  ( -1.000000000000000000, -1.206764157201257538E-15, 0.000000000000000000 ) ) ;
#29186=VERTEX_POINT ( 'NONE', #51218 ) ;
#29189=EDGE_CURVE ( 'NONE', #48853, #56759, #20632, .T. ) ;
#29193=EDGE_CURVE ( 'NONE', #34651, #58881, #2205, .T. ) ;
#29204=DIRECTION ( 'NONE',  ( 0.8660254037844382635, 0.5000000000000008882, -1.550000000000000022E-14 ) ) ;
#29209=LINE ( 'NONE', #71888, #11624 ) ;
#29221=CARTESIAN_POINT ( 'NONE',  ( 68.69165074297623619, -139.3035918984462000, 245.6745758308635175 ) ) ;
#29223=DIRECTION ( 'NONE',  ( 0.5000000000000015543, 0.8660254037844377084, -2.602085213965216006E-14 ) ) ;
#29224=CARTESIAN_POINT ( 'NONE',  ( 111.4303245704231244, -106.2204344580498372, -19.78219314458196010 ) ) ;
#29229=EDGE_CURVE ( 'NONE', #81211, #78112, #1758, .T. ) ;
#29240=DIRECTION ( 'NONE',  ( -3.100000000000000258E-29, 3.100000000000000044E-14, 1.000000000000000000 ) ) ;
#29258=ORIENTED_EDGE ( 'NONE', *, *, #40528, .T. ) ;
#29259=VECTOR ( 'NONE', #50661, 999.9999999999998863 ) ;
#29261=CARTESIAN_POINT ( 'NONE',  ( 132.1035770464691836, -92.77767617834375358, 250.2178068554180470 ) ) ;
#29269=CARTESIAN_POINT ( 'NONE',  ( 67.12633028470673935, -67.93405945762680176, 245.9787629646199036 ) ) ;
#29291=ADVANCED_FACE ( 'NONE', ( #79862 ), #52979, .T. ) ;
#29293=ORIENTED_EDGE ( 'NONE', *, *, #86196, .F. ) ;
#29327=EDGE_LOOP ( 'NONE', ( #27940, #4915, #74957, #62745 ) ) ;
#29335=CARTESIAN_POINT ( 'NONE',  ( 115.0439452383991892, -99.09543445804915507, 2.217806855417836509 ) ) ;
#29344=ORIENTED_EDGE ( 'NONE', *, *, #82344, .F. ) ;
#29353=DIRECTION ( 'NONE',  ( 0.000000000000000000, 0.000000000000000000, -1.000000000000000000 ) ) ;
#29365=B_SPLINE_CURVE_WITH_KNOTS ( 'NONE', 3,
 ( #82589, #20347, #48018, #13525, #34403, #46528 ),
 .UNSPECIFIED., .F., .F.,
 ( 4, 2, 4 ),
 ( 1.047024443964650053E-05, 0.008642110246132650442, 0.01810021157327289937 ),
 .UNSPECIFIED. ) ;
#29367=EDGE_CURVE ( 'NONE', #79206, #2874, #83018, .T. ) ;
#29369=VECTOR ( 'NONE', #63875, 1000.000000000000000 ) ;
#29373=ORIENTED_EDGE ( 'NONE', *, *, #79349, .F. ) ;
#29381=DIRECTION ( 'NONE',  ( -5.773159642023980606E-15, -5.773159642023980170E-30, -1.000000000000000000 ) ) ;
#29407=EDGE_LOOP ( 'NONE', ( #64057, #60635, #73709, #69561, #66421, #39769 ) ) ;
#29422=DIRECTION ( 'NONE',  ( -1.000000000000000000, -3.555032108465730541E-16, 0.000000000000000000 ) ) ;
#29439=DIRECTION ( 'NONE',  ( -3.100000000000000258E-29, 3.100000000000000044E-14, 1.000000000000000000 ) ) ;
#29449=EDGE_CURVE ( 'NONE', #68825, #60182, #81650, .T. ) ;
#29453=VECTOR ( 'NONE', #29204, 999.9999999999998863 ) ;
#29454=AXIS2_PLACEMENT_3D ( 'NONE', #33762, #7400, #83712 ) ;
#29456=ORIENTED_EDGE ( 'NONE', *, *, #82399, .F. ) ;
#29468=VERTEX_POINT ( 'NONE', #61615 ) ;
#29473=VECTOR ( 'NONE', #76818, 1000.000000000000000 ) ;
#29481=DIRECTION ( 'NONE',  ( -0.7071067811865473507, -0.7071067811865477948, 0.000000000000000000 ) ) ;
#29501=CARTESIAN_POINT ( 'NONE',  ( 92.81932083335593120, -113.5527167097541934, -11.78219314458173272 ) ) ;
#29507=CARTESIAN_POINT ( 'NONE',  ( 68.91678303834669350, -69.56165394957326953, 247.5002289977139753 ) ) ;
#29525=CARTESIAN_POINT ( 'NONE',  ( 143.1700167138480708, -139.0938916433959207, 247.5000110694289788 ) ) ;
#29557=VERTEX_POINT ( 'NONE', #75268 ) ;
#29560=EDGE_CURVE ( 'NONE', #24085, #85724, #87150, .T. ) ;
#29578=FACE_BOUND ( 'NONE', #26985, .T. ) ;
#29580=CARTESIAN_POINT ( 'NONE',  ( 124.6905118036815310, -83.08196156581362857, 250.2178068554180470 ) ) ;
#29582=EDGE_CURVE ( 'NONE', #42178, #4517, #76171, .T. ) ;
#29609=CARTESIAN_POINT ( 'NONE',  ( 145.2166182285888851, -69.56242951228074389, 247.5001056298889921 ) ) ;
#29612=EDGE_LOOP ( 'NONE', ( #36216, #7512, #83812, #335 ) ) ;
#29641=EDGE_LOOP ( 'NONE', ( #68639, #48409 ) ) ;
#29645=CARTESIAN_POINT ( 'NONE',  ( 70.27560645192561140, -140.3532164138353551, 246.6574697873465993 ) ) ;
#29669=DIRECTION ( 'NONE',  ( 1.000000000000000000, 0.000000000000000000, 0.000000000000000000 ) ) ;
#29673=DIRECTION ( 'NONE',  ( 3.100000000000000258E-29, -3.100000000000000044E-14, -1.000000000000000000 ) ) ;
#29685=LINE ( 'NONE', #10136, #21424 ) ;
#29691=EDGE_CURVE ( 'NONE', #3973, #68199, #10309, .T. ) ;
#29696=ORIENTED_EDGE ( 'NONE', *, *, #3850, .T. ) ;
#29707=EDGE_CURVE ( 'NONE', #23818, #77101, #35002, .T. ) ;
#29719=CARTESIAN_POINT ( 'NONE',  ( 145.6103092929421337, -69.25820179750351713, 247.4237039382404930 ) ) ;
#29726=PLANE ( 'NONE',  #34924 ) ;
#29732=ORIENTED_EDGE ( 'NONE', *, *, #46010, .T. ) ;
#29755=AXIS2_PLACEMENT_3D ( 'NONE', #55988, #71006, #21053 ) ;
#29802=EDGE_CURVE ( 'NONE', #8874, #5965, #57514, .T. ) ;
#29806=VECTOR ( 'NONE', #68656, 999.9999999999998863 ) ;
#29814=EDGE_CURVE ( 'NONE', #53126, #33347, #2119, .T. ) ;
#29827=EDGE_CURVE ( 'NONE', #27673, #74190, #78546, .T. ) ;
#29832=ADVANCED_FACE ( 'NONE', ( #12953 ), #52450, .F. ) ;
#29835=CARTESIAN_POINT ( 'NONE',  ( 79.56670390244703128, -105.9704134719596738, 250.2178068554180470 ) ) ;
#29837=ADVANCED_FACE ( 'NONE', ( #33381 ), #18402, .F. ) ;
#29857=AXIS2_PLACEMENT_3D ( 'NONE', #13951, #41635, #62545 ) ;
#29869=ORIENTED_EDGE ( 'NONE', *, *, #51162, .F. ) ;
#29892=DIRECTION ( 'NONE',  ( 0.000000000000000000, 0.000000000000000000, -1.000000000000000000 ) ) ;
#29894=ORIENTED_EDGE ( 'NONE', *, *, #54065, .F. ) ;
#29895=CARTESIAN_POINT ( 'NONE',  ( 74.06670390244701707, -90.27844715994098124, 222.2178068554179902 ) ) ;
#29907=EDGE_CURVE ( 'NONE', #76165, #58962, #81116, .T. ) ;
#29910=ORIENTED_EDGE ( 'NONE', *, *, #52240, .F. ) ;
#29924=VERTEX_POINT ( 'NONE', #27459 ) ;
#29928=CARTESIAN_POINT ( 'NONE',  ( 140.0667039024470455, -118.2784471599408960, 51.21780685541800437 ) ) ;
#29932=EDGE_CURVE ( 'NONE', #26236, #43244, #41083, .T. ) ;
#29938=CARTESIAN_POINT ( 'NONE',  ( 74.06670390244701707, -90.27844715994098124, 222.2178068554179902 ) ) ;
#29957=CARTESIAN_POINT ( 'NONE',  ( 140.0667039024470455, -118.2784471599408960, 222.2178068554179902 ) ) ;
#29972=CARTESIAN_POINT ( 'NONE',  ( 144.0315611170736645, -140.7135899453143111, 245.8512780488640033 ) ) ;
#30010=VECTOR ( 'NONE', #27073, 1000.000000000000000 ) ;
#30020=EDGE_CURVE ( 'NONE', #22233, #58142, #40931, .T. ) ;
#30059=CARTESIAN_POINT ( 'NONE',  ( 107.0667039024470313, -104.2784471599409528, 55.21780685541800437 ) ) ;
#30086=VERTEX_POINT ( 'NONE', #54692 ) ;
#30106=VECTOR ( 'NONE', #41537, 1000.000000000000000 ) ;
#30132=EDGE_CURVE ( 'NONE', #58881, #78082, #87218, .T. ) ;
#30139=EDGE_CURVE ( 'NONE', #59400, #71967, #84244, .T. ) ;
#30141=CARTESIAN_POINT ( 'NONE',  ( 107.9678037105606307, -121.2545485715093463, -19.18411693322849487 ) ) ;
#30161=CARTESIAN_POINT ( 'NONE',  ( 120.9654100508053176, -79.85256584427183668, 250.2201230397200220 ) ) ;
#30162=CARTESIAN_POINT ( 'NONE',  ( 146.8142838399337791, -68.11919575773853808, 246.4623081562874347 ) ) ;
#30178=ORIENTED_EDGE ( 'NONE', *, *, #67509, .F. ) ;
#30179=ORIENTED_EDGE ( 'NONE', *, *, #47951, .F. ) ;
#30184=FACE_OUTER_BOUND ( 'NONE', #52753, .T. ) ;
#30204=CYLINDRICAL_SURFACE ( 'NONE', #22611, 11.49999999999999645 ) ;
#30207=ADVANCED_FACE ( 'NONE', ( #10155 ), #79216, .F. ) ;
#30215=ORIENTED_EDGE ( 'NONE', *, *, #41968, .F. ) ;
#30252=CARTESIAN_POINT ( 'NONE',  ( 147.0667039024470739, -140.6784471599409017, 247.2178068554179902 ) ) ;
#30253=ORIENTED_EDGE ( 'NONE', *, *, #44334, .F. ) ;
#30265=ORIENTED_EDGE ( 'NONE', *, *, #29691, .T. ) ;
#30281=DIRECTION ( 'NONE',  ( 0.000000000000000000, 0.000000000000000000, -1.000000000000000000 ) ) ;
#30286=VERTEX_POINT ( 'NONE', #22453 ) ;
#30294=ORIENTED_EDGE ( 'NONE', *, *, #85795, .T. ) ;
#30299=EDGE_CURVE ( 'NONE', #49377, #53126, #75839, .T. ) ;
#30301=VECTOR ( 'NONE', #50833, 1000.000000000000000 ) ;
#30302=EDGE_CURVE ( 'NONE', #60027, #41538, #87353, .T. ) ;
#30321=ADVANCED_FACE ( 'NONE', ( #52338 ), #81003, .F. ) ;
#30327=LINE ( 'NONE', #42577, #34725 ) ;
#30340=DIRECTION ( 'NONE',  ( -1.000000000000000000, 0.000000000000000000, 0.000000000000000000 ) ) ;
#30349=ADVANCED_FACE ( 'NONE', ( #74166 ), #65993, .F. ) ;
#30354=VERTEX_POINT ( 'NONE', #45531 ) ;
#30357=CARTESIAN_POINT ( 'NONE',  ( 107.0667039024470313, -104.2784471599420897, -20.48315503890502143 ) ) ;
#30363=EDGE_CURVE ( 'NONE', #88034, #34414, #10591, .T. ) ;
#30368=VECTOR ( 'NONE', #20758, 1000.000000000000000 ) ;
#30373=CARTESIAN_POINT ( 'NONE',  ( 147.0667039024470171, -104.2784471599409102, 234.7178068554179902 ) ) ;
#30393=CARTESIAN_POINT ( 'NONE',  ( 107.5667039024470171, -94.77844715994137914, 2.217806855417697953 ) ) ;
#30397=CARTESIAN_POINT ( 'NONE',  ( 117.0667039024470313, -98.59953881414062948, 19.21780685541782319 ) ) ;
#30398=VECTOR ( 'NONE', #4684, 1000.000000000000000 ) ;
#30464=FACE_OUTER_BOUND ( 'NONE', #39997, .T. ) ;
#30466=CARTESIAN_POINT ( 'NONE',  ( 67.06670390244707392, -137.6784471599409869, 245.4361138696909848 ) ) ;
#30485=ORIENTED_EDGE ( 'NONE', *, *, #27404, .T. ) ;
#30502=DIRECTION ( 'NONE',  ( 1.000000000000000078E-15, -1.000000000000000000, 0.000000000000000000 ) ) ;
#30521=CYLINDRICAL_SURFACE ( 'NONE', #67310, 3.000000864267343026 ) ;
#30533=DIRECTION ( 'NONE',  ( 3.100000000000000258E-29, -3.100000000000000044E-14, -1.000000000000000000 ) ) ;
#30546=CARTESIAN_POINT ( 'NONE',  ( 102.7778427608900955, -89.25462229453661678, -11.78219314458248057 ) ) ;
#30547=CIRCLE ( 'NONE', #52231, 3.999999999999992895 ) ;
#30601=CARTESIAN_POINT ( 'NONE',  ( 145.2166182285888851, -69.56242951228074389, 247.5001056298889921 ) ) ;
#30610=CARTESIAN_POINT ( 'NONE',  ( 146.6569661690436703, -68.27214332003397601, 246.7106591300727416 ) ) ;
#30618=EDGE_LOOP ( 'NONE', ( #85726, #46992 ) ) ;
#30627=VECTOR ( 'NONE', #53515, 1000.000000000000000 ) ;
#30629=LINE ( 'NONE', #58327, #78304 ) ;
#30634=ORIENTED_EDGE ( 'NONE', *, *, #82134, .F. ) ;
#30653=AXIS2_PLACEMENT_3D ( 'NONE', #23067, #70293, #63474 ) ;
#30658=DIRECTION ( 'NONE',  ( 3.100000000000000258E-29, -3.100000000000000044E-14, -1.000000000000000000 ) ) ;
#30666=CARTESIAN_POINT ( 'NONE',  ( 67.23038816984393407, -137.5598464125348244, 246.3084021292352759 ) ) ;
#30686=ORIENTED_EDGE ( 'NONE', *, *, #19629, .T. ) ;
#30692=CARTESIAN_POINT ( 'NONE',  ( 147.0667039024470171, -79.67844715994090166, 55.21780685541800437 ) ) ;
#30717=CARTESIAN_POINT ( 'NONE',  ( 86.72755763596096301, -122.7870702624433648, 250.2178068554179902 ) ) ;
#30725=DIRECTION ( 'NONE',  ( 0.000000000000000000, 0.000000000000000000, 1.000000000000000000 ) ) ;
#30727=ORIENTED_EDGE ( 'NONE', *, *, #50358, .F. ) ;
#30739=CIRCLE ( 'NONE', #16231, 17.00000000000000000 ) ;
#30785=CARTESIAN_POINT ( 'NONE',  ( 91.91125933621933086, -96.68314769832139177, -21.78219314458224076 ) ) ;
#30789=EDGE_CURVE ( 'NONE', #61847, #80812, #89374, .T. ) ;
#30800=CARTESIAN_POINT ( 'NONE',  ( 146.0667039024470455, -121.7784471599409102, 55.21780685541800437 ) ) ;
#30806=ADVANCED_FACE ( 'NONE', ( #39416 ), #61200, .F. ) ;
#30842=CARTESIAN_POINT ( 'NONE',  ( 143.2570480158645978, -67.87844715994090450, 245.5376130668579719 ) ) ;
#30858=CARTESIAN_POINT ( 'NONE',  ( 144.5707550238523709, -140.1743960385356047, 245.5280425831230104 ) ) ;
#30871=DIRECTION ( 'NONE',  ( 1.000000000000000078E-15, -1.000000000000000000, 0.000000000000000000 ) ) ;
#30887=CARTESIAN_POINT ( 'NONE',  ( 102.7778427608900955, -89.25462229453692942, -21.78219314458248945 ) ) ;
#30891=DIRECTION ( 'NONE',  ( 0.000000000000000000, 0.000000000000000000, 1.000000000000000000 ) ) ;
#30905=CARTESIAN_POINT ( 'NONE',  ( 91.91125933621954402, -111.9799080603168449, -11.78219314458175937 ) ) ;
#30907=VECTOR ( 'NONE', #6132, 1000.000000000000000 ) ;
#30919=LINE ( 'NONE', #64556, #48558 ) ;
#30922=DIRECTION ( 'NONE',  ( -3.100000000000000258E-29, 3.100000000000000044E-14, 1.000000000000000000 ) ) ;
#30937=FACE_OUTER_BOUND ( 'NONE', #45831, .T. ) ;
#30942=ORIENTED_EDGE ( 'NONE', *, *, #73254, .T. ) ;
#30952=DIRECTION ( 'NONE',  ( 1.000000000000000000, 0.000000000000000000, 0.000000000000000000 ) ) ;
#30959=FACE_OUTER_BOUND ( 'NONE', #54343, .T. ) ;
#30963=EDGE_LOOP ( 'NONE', ( #75949, #45413, #78162, #11293 ) ) ;
#30968=AXIS2_PLACEMENT_3D ( 'NONE', #80342, #65360, #44452 ) ;
#30979=EDGE_CURVE ( 'NONE', #47447, #74740, #83391, .T. ) ;
#31023=CARTESIAN_POINT ( 'NONE',  ( 107.0667039024470313, -104.2784471599409102, 17.71780685541799016 ) ) ;
#31024=CARTESIAN_POINT ( 'NONE',  ( 144.5667039024470455, -118.2784471599408960, 45.21780685541799727 ) ) ;
#31025=CARTESIAN_POINT ( 'NONE',  ( 145.8907002709979963, -138.8544507913900077, 245.5998607319569942 ) ) ;
#31036=DIRECTION ( 'NONE',  ( 1.000000000000000000, 0.000000000000000000, 0.000000000000000000 ) ) ;
#31046=CARTESIAN_POINT ( 'NONE',  ( 76.05567402747949757, -69.25962940816080504, 247.5000682988239760 ) ) ;
#31051=VECTOR ( 'NONE', #36005, 1000.000000000000000 ) ;
#31059=LINE ( 'NONE', #85165, #10672 ) ;
#31061=CARTESIAN_POINT ( 'NONE',  ( 115.0988951105837259, -108.3384846469520113, 2.217806855418142042 ) ) ;
#31074=CARTESIAN_POINT ( 'NONE',  ( 97.81670390244700286, -67.87844715994096134, 55.21780685541800437 ) ) ;
#31080=DIRECTION ( 'NONE',  ( -0.7759704746411383303, 0.6307692307692303046, 0.000000000000000000 ) ) ;
#31082=CARTESIAN_POINT ( 'NONE',  ( 158.0667039024469886, -67.87844715994090450, 190.2178068554179902 ) ) ;
#31086=EDGE_CURVE ( 'NONE', #21942, #41501, #78447, .T. ) ;
#31093=CARTESIAN_POINT ( 'NONE',  ( 143.8252070173663810, -140.2851082128090070, 246.7259429745822388 ) ) ;
#31095=CYLINDRICAL_SURFACE ( 'NONE', #65890, 4.500000000000003553 ) ;
#31100=CARTESIAN_POINT ( 'NONE',  ( 67.71624685027074975, -137.3191804951919437, 246.9862057923735392 ) ) ;
#31111=CARTESIAN_POINT ( 'NONE',  ( 67.06670390244701707, -83.77844715994098124, 45.21780685541799727 ) ) ;
#31113=LINE ( 'NONE', #86554, #27660 ) ;
#31127=DIRECTION ( 'NONE',  ( -0.7071067811865470176, 2.110218113313392652E-14, 0.7071067811865480168 ) ) ;
#31133=ORIENTED_EDGE ( 'NONE', *, *, #76473, .T. ) ;
#31141=CARTESIAN_POINT ( 'NONE',  ( 91.91125933621933086, -100.4807974291317691, -21.78219314458213063 ) ) ;
#31152=PLANE ( 'NONE',  #67650 ) ;
#31200=DIRECTION ( 'NONE',  ( 3.100000000000000258E-29, -3.100000000000000044E-14, -1.000000000000000000 ) ) ;
#31207=CARTESIAN_POINT ( 'NONE',  ( 146.0667039024470455, -121.7784471599409102, 45.21780685541799727 ) ) ;
#31240=VECTOR ( 'NONE', #19711, 1000.000000000000000 ) ;
#31258=AXIS2_PLACEMENT_3D ( 'NONE', #4455, #46658, #52998 ) ;
#31269=VECTOR ( 'NONE', #22440, 1000.000000000000000 ) ;
#31274=CARTESIAN_POINT ( 'NONE',  ( 112.7841083645756015, -67.87923500319460857, 246.2950307662580087 ) ) ;
#31280=ORIENTED_EDGE ( 'NONE', *, *, #44463, .T. ) ;
#31285=EDGE_CURVE ( 'NONE', #77101, #24431, #7593, .T. ) ;
#31289=CARTESIAN_POINT ( 'NONE',  ( 89.92341143738899234, -67.87844715994096134, 245.7176246693439907 ) ) ;
#31292=VERTEX_POINT ( 'NONE', #5704 ) ;
#31301=DIRECTION ( 'NONE',  ( 0.7967329428042202455, -0.6043315462976655006, 1.875669758399919831E-14 ) ) ;
#31318=EDGE_CURVE ( 'NONE', #11860, #3381, #1121, .T. ) ;
#31325=EDGE_CURVE ( 'NONE', #45648, #20355, #70612, .T. ) ;
#31353=CARTESIAN_POINT ( 'NONE',  ( 67.06670390244701707, -81.17316614790567542, 245.5580738794290028 ) ) ;
#31372=DIRECTION ( 'NONE',  ( -1.000000000000000000, 0.000000000000000000, 0.000000000000000000 ) ) ;
#31404=VERTEX_POINT ( 'NONE', #20671 ) ;
#31423=EDGE_CURVE ( 'NONE', #11403, #19525, #7040, .T. ) ;
#31446=CIRCLE ( 'NONE', #82254, 4.500000000000003553 ) ;
#31450=ORIENTED_EDGE ( 'NONE', *, *, #10017, .T. ) ;
#31453=VERTEX_POINT ( 'NONE', #59189 ) ;
#31463=EDGE_CURVE ( 'NONE', #16883, #26687, #8846, .T. ) ;
#31481=CARTESIAN_POINT ( 'NONE',  ( 141.6666952063141878, -69.41153784729984011, 247.5000682988239760 ) ) ;
#31501=CIRCLE ( 'NONE', #82314, 7.999999999999992895 ) ;
#31504=DIRECTION ( 'NONE',  ( 3.100000000000000258E-29, -3.100000000000000044E-14, -1.000000000000000000 ) ) ;
#31505=EDGE_LOOP ( 'NONE', ( #81294, #43020, #34556 ) ) ;
#31514=EDGE_CURVE ( 'NONE', #9965, #39484, #32268, .T. ) ;
#31529=CIRCLE ( 'NONE', #21373, 7.999999999999992895 ) ;
#31539=DIRECTION ( 'NONE',  ( 0.000000000000000000, 0.000000000000000000, -1.000000000000000000 ) ) ;
#31560=DIRECTION ( 'NONE',  ( 0.000000000000000000, 0.000000000000000000, 1.000000000000000000 ) ) ;
#31568=VERTEX_POINT ( 'NONE', #32834 ) ;
#31577=ORIENTED_EDGE ( 'NONE', *, *, #18536, .F. ) ;
#31580=VECTOR ( 'NONE', #89691, 1000.000000000000000 ) ;
#31598=AXIS2_PLACEMENT_3D ( 'NONE', #66384, #86854, #24617 ) ;
#31599=CARTESIAN_POINT ( 'NONE',  ( 80.34435516212749917, -97.56809487397644887, 250.2178068554179902 ) ) ;
#31602=EDGE_CURVE ( 'NONE', #15550, #55635, #81905, .T. ) ;
#31606=CARTESIAN_POINT ( 'NONE',  ( 93.91125933621933086, -96.68314769832137756, -21.78219314458224076 ) ) ;
#31627=CARTESIAN_POINT ( 'NONE',  ( 90.06670390244701707, -101.5893827172046002, -9.937637710810113489 ) ) ;
#31635=EDGE_CURVE ( 'NONE', #24467, #54402, #85990, .T. ) ;
#31642=VECTOR ( 'NONE', #10342, 999.9999999999998863 ) ;
#31644=( BOUNDED_CURVE ( )  B_SPLINE_CURVE ( 2, ( #55294, #48038, #13987 ),
 .UNSPECIFIED., .F., .T. ) 
 B_SPLINE_CURVE_WITH_KNOTS ( ( 3, 3 ),
 ( 0.000000000000000000, 0.5053286420056770645 ),
 .UNSPECIFIED. ) 
 CURVE ( )  GEOMETRIC_REPRESENTATION_ITEM ( )  RATIONAL_B_SPLINE_CURVE ( ( 1.000000000000000000, 1.009299002520649857, 1.000420656333769864 ) ) 
 REPRESENTATION_ITEM ( '' )  );
#31657=CARTESIAN_POINT ( 'NONE',  ( 147.0667039024469886, -67.87844715994090450, 222.2178068554179902 ) ) ;
#31672=PLANE ( 'NONE',  #28279 ) ;
#31674=ORIENTED_EDGE ( 'NONE', *, *, #4765, .T. ) ;
#31676=ORIENTED_EDGE ( 'NONE', *, *, #29189, .T. ) ;
#31683=CARTESIAN_POINT ( 'NONE',  ( 122.2221484686747459, -111.8737466215628018, -19.26696060647578435 ) ) ;
#31701=VECTOR ( 'NONE', #26186, 1000.000000000000000 ) ;
#31725=AXIS2_PLACEMENT_3D ( 'NONE', #23538, #84425, #76696 ) ;
#31742=EDGE_CURVE ( 'NONE', #60190, #77633, #9636, .T. ) ;
#31748=AXIS2_PLACEMENT_3D ( 'NONE', #62304, #54566, #84117 ) ;
#31750=CARTESIAN_POINT ( 'NONE',  ( 99.48898161933318818, -91.15344715994181968, -11.78219314458242550 ) ) ;
#31763=EDGE_CURVE ( 'NONE', #86337, #57531, #32375, .T. ) ;
#31774=CARTESIAN_POINT ( 'NONE',  ( 144.0667052733537901, -71.37844715994090450, 55.21780685541800437 ) ) ;
#31791=AXIS2_PLACEMENT_3D ( 'NONE', #44614, #64630, #85548 ) ;
#31806=ORIENTED_EDGE ( 'NONE', *, *, #63985, .F. ) ;
#31807=DIRECTION ( 'NONE',  ( -4.440892098500939734E-16, 3.100000000000000044E-14, 1.000000000000000000 ) ) ;
#31823=ORIENTED_EDGE ( 'NONE', *, *, #83989, .F. ) ;
#31826=EDGE_CURVE ( 'NONE', #638, #36009, #49583, .T. ) ;
#31827=FACE_BOUND ( 'NONE', #16247, .T. ) ;
#31834=AXIS2_PLACEMENT_3D ( 'NONE', #85164, #17441, #45122 ) ;
#31837=CARTESIAN_POINT ( 'NONE',  ( 71.06670390244705970, -124.7784471599409812, 55.21780685541800437 ) ) ;
#31841=EDGE_LOOP ( 'NONE', ( #73803, #37420, #18216, #77059 ) ) ;
#31842=VECTOR ( 'NONE', #2267, 1000.000000000000000 ) ;
#31860=LINE ( 'NONE', #87727, #42836 ) ;
#31885=FACE_OUTER_BOUND ( 'NONE', #21722, .T. ) ;
#31911=FACE_OUTER_BOUND ( 'NONE', #22962, .T. ) ;
#31932=VERTEX_POINT ( 'NONE', #34626 ) ;
#31936=CARTESIAN_POINT ( 'NONE',  ( 146.0886660495907279, -68.82006323756704091, 247.2209606857130950 ) ) ;
#31994=CARTESIAN_POINT ( 'NONE',  ( 107.0667039024470313, -104.2784471599408676, 19.21780685541799016 ) ) ;
#32002=DIRECTION ( 'NONE',  ( 0.000000000000000000, 0.000000000000000000, -1.000000000000000000 ) ) ;
#32005=LINE ( 'NONE', #58809, #52163 ) ;
#32006=FACE_OUTER_BOUND ( 'NONE', #77663, .T. ) ;
#32031=EDGE_CURVE ( 'NONE', #38678, #28371, #63685, .T. ) ;
#32048=EDGE_CURVE ( 'NONE', #64360, #34428, #32191, .T. ) ;
#32056=ORIENTED_EDGE ( 'NONE', *, *, #34586, .F. ) ;
#32069=ORIENTED_EDGE ( 'NONE', *, *, #29827, .T. ) ;
#32081=ORIENTED_EDGE ( 'NONE', *, *, #48243, .T. ) ;
#32086=AXIS2_PLACEMENT_3D ( 'NONE', #74796, #39805, #60701 ) ;
#32103=CIRCLE ( 'NONE', #66927, 3.499999999999996003 ) ;
#32107=ORIENTED_EDGE ( 'NONE', *, *, #80428, .F. ) ;
#32113=CARTESIAN_POINT ( 'NONE',  ( 91.91441891875204817, -111.9861225405540637, -19.18411693322877198 ) ) ;
#32123=CARTESIAN_POINT ( 'NONE',  ( 117.0667039024470455, -109.9573555057411056, 17.71780685541815714 ) ) ;
#32124=CARTESIAN_POINT ( 'NONE',  ( 112.3521622943470675, -140.6784471636648561, 245.8674567499459727 ) ) ;
#32127=CARTESIAN_POINT ( 'NONE',  ( 69.56265278104177696, -140.1743960385357752, 245.5280425831230104 ) ) ;
#32146=ADVANCED_FACE ( 'NONE', ( #45441 ), #80448, .F. ) ;
#32182=CARTESIAN_POINT ( 'NONE',  ( 107.0667039024470313, -104.2784471599420755, -19.78219314458201694 ) ) ;
#32183=VERTEX_POINT ( 'NONE', #4130 ) ;
#32191=B_SPLINE_CURVE_WITH_KNOTS ( 'NONE', 3,
 ( #72294, #65468, #43673, #51370, #10063, #77766, #29609 ),
 .UNSPECIFIED., .F., .F.,
 ( 4, 1, 1, 1, 4 ),
 ( 0.000000000000000000, 0.2752441480442837096, 0.5749187429555715489, 0.8745933378668595548, 1.000000000000000000 ),
 .UNSPECIFIED. ) ;
#32210=VECTOR ( 'NONE', #16647, 1000.000000000000000 ) ;
#32246=CARTESIAN_POINT ( 'NONE',  ( 99.90204555947735798, -100.7192800061664713, -19.78219314458212708 ) ) ;
#32268=CIRCLE ( 'NONE', #80152, 7.999999999999992895 ) ;
#32269=LINE ( 'NONE', #12292, #18419 ) ;
#32270=DIRECTION ( 'NONE',  ( 0.000000000000000000, 0.000000000000000000, -1.000000000000000000 ) ) ;
#32281=VECTOR ( 'NONE', #604, 1000.000000000000114 ) ;
#32294=DIRECTION ( 'NONE',  ( -0.000000000000000000, -0.000000000000000000, -1.000000000000000000 ) ) ;
#32303=CARTESIAN_POINT ( 'NONE',  ( 75.29769027782792534, -100.6205720721962820, 249.3055308415380011 ) ) ;
#32304=ORIENTED_EDGE ( 'NONE', *, *, #7998, .F. ) ;
#32307=EDGE_LOOP ( 'NONE', ( #50959, #16275, #7384 ) ) ;
#32310=CARTESIAN_POINT ( 'NONE',  ( 107.0667039024470313, -104.2784471599420755, -19.78219314458201694 ) ) ;
#32311=CARTESIAN_POINT ( 'NONE',  ( 93.16752758198826712, -128.7026216972209625, 250.2203867545810283 ) ) ;
#32326=CARTESIAN_POINT ( 'NONE',  ( 54.06670390244700997, -79.67844715994098692, 55.21780685541800437 ) ) ;
#32346=DIRECTION ( 'NONE',  ( 0.000000000000000000, 0.000000000000000000, 1.000000000000000000 ) ) ;
#32347=EDGE_CURVE ( 'NONE', #56526, #85724, #40436, .T. ) ;
#32349=DIRECTION ( 'NONE',  ( 0.000000000000000000, 0.000000000000000000, -1.000000000000000000 ) ) ;
#32350=FACE_OUTER_BOUND ( 'NONE', #65754, .T. ) ;
#32375=LINE ( 'NONE', #11050, #20120 ) ;
#32379=CARTESIAN_POINT ( 'NONE',  ( 107.0667039024470313, -104.2784471599420755, -19.78219314458201694 ) ) ;
#32396=CARTESIAN_POINT ( 'NONE',  ( 99.53451269431033666, -99.35238426914629883, 2.217806855417836509 ) ) ;
#32407=DIRECTION ( 'NONE',  ( -1.000000000000000078E-15, 1.000000000000000000, 0.000000000000000000 ) ) ;
#32436=EDGE_CURVE ( 'NONE', #31292, #38678, #74625, .T. ) ;
#32445=DIRECTION ( 'NONE',  ( -3.100000000000000258E-29, 3.100000000000000044E-14, 1.000000000000000000 ) ) ;
#32448=DIRECTION ( 'NONE',  ( 1.000000000000000078E-15, -1.000000000000000000, 0.000000000000000000 ) ) ;
#32454=DIRECTION ( 'NONE',  ( 0.000000000000000000, 0.000000000000000000, -1.000000000000000000 ) ) ;
#32469=DIRECTION ( 'NONE',  ( 1.000000000000000000, 1.087812297297669405E-15, -2.722181216227750097E-30 ) ) ;
#32489=VECTOR ( 'NONE', #26431, 1000.000000000000000 ) ;
#32501=CARTESIAN_POINT ( 'NONE',  ( 104.0667030381796963, -67.87844715994094713, 93.21780742166239975 ) ) ;
#32504=ORIENTED_EDGE ( 'NONE', *, *, #29827, .F. ) ;
#32523=CIRCLE ( 'NONE', #44133, 3.499999999999996003 ) ;
#32555=CARTESIAN_POINT ( 'NONE',  ( 140.0667039024470171, -90.27844715994091018, 222.2178068554179902 ) ) ;
#32565=AXIS2_PLACEMENT_3D ( 'NONE', #20060, #60019, #32782 ) ;
#32571=CARTESIAN_POINT ( 'NONE',  ( 116.3167039024470029, -68.87844715994093292, 222.2178068554179902 ) ) ;
#32573=CARTESIAN_POINT ( 'NONE',  ( 127.0667052882549797, -71.37844715994091871, 55.21780685541800437 ) ) ;
#32574=CARTESIAN_POINT ( 'NONE',  ( 68.55293230179317732, -139.1646755592869908, 245.6810956053649875 ) ) ;
#32597=VECTOR ( 'NONE', #10332, 1000.000000000000000 ) ;
#32611=CARTESIAN_POINT ( 'NONE',  ( 147.0700838452252981, -67.87844715994090450, 246.0535151165250056 ) ) ;
#32620=AXIS2_PLACEMENT_3D ( 'NONE', #42174, #14041, #63076 ) ;
#32621=CIRCLE ( 'NONE', #86331, 27.49999999999999645 ) ;
#32622=VECTOR ( 'NONE', #8183, 1000.000000000000000 ) ;
#32623=ORIENTED_EDGE ( 'NONE', *, *, #10140, .T. ) ;
#32626=VECTOR ( 'NONE', #78881, 1000.000000000000000 ) ;
#32636=CARTESIAN_POINT ( 'NONE',  ( 74.06670390244704549, -118.2784471599409812, 51.21780685541800437 ) ) ;
#32654=VERTEX_POINT ( 'NONE', #47013 ) ;
#32655=CARTESIAN_POINT ( 'NONE',  ( 108.0667039024470455, -121.2010968907522113, -11.78219314458148226 ) ) ;
#32658=EDGE_CURVE ( 'NONE', #61103, #74274, #73845, .T. ) ;
#32672=ORIENTED_EDGE ( 'NONE', *, *, #70287, .F. ) ;
#32673=EDGE_CURVE ( 'NONE', #11503, #31292, #42009, .T. ) ;
#32685=CARTESIAN_POINT ( 'NONE',  ( 110.7536356736639078, -102.7271463785358492, -19.78219314458207378 ) ) ;
#32691=CIRCLE ( 'NONE', #39947, 11.49999999999999645 ) ;
#32704=ORIENTED_EDGE ( 'NONE', *, *, #36375, .T. ) ;
#32731=ORIENTED_EDGE ( 'NONE', *, *, #56380, .F. ) ;
#32741=DIRECTION ( 'NONE',  ( 3.100000000000000258E-29, -3.100000000000000044E-14, -1.000000000000000000 ) ) ;
#32757=DIRECTION ( 'NONE',  ( 1.000000000000000000, 1.000000000000000078E-15, 0.000000000000000000 ) ) ;
#32759=LINE ( 'NONE', #60454, #48931 ) ;
#32782=DIRECTION ( 'NONE',  ( -3.100000000000000258E-29, 3.100000000000000044E-14, 1.000000000000000000 ) ) ;
#32812=CIRCLE ( 'NONE', #64727, 121.3994834560769647 ) ;
#32826=B_SPLINE_SURFACE_WITH_KNOTS ( 'NONE', 3, 3, ( 
 ( #35042, #40520, #984, #55918 ),
 ( #76838, #61404, #69581, #6896 ),
 ( #35488, #41402, #83218, #7353 ),
 ( #75502, #62752, #70030, #63207 ),
 ( #55467, #20542, #21888, #82781 ) ),
 .UNSPECIFIED., .F., .F., .F.,
 ( 4, 1, 4 ),
 ( 4, 4 ),
 ( 0.000000000000000000, 0.5714285714285709528, 1.000000000000000000 ),
 ( -1.896658054595430056E-14, 0.2508910862621460125 ),
 .UNSPECIFIED. ) ;
#32834=CARTESIAN_POINT ( 'NONE',  ( 106.1656040943334318, -87.30234574837452044, -11.78219314458253741 ) ) ;
#32837=ORIENTED_EDGE ( 'NONE', *, *, #55698, .F. ) ;
#32849=CARTESIAN_POINT ( 'NONE',  ( 71.06670390244701707, -83.77844715994098124, 55.21780685541800437 ) ) ;
#32881=DIRECTION ( 'NONE',  ( 1.000000000000000000, 0.000000000000000000, 0.000000000000000000 ) ) ;
#32886=LINE ( 'NONE', #60585, #61447 ) ;
#32888=CARTESIAN_POINT ( 'NONE',  ( 115.5439452383991892, -99.96145986183427112, -19.78219314458215550 ) ) ;
#32891=CARTESIAN_POINT ( 'NONE',  ( 103.3797721312301547, -105.8297479413482876, -19.78219314458196010 ) ) ;
#32894=DIRECTION ( 'NONE',  ( 1.000000000000000000, 1.000000000000000078E-15, 0.000000000000000000 ) ) ;
#32903=DIRECTION ( 'NONE',  ( -1.000000000000000000, 0.000000000000000000, 0.000000000000000000 ) ) ;
#32910=ORIENTED_EDGE ( 'NONE', *, *, #15660, .T. ) ;
#32913=FACE_OUTER_BOUND ( 'NONE', #38760, .T. ) ;
#32916=CARTESIAN_POINT ( 'NONE',  ( 107.9678037105606023, -87.30234574837452044, -11.78219314458253741 ) ) ;
#32926=DIRECTION ( 'NONE',  ( 1.000000000000000000, 1.000000000000000078E-15, 0.000000000000000000 ) ) ;
#32939=VECTOR ( 'NONE', #57250, 1000.000000000000000 ) ;
#32945=ORIENTED_EDGE ( 'NONE', *, *, #41855, .F. ) ;
#33014=DIRECTION ( 'NONE',  ( -0.000000000000000000, -0.000000000000000000, 1.000000000000000000 ) ) ;
#33016=AXIS2_PLACEMENT_3D ( 'NONE', #40391, #12704, #88117 ) ;
#33017=VECTOR ( 'NONE', #21085, 1000.000000000000000 ) ;
#33025=AXIS2_PLACEMENT_3D ( 'NONE', #41238, #35325, #20380 ) ;
#33026=CARTESIAN_POINT ( 'NONE',  ( 145.2153822645345826, -139.0823765015731794, 246.7463595109249184 ) ) ;
#33056=ADVANCED_FACE ( 'NONE', ( #24258 ), #64260, .T. ) ;
#33060=ORIENTED_EDGE ( 'NONE', *, *, #7369, .F. ) ;
#33070=CARTESIAN_POINT ( 'NONE',  ( 117.0667039024470313, -104.2784471599408960, 17.71780685541799016 ) ) ;
#33074=ORIENTED_EDGE ( 'NONE', *, *, #13978, .T. ) ;
#33077=ORIENTED_EDGE ( 'NONE', *, *, #83155, .F. ) ;
#33081=DIRECTION ( 'NONE',  ( -0.9999999999998281375, 0.000000000000000000, 5.861124988064729938E-07 ) ) ;
#33110=ORIENTED_EDGE ( 'NONE', *, *, #61350, .F. ) ;
#33125=CIRCLE ( 'NONE', #34544, 8.999999999999994671 ) ;
#33131=VERTEX_POINT ( 'NONE', #60539 ) ;
#33152=AXIS2_PLACEMENT_3D ( 'NONE', #88367, #89708, #27018 ) ;
#33155=DIRECTION ( 'NONE',  ( -3.100000000000000258E-29, 3.100000000000000044E-14, 1.000000000000000000 ) ) ;
#33156=AXIS2_PLACEMENT_3D ( 'NONE', #49068, #14585, #42261 ) ;
#33191=ORIENTED_EDGE ( 'NONE', *, *, #18536, .T. ) ;
#33242=CARTESIAN_POINT ( 'NONE',  ( 136.5167039024470341, -103.2284471599409272, 55.21780685541800437 ) ) ;
#33244=EDGE_CURVE ( 'NONE', #37103, #33131, #46004, .T. ) ;
#33252=CARTESIAN_POINT ( 'NONE',  ( 145.7718159158550293, -125.9396293856170956, 247.4783998280190076 ) ) ;
#33274=LINE ( 'NONE', #88259, #88452 ) ;
#33297=ORIENTED_EDGE ( 'NONE', *, *, #48557, .T. ) ;
#33305=CYLINDRICAL_SURFACE ( 'NONE', #62382, 3.500000000000003109 ) ;
#33311=VERTEX_POINT ( 'NONE', #35985 ) ;
#33347=VERTEX_POINT ( 'NONE', #34182 ) ;
#33365=ORIENTED_EDGE ( 'NONE', *, *, #82116, .F. ) ;
#33377=FACE_OUTER_BOUND ( 'NONE', #51754, .T. ) ;
#33381=FACE_OUTER_BOUND ( 'NONE', #83588, .T. ) ;
#33399=CARTESIAN_POINT ( 'NONE',  ( 144.0667052733537901, -75.82844715994092155, 222.2178068554179902 ) ) ;
#33408=ORIENTED_EDGE ( 'NONE', *, *, #9191, .T. ) ;
#33413=CARTESIAN_POINT ( 'NONE',  ( 107.0667039024470313, -104.2784471599420755, -19.78219314458201694 ) ) ;
#33435=ORIENTED_EDGE ( 'NONE', *, *, #45791, .F. ) ;
#33475=CARTESIAN_POINT ( 'NONE',  ( 145.4156254839468829, -139.2796780384615261, 246.0351580304962056 ) ) ;
#33477=CARTESIAN_POINT ( 'NONE',  ( 122.2211117073404409, -111.9484015127202667, -19.21046202161275218 ) ) ;
#33507=FACE_BOUND ( 'NONE', #86158, .T. ) ;
#33511=EDGE_CURVE ( 'NONE', #76783, #67053, #86825, .T. ) ;
#33513=ADVANCED_FACE ( 'NONE', ( #24156 ), #8010, .T. ) ;
#33521=DIRECTION ( 'NONE',  ( -3.100000000000000258E-29, 3.100000000000000044E-14, 1.000000000000000000 ) ) ;
#33524=CARTESIAN_POINT ( 'NONE',  ( 74.06670390244704549, -118.2784471599409812, 230.7030882296565721 ) ) ;
#33545=DIRECTION ( 'NONE',  ( -1.000000000000000000, -8.540177112501204385E-16, 0.000000000000000000 ) ) ;
#33562=ORIENTED_EDGE ( 'NONE', *, *, #53543, .T. ) ;
#33563=UNCERTAINTY_MEASURE_WITH_UNIT (LENGTH_MEASURE( 1.000000000000000082E-05 ), #70451, 'distance_accuracy_value', 'NONE');
#33623=EDGE_CURVE ( 'NONE', #13040, #28371, #53151, .T. ) ;
#33626=DIRECTION ( 'NONE',  ( 0.000000000000000000, 0.000000000000000000, 1.000000000000000000 ) ) ;
#33639=ORIENTED_EDGE ( 'NONE', *, *, #19453, .T. ) ;
#33640=ORIENTED_EDGE ( 'NONE', *, *, #50512, .T. ) ;
#33659=DIRECTION ( 'NONE',  ( 1.000000000000000078E-15, -1.000000000000000000, 0.000000000000000000 ) ) ;
#33661=CARTESIAN_POINT ( 'NONE',  ( 107.0667039024470313, -104.2784471599409528, 45.21780685541799727 ) ) ;
#33674=CARTESIAN_POINT ( 'NONE',  ( 145.2084014158841399, -138.9257025692045033, 247.5112265945679724 ) ) ;
#33682=DIRECTION ( 'NONE',  ( -1.000000000000000000, -1.541976423090496028E-15, 0.000000000000000000 ) ) ;
#33713=EDGE_CURVE ( 'NONE', #23612, #60182, #28160, .T. ) ;
#33725=CARTESIAN_POINT ( 'NONE',  ( 67.06670390244700286, -67.87844715994098976, 247.2178068554179902 ) ) ;
#33728=CARTESIAN_POINT ( 'NONE',  ( 107.0667039024470313, -104.2784471599409528, 19.21780685541800437 ) ) ;
#33729=CARTESIAN_POINT ( 'NONE',  ( 76.06670390244703128, -104.2784471599409812, 45.21780685541799727 ) ) ;
#33733=EDGE_LOOP ( 'NONE', ( #36295, #30634, #64589, #25035 ) ) ;
#33752=ORIENTED_EDGE ( 'NONE', *, *, #68372, .F. ) ;
#33754=CARTESIAN_POINT ( 'NONE',  ( 107.0667039024470313, -104.2784471599409528, 23.21780685541800082 ) ) ;
#33756=ORIENTED_EDGE ( 'NONE', *, *, #37285, .F. ) ;
#33761=ORIENTED_EDGE ( 'NONE', *, *, #21302, .T. ) ;
#33762=CARTESIAN_POINT ( 'NONE',  ( 140.0667039024470455, -118.2784471599408960, 222.2178068554179902 ) ) ;
#33796=PLANE ( 'NONE',  #17644 ) ;
#33807=CIRCLE ( 'NONE', #45395, 32.50000000000001421 ) ;
#33808=EDGE_LOOP ( 'NONE', ( #80748, #55777, #59944, #84979 ) ) ;
#33809=ORIENTED_EDGE ( 'NONE', *, *, #18736, .T. ) ;
#33837=VERTEX_POINT ( 'NONE', #27723 ) ;
#33848=EDGE_LOOP ( 'NONE', ( #58763, #14446, #5574, #78457 ) ) ;
#33849=ORIENTED_EDGE ( 'NONE', *, *, #33244, .T. ) ;
#33876=VERTEX_POINT ( 'NONE', #26818 ) ;
#33879=ORIENTED_EDGE ( 'NONE', *, *, #63660, .F. ) ;
#33881=DIRECTION ( 'NONE',  ( 1.000000000000000000, 1.000000000000000078E-15, 0.000000000000000000 ) ) ;
#33892=VERTEX_POINT ( 'NONE', #48142 ) ;
#33918=CARTESIAN_POINT ( 'NONE',  ( 93.91125933621934507, -111.8737466215625744, -11.78219314458178779 ) ) ;
#33920=LINE ( 'NONE', #32571, #71623 ) ;
#33921=CARTESIAN_POINT ( 'NONE',  ( 145.4224990655192187, -139.2862363000336074, 245.9798482249633764 ) ) ;
#33950=VERTEX_POINT ( 'NONE', #44019 ) ;
#33973=CARTESIAN_POINT ( 'NONE',  ( 107.0667039024470171, -89.08784823670032438, -11.78219314458248057 ) ) ;
#33975=LINE ( 'NONE', #48475, #85402 ) ;
#33987=FACE_OUTER_BOUND ( 'NONE', #16127, .T. ) ;
#34006=CARTESIAN_POINT ( 'NONE',  ( 107.0667039024469886, -70.87844715994094713, 133.2178068554180186 ) ) ;
#34007=ORIENTED_EDGE ( 'NONE', *, *, #74300, .T. ) ;
#34012=VERTEX_POINT ( 'NONE', #50393 ) ;
#34019=LINE ( 'NONE', #28553, #10917 ) ;
#34035=CARTESIAN_POINT ( 'NONE',  ( 107.0667039024470313, -104.2784471599420755, -19.78219314458201694 ) ) ;
#34043=LINE ( 'NONE', #42205, #67652 ) ;
#34061=VERTEX_POINT ( 'NONE', #29076 ) ;
#34077=CARTESIAN_POINT ( 'NONE',  ( 98.58946256649485917, -108.5954344580491835, 2.217806855418142042 ) ) ;
#34083=EDGE_LOOP ( 'NONE', ( #40417, #64828, #40779, #21568 ) ) ;
#34088=ORIENTED_EDGE ( 'NONE', *, *, #19731, .T. ) ;
#34106=CARTESIAN_POINT ( 'NONE',  ( 101.5797435165433598, -139.8917819456133600, 247.5112265945679724 ) ) ;
#34112=AXIS2_PLACEMENT_3D ( 'NONE', #85348, #65751, #3539 ) ;
#34121=EDGE_CURVE ( 'NONE', #31404, #14173, #34175, .T. ) ;
#34125=CARTESIAN_POINT ( 'NONE',  ( 115.0439452383992318, -109.4614598618335890, 2.217806855418169576 ) ) ;
#34130=CARTESIAN_POINT ( 'NONE',  ( 59.56670390244699576, -67.87844715994098976, 155.2178068554179902 ) ) ;
#34133=VECTOR ( 'NONE', #65540, 1000.000000000000000 ) ;
#34135=CARTESIAN_POINT ( 'NONE',  ( 129.9953678291896040, -88.62578511436512940, 250.2191008560389776 ) ) ;
#34175=CIRCLE ( 'NONE', #31258, 11.49999999999999645 ) ;
#34182=CARTESIAN_POINT ( 'NONE',  ( 114.5988951105837117, -99.35238426914628462, 2.217806855417836509 ) ) ;
#34189=ORIENTED_EDGE ( 'NONE', *, *, #8505, .F. ) ;
#34251=ORIENTED_EDGE ( 'NONE', *, *, #37377, .F. ) ;
#34260=CARTESIAN_POINT ( 'NONE',  ( 83.56670390244703128, -104.2784471599409670, 23.21780685541800082 ) ) ;
#34271=CARTESIAN_POINT ( 'NONE',  ( 122.2221484686747317, -96.68314769832130651, -19.26696060647622843 ) ) ;
#34282=CARTESIAN_POINT ( 'NONE',  ( 70.06670417066790435, -69.62844715994098976, 55.21780685541800437 ) ) ;
#34284=ADVANCED_FACE ( 'NONE', ( #20333 ), #83446, .F. ) ;
#34302=ORIENTED_EDGE ( 'NONE', *, *, #23475, .F. ) ;
#34309=ORIENTED_EDGE ( 'NONE', *, *, #53470, .T. ) ;
#34332=FACE_OUTER_BOUND ( 'NONE', #61108, .T. ) ;
#34359=ORIENTED_EDGE ( 'NONE', *, *, #84582, .T. ) ;
#34371=ORIENTED_EDGE ( 'NONE', *, *, #77603, .F. ) ;
#34374=AXIS2_PLACEMENT_3D ( 'NONE', #77367, #35572, #15147 ) ;
#34402=ADVANCED_FACE ( 'NONE', ( #55260 ), #62095, .F. ) ;
#34403=CARTESIAN_POINT ( 'NONE',  ( 145.3334424738984012, -69.47022780016817478, 247.4823562763598090 ) ) ;
#34414=VERTEX_POINT ( 'NONE', #45101 ) ;
#34428=VERTEX_POINT ( 'NONE', #30601 ) ;
#34444=ORIENTED_EDGE ( 'NONE', *, *, #24792, .T. ) ;
#34447=DIRECTION ( 'NONE',  ( 0.000000000000000000, 0.000000000000000000, -1.000000000000000000 ) ) ;
#34453=DIRECTION ( 'NONE',  ( -3.100000000000000258E-29, 3.100000000000000044E-14, 1.000000000000000000 ) ) ;
#34455=AXIS2_PLACEMENT_3D ( 'NONE', #74501, #81346, #12278 ) ;
#34466=ORIENTED_EDGE ( 'NONE', *, *, #13524, .T. ) ;
#34471=CARTESIAN_POINT ( 'NONE',  ( 103.3797721312301547, -105.8297479413482876, -19.78219314458196010 ) ) ;
#34531=CARTESIAN_POINT ( 'NONE',  ( 144.0667039024470171, -102.7784471599409102, 222.2178068554179902 ) ) ;
#34541=CIRCLE ( 'NONE', #76635, 2.000000000000001776 ) ;
#34544=AXIS2_PLACEMENT_3D ( 'NONE', #44759, #79313, #37520 ) ;
#34546=CARTESIAN_POINT ( 'NONE',  ( 118.2946795739112531, -90.36568251306729849, -9.274842254011062437 ) ) ;
#34556=ORIENTED_EDGE ( 'NONE', *, *, #29189, .F. ) ;
#34572=CARTESIAN_POINT ( 'NONE',  ( 68.76053423562146349, -136.8603496727827746, 247.4879725229279757 ) ) ;
#34578=FACE_OUTER_BOUND ( 'NONE', #71081, .T. ) ;
#34586=EDGE_CURVE ( 'NONE', #19483, #36508, #57462, .T. ) ;
#34587=CARTESIAN_POINT ( 'NONE',  ( 134.2858849160865589, -126.1915520417814207, 249.3055338466990065 ) ) ;
#34590=CIRCLE ( 'NONE', #27390, 2.999999999999988898 ) ;
#34604=ORIENTED_EDGE ( 'NONE', *, *, #63169, .T. ) ;
#34606=AXIS2_PLACEMENT_3D ( 'NONE', #38727, #81441, #4218 ) ;
#34621=VERTEX_POINT ( 'NONE', #87797 ) ;
#34626=CARTESIAN_POINT ( 'NONE',  ( 107.5667039024470171, -96.29408744860640468, -19.78219314458226563 ) ) ;
#34630=ORIENTED_EDGE ( 'NONE', *, *, #51344, .F. ) ;
#34635=VECTOR ( 'NONE', #89733, 1000.000000000000000 ) ;
#34640=ADVANCED_FACE ( 'NONE', ( #81455 ), #39632, .T. ) ;
#34648=ORIENTED_EDGE ( 'NONE', *, *, #46466, .T. ) ;
#34651=VERTEX_POINT ( 'NONE', #60517 ) ;
#34653=CARTESIAN_POINT ( 'NONE',  ( 106.5667039024470455, -112.2628068712777036, -19.78219314458176825 ) ) ;
#34680=ORIENTED_EDGE ( 'NONE', *, *, #40667, .F. ) ;
#34682=CARTESIAN_POINT ( 'NONE',  ( 154.5667039024469886, -67.87844715994090450, 190.2178068554179902 ) ) ;
#34707=CARTESIAN_POINT ( 'NONE',  ( 69.94614915224266838, -138.0587248278177697, 247.6570847665630026 ) ) ;
#34708=CARTESIAN_POINT ( 'NONE',  ( 160.0667039024470171, -79.67844715994088745, 222.2178068554179902 ) ) ;
#34721=CARTESIAN_POINT ( 'NONE',  ( 107.0667039024470313, -104.2784471599413791, 2.217806855418003043 ) ) ;
#34725=VECTOR ( 'NONE', #23084, 1000.000000000000000 ) ;
#34751=VECTOR ( 'NONE', #28196, 1000.000000000000000 ) ;
#34787=DIRECTION ( 'NONE',  ( 3.100000000000000258E-29, -3.100000000000000044E-14, -1.000000000000000000 ) ) ;
#34789=VERTEX_POINT ( 'NONE', #35054 ) ;
#34807=ORIENTED_EDGE ( 'NONE', *, *, #10807, .T. ) ;
#34814=ADVANCED_FACE ( 'NONE', ( #13730 ), #82795, .F. ) ;
#34819=CARTESIAN_POINT ( 'NONE',  ( 145.1716789765235660, -139.0389598750564915, 246.8368799019731910 ) ) ;
#34831=LINE ( 'NONE', #62538, #79653 ) ;
#34851=EDGE_LOOP ( 'NONE', ( #23922, #52667, #80532, #75552 ) ) ;
#34853=VERTEX_POINT ( 'NONE', #76404 ) ;
#34885=DIRECTION ( 'NONE',  ( -0.7071067811865487940, 0.7071067811865463515, 0.000000000000000000 ) ) ;
#34908=EDGE_CURVE ( 'NONE', #41047, #20369, #86359, .T. ) ;
#34911=AXIS2_PLACEMENT_3D ( 'NONE', #83583, #27260, #26367 ) ;
#34913=VECTOR ( 'NONE', #31560, 1000.000000000000000 ) ;
#34915=ORIENTED_EDGE ( 'NONE', *, *, #62805, .T. ) ;
#34924=AXIS2_PLACEMENT_3D ( 'NONE', #220, #69721, #42435 ) ;
#34936=AXIS2_PLACEMENT_3D ( 'NONE', #22207, #42611, #70343 ) ;
#34943=FACE_OUTER_BOUND ( 'NONE', #46993, .T. ) ;
#34956=DIRECTION ( 'NONE',  ( 1.000000000000000000, 0.000000000000000000, 0.000000000000000000 ) ) ;
#34967=ORIENTED_EDGE ( 'NONE', *, *, #74300, .F. ) ;
#34972=ORIENTED_EDGE ( 'NONE', *, *, #22576, .T. ) ;
#34983=CARTESIAN_POINT ( 'NONE',  ( 106.1656040943334602, -121.2545485715093463, -19.18411693322849487 ) ) ;
#34986=VERTEX_POINT ( 'NONE', #2348 ) ;
#34991=DIRECTION ( 'NONE',  ( -1.000000000000000000, -1.000000000000000078E-15, 0.000000000000000000 ) ) ;
#35002=CIRCLE ( 'NONE', #61071, 1.999999999999995781 ) ;
#35006=CARTESIAN_POINT ( 'NONE',  ( 88.18995264527245581, -124.3682898089926709, 250.2203867545810283 ) ) ;
#35016=EDGE_LOOP ( 'NONE', ( #14388, #87117, #73195, #40130, #3059 ) ) ;
#35035=VERTEX_POINT ( 'NONE', #57286 ) ;
#35041=DIRECTION ( 'NONE',  ( 3.100000000000000258E-29, -3.100000000000000044E-14, -1.000000000000000000 ) ) ;
#35042=CARTESIAN_POINT ( 'NONE',  ( 69.95929469538086209, -138.0461895383714932, 247.6591799766680140 ) ) ;
#35054=CARTESIAN_POINT ( 'NONE',  ( 67.06670390244700286, -67.87844716047356997, 245.4920193514540188 ) ) ;
#35055=DIRECTION ( 'NONE',  ( -1.000000000000000000, -8.540177112501204385E-16, 0.000000000000000000 ) ) ;
#35065=ADVANCED_FACE ( 'NONE', ( #15980 ), #71397, .T. ) ;
#35081=CARTESIAN_POINT ( 'NONE',  ( 61.06670390244706681, -137.6784471599409869, 55.21780685541800437 ) ) ;
#35108=ORIENTED_EDGE ( 'NONE', *, *, #40528, .F. ) ;
#35115=CARTESIAN_POINT ( 'NONE',  ( 68.69356659899807482, -139.3022005417465436, 245.7546487670440740 ) ) ;
#35125=CARTESIAN_POINT ( 'NONE',  ( 99.51799851144285469, -130.7908339518065191, 250.2178068554179902 ) ) ;
#35164=CARTESIAN_POINT ( 'NONE',  ( 67.75193203802449204, -68.53543518790235112, 247.0040750501697744 ) ) ;
#35190=CARTESIAN_POINT ( 'NONE',  ( 158.0667039024470171, -79.67844715994088745, 190.2178068554179902 ) ) ;
#35208=DIRECTION ( 'NONE',  ( -1.000000000000000000, -8.163404592832032979E-16, 0.000000000000000000 ) ) ;
#35214=EDGE_CURVE ( 'NONE', #73928, #88034, #34043, .T. ) ;
#35224=DIRECTION ( 'NONE',  ( -8.538276166416950255E-16, 1.000000000000000000, -3.100000000000000044E-14 ) ) ;
#35229=LINE ( 'NONE', #29335, #16187 ) ;
#35245=CARTESIAN_POINT ( 'NONE',  ( 107.0667039024470313, -104.2784471599418197, -11.78219314458200984 ) ) ;
#35248=DIRECTION ( 'NONE',  ( 1.157009245868378063E-15, -1.000000000000000000, 3.100000000000000044E-14 ) ) ;
#35250=VECTOR ( 'NONE', #38109, 1000.000000000000000 ) ;
#35252=VERTEX_POINT ( 'NONE', #55372 ) ;
#35264=ORIENTED_EDGE ( 'NONE', *, *, #80391, .F. ) ;
#35266=ORIENTED_EDGE ( 'NONE', *, *, #89164, .F. ) ;
#35284=AXIS2_PLACEMENT_3D ( 'NONE', #67873, #32002, #59696 ) ;
#35285=FACE_OUTER_BOUND ( 'NONE', #35807, .T. ) ;
#35288=ORIENTED_EDGE ( 'NONE', *, *, #44690, .F. ) ;
#35319=EDGE_CURVE ( 'NONE', #76564, #86303, #86244, .T. ) ;
#35325=DIRECTION ( 'NONE',  ( -0.000000000000000000, -0.000000000000000000, -1.000000000000000000 ) ) ;
#35347=CARTESIAN_POINT ( 'NONE',  ( 77.65064691800776586, -139.0649736490145187, 247.5503376965620532 ) ) ;
#35371=DIRECTION ( 'NONE',  ( -0.8660254037844382635, -0.5000000000000008882, 1.550000000000000022E-14 ) ) ;
#35380=ORIENTED_EDGE ( 'NONE', *, *, #17599, .F. ) ;
#35391=ORIENTED_EDGE ( 'NONE', *, *, #8903, .F. ) ;
#35393=LINE ( 'NONE', #68594, #62905 ) ;
#35400=CARTESIAN_POINT ( 'NONE',  ( 107.0667039024469886, -70.87844715994094713, 173.2178068554179902 ) ) ;
#35413=AXIS2_PLACEMENT_3D ( 'NONE', #66162, #46153, #45701 ) ;
#35414=ORIENTED_EDGE ( 'NONE', *, *, #24527, .F. ) ;
#35429=DIRECTION ( 'NONE',  ( 3.100000000000000258E-29, -3.100000000000000044E-14, -1.000000000000000000 ) ) ;
#35436=DIRECTION ( 'NONE',  ( -3.100000000000000258E-29, 3.100000000000000044E-14, 1.000000000000000000 ) ) ;
#35446=ORIENTED_EDGE ( 'NONE', *, *, #47258, .T. ) ;
#35451=CARTESIAN_POINT ( 'NONE',  ( 107.0667036193247696, -67.87844715994094713, 90.21780599115065513 ) ) ;
#35461=CARTESIAN_POINT ( 'NONE',  ( 107.0667039024470313, -104.2784471599409528, 19.21780685541800437 ) ) ;
#35466=DIRECTION ( 'NONE',  ( 0.000000000000000000, 0.000000000000000000, -1.000000000000000000 ) ) ;
#35471=CARTESIAN_POINT ( 'NONE',  ( 56.06670390244699576, -67.87844715994098976, 190.2178068554179902 ) ) ;
#35479=DIRECTION ( 'NONE',  ( -1.000000000000000000, -1.181088324069315053E-15, 0.000000000000000000 ) ) ;
#35488=CARTESIAN_POINT ( 'NONE',  ( 68.96011658976357239, -139.1256438676158780, 247.0684195519230002 ) ) ;
#35511=VECTOR ( 'NONE', #89681, 1000.000000000000000 ) ;
#35539=ORIENTED_EDGE ( 'NONE', *, *, #65176, .F. ) ;
#35541=VECTOR ( 'NONE', #75537, 1000.000000000000000 ) ;
#35545=AXIS2_PLACEMENT_3D ( 'NONE', #30785, #46627, #73007 ) ;
#35550=B_SPLINE_CURVE_WITH_KNOTS ( 'NONE', 3,
 ( #64308, #63861, #42938, #85216, #16160, #55653, #71576, #22091, #8447, #37039, #7550, #49756, #56111, #43839, #35688, #720, #281, #83404, #70672 ),
 .UNSPECIFIED., .F., .F.,
 ( 4, 2, 2, 2, 1, 1, 1, 2, 2, 2, 4 ),
 ( 0.000000000000000000, 0.2499999999998125944, 0.3749999999997070121, 0.4374999999996485589, 0.4687499999996253552, 0.4843749999996137534, 0.4921874999995934363, 0.4960937499995964339, 0.4999999999995994315, 0.7499999999997997158, 1.000000000000000000 ),
 .UNSPECIFIED. ) ;
#35556=VECTOR ( 'NONE', #22323, 1000.000000000000000 ) ;
#35565=VECTOR ( 'NONE', #11908, 1000.000000000000000 ) ;
#35572=DIRECTION ( 'NONE',  ( 1.000000000000000078E-15, -1.000000000000000000, 0.000000000000000000 ) ) ;
#35574=DIRECTION ( 'NONE',  ( 1.000000000000000000, 0.000000000000000000, 0.000000000000000000 ) ) ;
#35576=CARTESIAN_POINT ( 'NONE',  ( 92.53858863555701930, -127.7054288962555830, 250.2178068554179902 ) ) ;
#35596=CARTESIAN_POINT ( 'NONE',  ( 147.0667039024470171, -79.67844715994090166, 96.96780685541800437 ) ) ;
#35599=DIRECTION ( 'NONE',  ( 1.000000000000000078E-15, -1.000000000000000000, 0.000000000000000000 ) ) ;
#35605=ORIENTED_EDGE ( 'NONE', *, *, #622, .T. ) ;
#35606=EDGE_LOOP ( 'NONE', ( #44857, #54870, #58070, #61183 ) ) ;
#35618=DIRECTION ( 'NONE',  ( -3.100000000000000258E-29, 3.100000000000000044E-14, 1.000000000000000000 ) ) ;
#35620=CARTESIAN_POINT ( 'NONE',  ( 68.14696562930211599, -68.91192709141064654, 247.2707748063552344 ) ) ;
#35651=ORIENTED_EDGE ( 'NONE', *, *, #9500, .F. ) ;
#35688=CARTESIAN_POINT ( 'NONE',  ( 146.7350708469755602, -137.4719268671379098, 246.6379283462439673 ) ) ;
#35702=ORIENTED_EDGE ( 'NONE', *, *, #4254, .T. ) ;
#35705=EDGE_CURVE ( 'NONE', #80877, #8011, #50325, .T. ) ;
#35706=ORIENTED_EDGE ( 'NONE', *, *, #31826, .F. ) ;
#35719=EDGE_LOOP ( 'NONE', ( #30727, #55672, #47487, #43338 ) ) ;
#35721=DIRECTION ( 'NONE',  ( -1.000000000000000078E-15, 1.000000000000000000, 0.000000000000000000 ) ) ;
#35731=VERTEX_POINT ( 'NONE', #10277 ) ;
#35740=CARTESIAN_POINT ( 'NONE',  ( 70.06670417066790435, -71.37844715994097555, 55.21780685541800437 ) ) ;
#35755=ORIENTED_EDGE ( 'NONE', *, *, #1851, .T. ) ;
#35767=ORIENTED_EDGE ( 'NONE', *, *, #69390, .F. ) ;
#35779=LINE ( 'NONE', #49850, #57136 ) ;
#35785=ORIENTED_EDGE ( 'NONE', *, *, #69069, .F. ) ;
#35807=EDGE_LOOP ( 'NONE', ( #89890, #85321, #12180, #76050, #46900 ) ) ;
#35813=DIRECTION ( 'NONE',  ( 0.000000000000000000, 0.000000000000000000, -1.000000000000000000 ) ) ;
#35842=EDGE_CURVE ( 'NONE', #35871, #33311, #17973, .T. ) ;
#35844=DIRECTION ( 'NONE',  ( -0.4999999999999931166, -0.8660254037844425934, 2.684678751731770391E-14 ) ) ;
#35863=VERTEX_POINT ( 'NONE', #45221 ) ;
#35871=VERTEX_POINT ( 'NONE', #46561 ) ;
#35884=CARTESIAN_POINT ( 'NONE',  ( 106.0667039024470455, -121.2010968907524529, -19.26696060647547881 ) ) ;
#35902=VERTEX_POINT ( 'NONE', #11159 ) ;
#35910=CARTESIAN_POINT ( 'NONE',  ( 67.30555758892512586, -104.4393591762123918, 246.9440934771770060 ) ) ;
#35920=LINE ( 'NONE', #28662, #32939 ) ;
#35930=ORIENTED_EDGE ( 'NONE', *, *, #36276, .F. ) ;
#35932=B_SPLINE_CURVE_WITH_KNOTS ( 'NONE', 3,
 ( #77830, #69664, #62836, #35576, #56463, #8798, #35125, #612, #28309, #56001, #83751, #15607, #43280, #15152, #84209, #49196, #42828, #14708 ),
 .UNSPECIFIED., .F., .F.,
 ( 4, 2, 2, 2, 2, 2, 2, 2, 4 ),
 ( 0.000000000000000000, 0.1250000000000000000, 0.2500000000000000000, 0.3750000000000000000, 0.5000000000000000000, 0.6250000000000000000, 0.7500000000000000000, 0.8750000000000000000, 1.000000000000000000 ),
 .UNSPECIFIED. ) ;
#35959=CARTESIAN_POINT ( 'NONE',  ( 147.0667039024470739, -137.6766936010357938, 245.4930511039999885 ) ) ;
#35962=DIRECTION ( 'NONE',  ( 0.000000000000000000, 0.000000000000000000, 1.000000000000000000 ) ) ;
#35981=B_SPLINE_CURVE_WITH_KNOTS ( 'NONE', 3,
 ( #51964, #37475, #52397, #24733, #66506, #45158, #60125, #31093, #72881, #51527, #38354, #44268, #79277, #37919, #10214, #65619, #10648, #87410, #9772, #73322, #78828, #39253, #87859, #66053, #23855, #17037, #4295, #44717, #3844 ),
 .UNSPECIFIED., .F., .F.,
 ( 4, 2, 2, 2, 1, 1, 2, 2, 2, 2, 1, 1, 1, 2, 2, 2, 4 ),
 ( 0.000000000000000000, 0.2500000000002285949, 0.3750000000003456679, 0.4375000000003927969, 0.4687500000004163891, 0.4843750000004282130, 0.4921875000004340972, 0.5000000000004399814, 0.6250000000006787904, 0.6875000000008131273, 0.7187500000008804069, 0.7343750000009092727, 0.7421875000009192647, 0.7460937500009182655, 0.7500000000009172663, 0.8750000000004586331, 1.000000000000000000 ),
 .UNSPECIFIED. ) ;
#35985=CARTESIAN_POINT ( 'NONE',  ( 114.2313622454166904, -100.7192800061664570, -19.78219314458212708 ) ) ;
#35992=EDGE_CURVE ( 'NONE', #83707, #20491, #67920, .T. ) ;
#36005=DIRECTION ( 'NONE',  ( -1.150535366796005147E-15, 1.000000000000000000, -3.100000000000000044E-14 ) ) ;
#36009=VERTEX_POINT ( 'NONE', #82474 ) ;
#36014=CARTESIAN_POINT ( 'NONE',  ( 70.38652669525582439, -140.1242979453984390, 246.9157945169867787 ) ) ;
#36039=CARTESIAN_POINT ( 'NONE',  ( 139.9417039024470455, -127.9034471599408960, 45.21780685541799727 ) ) ;
#36042=LINE ( 'NONE', #7889, #3524 ) ;
#36052=CARTESIAN_POINT ( 'NONE',  ( 121.3140869715381314, -95.00417761012944595, -11.78219314458228695 ) ) ;
#36053=EDGE_CURVE ( 'NONE', #86385, #58881, #22858, .T. ) ;
#36069=CARTESIAN_POINT ( 'NONE',  ( 107.0667039024469886, -67.87844715994094713, 93.21780685541800437 ) ) ;
#36086=CIRCLE ( 'NONE', #46226, 3.000000000000002665 ) ;
#36100=DIRECTION ( 'NONE',  ( 0.000000000000000000, 0.000000000000000000, 1.000000000000000000 ) ) ;
#36109=ORIENTED_EDGE ( 'NONE', *, *, #67740, .T. ) ;
#36122=VERTEX_POINT ( 'NONE', #6592 ) ;
#36133=CARTESIAN_POINT ( 'NONE',  ( 52.06670390244699576, -67.87844715994100397, 55.21780685541800437 ) ) ;
#36139=CARTESIAN_POINT ( 'NONE',  ( 107.0667039024470313, -104.2784471599413934, 2.217806855418003043 ) ) ;
#36157=CARTESIAN_POINT ( 'NONE',  ( 107.0667039024470313, -104.2784471599409528, 45.21780685541799727 ) ) ;
#36159=LINE ( 'NONE', #70684, #40748 ) ;
#36162=ORIENTED_EDGE ( 'NONE', *, *, #71384, .T. ) ;
#36164=EDGE_CURVE ( 'NONE', #50049, #45547, #61994, .T. ) ;
#36168=EDGE_CURVE ( 'NONE', #44336, #40469, #27478, .T. ) ;
#36179=EDGE_LOOP ( 'NONE', ( #55323, #71213, #18134 ) ) ;
#36184=FACE_OUTER_BOUND ( 'NONE', #48972, .T. ) ;
#36186=DIRECTION ( 'NONE',  ( 0.5000000000000015543, 0.8660254037844377084, -2.688821387764056676E-14 ) ) ;
#36206=STYLED_ITEM ( 'NONE', ( #8224 ), #3408 ) ;
#36216=ORIENTED_EDGE ( 'NONE', *, *, #50859, .F. ) ;
#36226=LINE ( 'NONE', #49388, #69795 ) ;
#36241=LINE ( 'NONE', #85756, #7867 ) ;
#36245=DIRECTION ( 'NONE',  ( 1.000000000000000000, 0.000000000000000000, 0.000000000000000000 ) ) ;
#36248=DIRECTION ( 'NONE',  ( -3.100000000000000258E-29, 3.100000000000000044E-14, 1.000000000000000000 ) ) ;
#36251=CARTESIAN_POINT ( 'NONE',  ( 97.06670390244701707, -98.59953881414064369, 19.21780685541782319 ) ) ;
#36262=CARTESIAN_POINT ( 'NONE',  ( 106.0667039024470455, -121.2010968907525239, -21.78219314458149114 ) ) ;
#36269=AXIS2_PLACEMENT_3D ( 'NONE', #7834, #1027, #78251 ) ;
#36276=EDGE_CURVE ( 'NONE', #45648, #60002, #14091, .T. ) ;
#36295=ORIENTED_EDGE ( 'NONE', *, *, #22226, .F. ) ;
#36315=CIRCLE ( 'NONE', #79841, 3.499999999999996003 ) ;
#36321=CARTESIAN_POINT ( 'NONE',  ( 68.90655442492621319, -69.55252416307811814, 247.4986722481951631 ) ) ;
#36324=VECTOR ( 'NONE', #78620, 999.9999999999998863 ) ;
#36343=DIRECTION ( 'NONE',  ( 1.000000000000000000, 1.000000000000000078E-15, 0.000000000000000000 ) ) ;
#36375=EDGE_CURVE ( 'NONE', #59958, #56065, #66012, .T. ) ;
#36383=LINE ( 'NONE', #15498, #26353 ) ;
#36409=CARTESIAN_POINT ( 'NONE',  ( 119.9305508289310609, -79.89790063748476712, 250.2178068554179902 ) ) ;
#36425=DIRECTION ( 'NONE',  ( 1.000000000000000000, 0.000000000000000000, 0.000000000000000000 ) ) ;
#36446=CARTESIAN_POINT ( 'NONE',  ( 107.0667039024470171, -89.08784823670032438, -11.78219314458248057 ) ) ;
#36456=ORIENTED_EDGE ( 'NONE', *, *, #31318, .T. ) ;
#36459=ORIENTED_EDGE ( 'NONE', *, *, #52457, .T. ) ;
#36474=CARTESIAN_POINT ( 'NONE',  ( 70.61455841086757346, -139.6273172416246950, 247.2949093517953827 ) ) ;
#36478=VERTEX_POINT ( 'NONE', #84036 ) ;
#36486=CARTESIAN_POINT ( 'NONE',  ( 154.5667039024470171, -79.67844715994088745, 120.2178068554179902 ) ) ;
#36496=FACE_OUTER_BOUND ( 'NONE', #28611, .T. ) ;
#36504=EDGE_CURVE ( 'NONE', #89615, #34853, #64726, .T. ) ;
#36508=VERTEX_POINT ( 'NONE', #77665 ) ;
#36516=CARTESIAN_POINT ( 'NONE',  ( 122.2221484686746322, -104.2784471599418055, -11.78219314458200984 ) ) ;
#36520=CARTESIAN_POINT ( 'NONE',  ( 145.1595140859767810, -137.8496423039705121, 247.5170369397599757 ) ) ;
#36530=CARTESIAN_POINT ( 'NONE',  ( 74.06670390244701707, -90.27844715994098124, 230.7030882296565721 ) ) ;
#36543=CARTESIAN_POINT ( 'NONE',  ( 145.5097900936629856, -69.34210384614996769, 247.4498248016565469 ) ) ;
#36556=VERTEX_POINT ( 'NONE', #27714 ) ;
#36563=VECTOR ( 'NONE', #3628, 1000.000000000000000 ) ;
#36576=ADVANCED_FACE ( 'NONE', ( #24043 ), #79464, .T. ) ;
#36579=DIRECTION ( 'NONE',  ( 1.000000000000000000, 1.000000000000000078E-15, 0.000000000000000000 ) ) ;
#36586=EDGE_CURVE ( 'NONE', #29924, #64928, #78127, .T. ) ;
#36596=FACE_OUTER_BOUND ( 'NONE', #40216, .T. ) ;
#36606=LINE ( 'NONE', #57922, #56075 ) ;
#36645=DIRECTION ( 'NONE',  ( 0.7071067811865482389, -0.7071067811865467956, 0.000000000000000000 ) ) ;
#36648=VECTOR ( 'NONE', #21119, 1000.000000000000000 ) ;
#36650=CARTESIAN_POINT ( 'NONE',  ( 106.5667039024470171, -95.29234678213566667, 2.217806855417725487 ) ) ;
#36676=EDGE_CURVE ( 'NONE', #26317, #54219, #45827, .T. ) ;
#36688=CARTESIAN_POINT ( 'NONE',  ( 70.06670390244705970, -124.7784471599409670, 222.2178068554179902 ) ) ;
#36703=ADVANCED_FACE ( 'NONE', ( #37669 ), #71742, .T. ) ;
#36720=VECTOR ( 'NONE', #62155, 1000.000000000000000 ) ;
#36740=CARTESIAN_POINT ( 'NONE',  ( 107.0667039024470313, -104.2784471599409528, 55.21780685541800437 ) ) ;
#36774=DIRECTION ( 'NONE',  ( 0.000000000000000000, 0.000000000000000000, 1.000000000000000000 ) ) ;
#36778=AXIS2_PLACEMENT_3D ( 'NONE', #64061, #35436, #56317 ) ;
#36810=AXIS2_PLACEMENT_3D ( 'NONE', #3003, #71611, #51575 ) ;
#36821=VERTEX_POINT ( 'NONE', #73966 ) ;
#36827=ORIENTED_EDGE ( 'NONE', *, *, #79981, .F. ) ;
#36832=CARTESIAN_POINT ( 'NONE',  ( 67.06670390244707392, -137.6782278263010824, 245.4503596485529897 ) ) ;
#36843=CARTESIAN_POINT ( 'NONE',  ( 158.0667039024469886, -67.87844715994090450, 85.21780685541799016 ) ) ;
#36844=DIRECTION ( 'NONE',  ( 0.000000000000000000, 0.000000000000000000, -1.000000000000000000 ) ) ;
#36845=DIRECTION ( 'NONE',  ( 0.000000000000000000, 0.000000000000000000, 1.000000000000000000 ) ) ;
#36846=FACE_OUTER_BOUND ( 'NONE', #30963, .T. ) ;
#36859=CARTESIAN_POINT ( 'NONE',  ( 161.5667039024469886, -68.37844715994089029, 96.96780685541800437 ) ) ;
#36883=DIRECTION ( 'NONE',  ( 0.000000000000000000, 0.000000000000000000, 1.000000000000000000 ) ) ;
#36884=DIRECTION ( 'NONE',  ( 1.000000000000000000, 0.000000000000000000, 0.000000000000000000 ) ) ;
#36907=DIRECTION ( 'NONE',  ( 1.000000000000000078E-15, -1.000000000000000000, 0.000000000000000000 ) ) ;
#36919=CIRCLE ( 'NONE', #48484, 2.999999999999988898 ) ;
#36922=CARTESIAN_POINT ( 'NONE',  ( 68.88219323916185033, -139.1179055681215573, 246.6639347725188145 ) ) ;
#36944=FACE_OUTER_BOUND ( 'NONE', #65945, .T. ) ;
#36954=ORIENTED_EDGE ( 'NONE', *, *, #6776, .T. ) ;
#36961=DIRECTION ( 'NONE',  ( 1.000000000000000000, 1.000000000000000078E-15, 0.000000000000000000 ) ) ;
#36963=EDGE_CURVE ( 'NONE', #42066, #68825, #41656, .T. ) ;
#36965=EDGE_CURVE ( 'NONE', #23110, #45437, #7171, .T. ) ;
#37014=LINE ( 'NONE', #70648, #59744 ) ;
#37017=CARTESIAN_POINT ( 'NONE',  ( 74.76628479679460781, -74.85678555694860847, 248.3919653347779786 ) ) ;
#37036=CARTESIAN_POINT ( 'NONE',  ( 133.5825581355576901, -151.1625929302300051, 73.15139425029549614 ) ) ;
#37039=CARTESIAN_POINT ( 'NONE',  ( 146.5419990862876034, -137.3788609484426786, 246.8585042003560375 ) ) ;
#37052=ORIENTED_EDGE ( 'NONE', *, *, #41875, .T. ) ;
#37053=ADVANCED_FACE ( 'NONE', ( #52041 ), #9401, .F. ) ;
#37055=CIRCLE ( 'NONE', #57391, 8.999999999999994671 ) ;
#37067=VECTOR ( 'NONE', #40836, 1000.000000000000000 ) ;
#37068=PLANE ( 'NONE',  #86261 ) ;
#37085=EDGE_CURVE ( 'NONE', #30354, #25238, #66194, .T. ) ;
#37092=DIRECTION ( 'NONE',  ( 0.000000000000000000, 0.000000000000000000, 1.000000000000000000 ) ) ;
#37093=CARTESIAN_POINT ( 'NONE',  ( 85.58879520791425932, -121.5356829788755562, 250.2178068554179902 ) ) ;
#37103=VERTEX_POINT ( 'NONE', #87490 ) ;
#37120=ORIENTED_EDGE ( 'NONE', *, *, #9101, .T. ) ;
#37127=ORIENTED_EDGE ( 'NONE', *, *, #58975, .F. ) ;
#37134=VERTEX_POINT ( 'NONE', #24815 ) ;
#37135=CARTESIAN_POINT ( 'NONE',  ( 108.0667039024470171, -87.35579742913164125, -19.26696060647653397 ) ) ;
#37172=AXIS2_PLACEMENT_3D ( 'NONE', #22259, #15445, #21813 ) ;
#37177=CIRCLE ( 'NONE', #73401, 3.500000000000003109 ) ;
#37203=VERTEX_POINT ( 'NONE', #44693 ) ;
#37204=CARTESIAN_POINT ( 'NONE',  ( 103.8797721312301405, -101.8611209747514010, -19.78219314458209865 ) ) ;
#37228=CARTESIAN_POINT ( 'NONE',  ( 144.0716631786001471, -138.9592723264545953, 247.5160078862170110 ) ) ;
#37241=VECTOR ( 'NONE', #78229, 1000.000000000000000 ) ;
#37266=ORIENTED_EDGE ( 'NONE', *, *, #87474, .T. ) ;
#37267=VECTOR ( 'NONE', #58886, 1000.000000000000000 ) ;
#37268=EDGE_CURVE ( 'NONE', #58881, #23612, #15677, .T. ) ;
#37276=DIRECTION ( 'NONE',  ( 1.000000000000000000, 1.000000000000000078E-15, -0.000000000000000000 ) ) ;
#37285=EDGE_CURVE ( 'NONE', #59268, #27442, #27050, .T. ) ;
#37301=DIRECTION ( 'NONE',  ( 1.000000000000000000, 0.000000000000000000, 0.000000000000000000 ) ) ;
#37317=CARTESIAN_POINT ( 'NONE',  ( 107.0667039024470313, -104.2784471599409528, 25.71780685541800437 ) ) ;
#37335=FACE_BOUND ( 'NONE', #56786, .T. ) ;
#37337=VERTEX_POINT ( 'NONE', #88296 ) ;
#37346=CARTESIAN_POINT ( 'NONE',  ( 107.0667039024470313, -104.2784471599420471, -19.18411693322902423 ) ) ;
#37355=CARTESIAN_POINT ( 'NONE',  ( 71.06670390244701707, -90.27844715994098124, 230.7030882296565721 ) ) ;
#37377=EDGE_CURVE ( 'NONE', #44246, #34853, #46012, .T. ) ;
#37387=CIRCLE ( 'NONE', #8415, 11.49999999999999645 ) ;
#37406=VERTEX_POINT ( 'NONE', #72855 ) ;
#37420=ORIENTED_EDGE ( 'NONE', *, *, #29814, .F. ) ;
#37428=CARTESIAN_POINT ( 'NONE',  ( 83.56670390244703128, -104.2784471599409670, 23.21780685541800082 ) ) ;
#37449=DIRECTION ( 'NONE',  ( 1.777766061779359009E-15, -1.000000000000000000, 3.100000000000000044E-14 ) ) ;
#37474=CARTESIAN_POINT ( 'NONE',  ( 91.91125933621934507, -111.8737466215628160, -19.26696060647578435 ) ) ;
#37475=CARTESIAN_POINT ( 'NONE',  ( 144.0491476497456915, -140.6784470014346198, 245.7567723467967653 ) ) ;
#37481=CARTESIAN_POINT ( 'NONE',  ( 106.5667039024470313, -108.2470741265389620, -19.78219314458190681 ) ) ;
#37484=CARTESIAN_POINT ( 'NONE',  ( 67.46744162048150883, -137.4384689103915207, 246.7095008466345405 ) ) ;
#37507=( BOUNDED_CURVE ( )  B_SPLINE_CURVE ( 2, ( #86455, #65979, #24222 ),
 .UNSPECIFIED., .F., .T. ) 
 B_SPLINE_CURVE_WITH_KNOTS ( ( 3, 3 ),
 ( 0.000000000000000000, 0.5053286420056760653 ),
 .UNSPECIFIED. ) 
 CURVE ( )  GEOMETRIC_REPRESENTATION_ITEM ( )  RATIONAL_B_SPLINE_CURVE ( ( 1.000000000000000000, 1.009299002520659849, 1.000420656333769864 ) ) 
 REPRESENTATION_ITEM ( '' )  );
#37519=LINE ( 'NONE', #39288, #28269 ) ;
#37520=DIRECTION ( 'NONE',  ( -1.000000000000000000, -1.541976423090496028E-15, 0.000000000000000000 ) ) ;
#37537=ORIENTED_EDGE ( 'NONE', *, *, #13524, .F. ) ;
#37542=CARTESIAN_POINT ( 'NONE',  ( 79.72329571771361145, -100.8945472140120501, 250.2178068554180470 ) ) ;
#37579=CARTESIAN_POINT ( 'NONE',  ( 91.91125933621933086, -96.68314769832132072, -19.26696060647622843 ) ) ;
#37582=CARTESIAN_POINT ( 'NONE',  ( 59.56670390244699576, -67.87844715994098976, 85.21780685541799016 ) ) ;
#37610=CARTESIAN_POINT ( 'NONE',  ( 151.0667039024469886, -79.67844715994088745, 155.2178068554179902 ) ) ;
#37613=EDGE_CURVE ( 'NONE', #74740, #8011, #42628, .T. ) ;
#37620=FACE_OUTER_BOUND ( 'NONE', #61966, .T. ) ;
#37650=VERTEX_POINT ( 'NONE', #78089 ) ;
#37656=B_SPLINE_CURVE_WITH_KNOTS ( 'NONE', 3,
 ( #48348, #47010, #82029, #13861, #26588, #76084 ),
 .UNSPECIFIED., .F., .F.,
 ( 4, 2, 4 ),
 ( 0.000000000000000000, 0.0009145665419566550210, 0.001828735834957770194 ),
 .UNSPECIFIED. ) ;
#37662=CARTESIAN_POINT ( 'NONE',  ( 96.67439905703393777, -115.7784471599421323, -21.78219314458165812 ) ) ;
#37663=CARTESIAN_POINT ( 'NONE',  ( 89.89934876040919676, -68.97671693066587295, 247.5435304005999910 ) ) ;
#37669=FACE_OUTER_BOUND ( 'NONE', #15844, .T. ) ;
#37670=EDGE_LOOP ( 'NONE', ( #8216, #71112, #18142, #41428 ) ) ;
#37675=CARTESIAN_POINT ( 'NONE',  ( 162.0667039024469886, -67.87844715994089029, 222.2178068554179902 ) ) ;
#37680=CARTESIAN_POINT ( 'NONE',  ( 145.5504341359485636, -139.1947169264394120, 246.0943807925750093 ) ) ;
#37681=CARTESIAN_POINT ( 'NONE',  ( 124.0667039024470313, -106.9675116026789254, -9.937637710809946512 ) ) ;
#37691=DIRECTION ( 'NONE',  ( 0.3535533905932745080, -0.6123724356957719328, 0.7071067811865667796 ) ) ;
#37692=CARTESIAN_POINT ( 'NONE',  ( 118.5667039024470313, -104.2784471599408533, 19.21780685541799016 ) ) ;
#37708=DIRECTION ( 'NONE',  ( -0.8660254037844392627, 0.4999999999999990008, -1.549999999999999706E-14 ) ) ;
#37714=DIRECTION ( 'NONE',  ( 0.8660254037844392627, -0.4999999999999990008, 1.549999999999999706E-14 ) ) ;
#37753=AXIS2_PLACEMENT_3D ( 'NONE', #37582, #11201, #17580 ) ;
#37775=EDGE_CURVE ( 'NONE', #35252, #57634, #43080, .T. ) ;
#37777=PLANE ( 'NONE',  #43923 ) ;
#37790=ORIENTED_EDGE ( 'NONE', *, *, #6036, .F. ) ;
#37794=EDGE_LOOP ( 'NONE', ( #13044, #10727, #41515, #46809 ) ) ;
#37801=EDGE_CURVE ( 'NONE', #73518, #33311, #31501, .T. ) ;
#37805=AXIS2_PLACEMENT_3D ( 'NONE', #60382, #39505, #26325 ) ;
#37820=CARTESIAN_POINT ( 'NONE',  ( 69.57274467425236253, -138.4326786319161329, 247.5388220368722045 ) ) ;
#37828=B_SPLINE_CURVE_WITH_KNOTS ( 'NONE', 3,
 ( #44277, #73785, #86542, #9781 ),
 .UNSPECIFIED., .F., .F.,
 ( 4, 4 ),
 ( -0.3438257506183129975, -0.1481392554759810298 ),
 .UNSPECIFIED. ) ;
#37829=FACE_BOUND ( 'NONE', #82975, .T. ) ;
#37837=ORIENTED_EDGE ( 'NONE', *, *, #85582, .F. ) ;
#37851=DIRECTION ( 'NONE',  ( 1.000000000000000000, 0.000000000000000000, 0.000000000000000000 ) ) ;
#37855=VERTEX_POINT ( 'NONE', #12202 ) ;
#37860=CARTESIAN_POINT ( 'NONE',  ( 68.06670390244705970, -121.7784471599409954, 55.21780685541800437 ) ) ;
#37874=CARTESIAN_POINT ( 'NONE',  ( 97.08661802161040555, -77.52859162019140626, 250.2201230397200220 ) ) ;
#37876=CARTESIAN_POINT ( 'NONE',  ( 120.2221484686747317, -111.8737466215625602, -11.78219314458178779 ) ) ;
#37907=DIRECTION ( 'NONE',  ( -1.000000000000000000, -1.206764157201257538E-15, 0.000000000000000000 ) ) ;
#37919=CARTESIAN_POINT ( 'NONE',  ( 143.7437383847394301, -140.1181772184977490, 246.9254612266167612 ) ) ;
#37932=ORIENTED_EDGE ( 'NONE', *, *, #18, .F. ) ;
#37944=CARTESIAN_POINT ( 'NONE',  ( 70.06670417066790435, -69.62844715994098976, 222.2178068554179902 ) ) ;
#37952=AXIS2_PLACEMENT_3D ( 'NONE', #84757, #34787, #42930 ) ;
#37954=DIRECTION ( 'NONE',  ( -1.000000000000000078E-15, 1.000000000000000000, 0.000000000000000000 ) ) ;
#37964=DIRECTION ( 'NONE',  ( 0.000000000000000000, 0.000000000000000000, 1.000000000000000000 ) ) ;
#37972=DIRECTION ( 'NONE',  ( -1.000000000000000078E-15, 1.000000000000000000, 0.000000000000000000 ) ) ;
#37975=CARTESIAN_POINT ( 'NONE',  ( 84.56587091301774706, -88.37796714256990072, 250.2178068554180470 ) ) ;
#37977=AXIS2_PLACEMENT_3D ( 'NONE', #63374, #50631, #36579 ) ;
#37978=EDGE_CURVE ( 'NONE', #64854, #16883, #77966, .T. ) ;
#37984=DIRECTION ( 'NONE',  ( 1.000000000000000000, 0.000000000000000000, 0.000000000000000000 ) ) ;
#37988=VECTOR ( 'NONE', #41296, 1000.000000000000000 ) ;
#38020=ORIENTED_EDGE ( 'NONE', *, *, #68766, .F. ) ;
#38022=( BOUNDED_CURVE ( )  B_SPLINE_CURVE ( 2, ( #39371, #38916, #79390 ),
 .UNSPECIFIED., .F., .T. ) 
 B_SPLINE_CURVE_WITH_KNOTS ( ( 3, 3 ),
 ( 0.01169420784673960018, 0.5170228498526600047 ),
 .UNSPECIFIED. ) 
 CURVE ( )  GEOMETRIC_REPRESENTATION_ITEM ( )  RATIONAL_B_SPLINE_CURVE ( ( 1.000420656333759872, 1.009299002520659849, 1.000000000000000000 ) ) 
 REPRESENTATION_ITEM ( '' )  );
#38033=ORIENTED_EDGE ( 'NONE', *, *, #87139, .F. ) ;
#38069=LINE ( 'NONE', #24889, #28213 ) ;
#38100=EDGE_CURVE ( 'NONE', #37203, #82603, #24826, .T. ) ;
#38102=CARTESIAN_POINT ( 'NONE',  ( 147.0665937085389032, -67.87844715994090450, 245.5130139786259917 ) ) ;
#38109=DIRECTION ( 'NONE',  ( -0.8660254037844392627, 0.4999999999999990008, -1.549999999999999706E-14 ) ) ;
#38110=EDGE_LOOP ( 'NONE', ( #12367, #46909, #56425, #23372 ) ) ;
#38123=EDGE_CURVE ( 'NONE', #60056, #47600, #66595, .T. ) ;
#38140=EDGE_LOOP ( 'NONE', ( #9403, #18368, #11188, #69345 ) ) ;
#38142=CARTESIAN_POINT ( 'NONE',  ( 107.0667039024469886, -70.87844715994094713, 93.21780685541800437 ) ) ;
#38163=DIRECTION ( 'NONE',  ( -1.000000000000000000, -1.734723475976808672E-15, 0.000000000000000000 ) ) ;
#38189=AXIS2_PLACEMENT_3D ( 'NONE', #20038, #48600, #12322 ) ;
#38209=LINE ( 'NONE', #17767, #44151 ) ;
#38210=ADVANCED_FACE ( 'NONE', ( #75217 ), #55971, .T. ) ;
#38217=ADVANCED_FACE ( 'NONE', ( #70076 ), #26169, .F. ) ;
#38234=DIRECTION ( 'NONE',  ( -1.000000000000000000, -8.163404592832032979E-16, 0.000000000000000000 ) ) ;
#38235=DIRECTION ( 'NONE',  ( -3.100000000000000258E-29, 3.100000000000000044E-14, 1.000000000000000000 ) ) ;
#38241=CARTESIAN_POINT ( 'NONE',  ( 107.0667039024470313, -104.2784471599409528, 22.21780685541800082 ) ) ;
#38245=EDGE_CURVE ( 'NONE', #9096, #77101, #46587, .T. ) ;
#38255=CARTESIAN_POINT ( 'NONE',  ( 69.32970740376067909, -138.6740805926116593, 247.3339793106913760 ) ) ;
#38282=PLANE ( 'NONE',  #38516 ) ;
#38294=DIRECTION ( 'NONE',  ( 3.100000000000000258E-29, -3.100000000000000044E-14, -1.000000000000000000 ) ) ;
#38295=ADVANCED_FACE ( 'NONE', ( #8303 ), #12543, .F. ) ;
#38306=CARTESIAN_POINT ( 'NONE',  ( 124.2517790421138102, -76.23676170112041461, 249.3134381260879877 ) ) ;
#38311=PLANE ( 'NONE',  #62550 ) ;
#38316=EDGE_LOOP ( 'NONE', ( #73296, #72755, #59668, #72709 ) ) ;
#38334=VECTOR ( 'NONE', #51638, 1000.000000000000000 ) ;
#38336=AXIS2_PLACEMENT_3D ( 'NONE', #40701, #55203, #27524 ) ;
#38345=ORIENTED_EDGE ( 'NONE', *, *, #72068, .F. ) ;
#38354=CARTESIAN_POINT ( 'NONE',  ( 143.7865590713107338, -140.2063866955903393, 246.8245229315576807 ) ) ;
#38365=EDGE_LOOP ( 'NONE', ( #73036, #27900 ) ) ;
#38391=ORIENTED_EDGE ( 'NONE', *, *, #72483, .F. ) ;
#38395=VECTOR ( 'NONE', #35371, 999.9999999999998863 ) ;
#38417=ORIENTED_EDGE ( 'NONE', *, *, #69091, .T. ) ;
#38418=ORIENTED_EDGE ( 'NONE', *, *, #53536, .T. ) ;
#38480=CARTESIAN_POINT ( 'NONE',  ( 140.0667039024470171, -90.27844715994091018, 230.7030882296565721 ) ) ;
#38492=EDGE_CURVE ( 'NONE', #87073, #17863, #46366, .T. ) ;
#38516=AXIS2_PLACEMENT_3D ( 'NONE', #51886, #79642, #66426 ) ;
#38517=VECTOR ( 'NONE', #68692, 1000.000000000000000 ) ;
#38525=EDGE_CURVE ( 'NONE', #11319, #753, #32759, .T. ) ;
#38530=ADVANCED_FACE ( 'NONE', ( #53622 ), #88643, .F. ) ;
#38539=CARTESIAN_POINT ( 'NONE',  ( 147.0789628650053089, -69.17499946017579759, 247.4285673639549827 ) ) ;
#38543=DIRECTION ( 'NONE',  ( -0.7071067811865463515, -0.7071067811865487940, 0.000000000000000000 ) ) ;
#38546=ORIENTED_EDGE ( 'NONE', *, *, #39896, .F. ) ;
#38548=ORIENTED_EDGE ( 'NONE', *, *, #52113, .T. ) ;
#38553=CARTESIAN_POINT ( 'NONE',  ( 74.68590766205718978, -67.87844715994097555, 245.5622121773279787 ) ) ;
#38597=DIRECTION ( 'NONE',  ( 1.000000000000000000, 0.000000000000000000, 0.000000000000000000 ) ) ;
#38611=VERTEX_POINT ( 'NONE', #40 ) ;
#38625=ORIENTED_EDGE ( 'NONE', *, *, #22638, .F. ) ;
#38643=CARTESIAN_POINT ( 'NONE',  ( 115.0439452383991892, -99.09543445804983719, -19.78219314458218392 ) ) ;
#38649=ORIENTED_EDGE ( 'NONE', *, *, #83858, .F. ) ;
#38669=ORIENTED_EDGE ( 'NONE', *, *, #22463, .F. ) ;
#38678=VERTEX_POINT ( 'NONE', #69980 ) ;
#38679=DIRECTION ( 'NONE',  ( 0.000000000000000000, 0.000000000000000000, -1.000000000000000000 ) ) ;
#38687=ORIENTED_EDGE ( 'NONE', *, *, #19453, .F. ) ;
#38692=CARTESIAN_POINT ( 'NONE',  ( 68.74524693519704499, -139.2530727251857456, 246.1985092402615862 ) ) ;
#38699=CARTESIAN_POINT ( 'NONE',  ( 145.6354771369172170, -101.1103950255152171, 247.6425393530529959 ) ) ;
#38727=CARTESIAN_POINT ( 'NONE',  ( 107.0667039024470313, -104.2784471599418197, -11.78219314458200984 ) ) ;
#38739=CARTESIAN_POINT ( 'NONE',  ( 107.0667039024470313, -104.2784471599413791, 2.217806855418003043 ) ) ;
#38749=CARTESIAN_POINT ( 'NONE',  ( 146.8415613695535171, -68.09268944053143002, 246.4109134068758067 ) ) ;
#38751=CARTESIAN_POINT ( 'NONE',  ( 115.0439452383992318, -109.4614598618342853, -19.78219314458184996 ) ) ;
#38760=EDGE_LOOP ( 'NONE', ( #63978, #48879, #70858 ) ) ;
#38773=VECTOR ( 'NONE', #65079, 1000.000000000000114 ) ;
#38807=CARTESIAN_POINT ( 'NONE',  ( 71.06670390244701707, -90.27844715994098124, 222.2178068554179902 ) ) ;
#38825=DIRECTION ( 'NONE',  ( 3.100000000000000258E-29, -3.100000000000000044E-14, -1.000000000000000000 ) ) ;
#38828=VERTEX_POINT ( 'NONE', #56778 ) ;
#38829=EDGE_LOOP ( 'NONE', ( #60278, #84943, #2532, #76537, #5253 ) ) ;
#38848=CARTESIAN_POINT ( 'NONE',  ( 154.4628380807770327, -130.5939552399572108, 126.9238073912448925 ) ) ;
#38865=EDGE_CURVE ( 'NONE', #69445, #41770, #71772, .T. ) ;
#38877=VECTOR ( 'NONE', #28786, 1000.000000000000000 ) ;
#38879=ORIENTED_EDGE ( 'NONE', *, *, #37801, .F. ) ;
#38887=CARTESIAN_POINT ( 'NONE',  ( 87.68693475024628015, -140.6784471599409585, 245.6812587119739817 ) ) ;
#38897=B_SPLINE_CURVE_WITH_KNOTS ( 'NONE', 3,
 ( #31683, #60721, #33477, #3986 ),
 .UNSPECIFIED., .F., .F.,
 ( 4, 4 ),
 ( -0.6035999334370359959, -0.5903216970416030884 ),
 .UNSPECIFIED. ) ;
#38913=DIRECTION ( 'NONE',  ( -1.000000000000000078E-15, 1.000000000000000000, 0.000000000000000000 ) ) ;
#38916=CARTESIAN_POINT ( 'NONE',  ( 104.1009375265828538, -120.0661611444834023, -21.02845593540877189 ) ) ;
#38922=ORIENTED_EDGE ( 'NONE', *, *, #60951, .T. ) ;
#38924=DIRECTION ( 'NONE',  ( -1.000000000000000000, -1.541976423090496028E-15, 0.000000000000000000 ) ) ;
#38931=CARTESIAN_POINT ( 'NONE',  ( 52.06670390244699576, -68.87844715994100397, 55.21780685541800437 ) ) ;
#38938=CARTESIAN_POINT ( 'NONE',  ( 140.0667039024470171, -90.27844715994091018, 51.21780685541800437 ) ) ;
#38940=LINE ( 'NONE', #69230, #78096 ) ;
#38942=CARTESIAN_POINT ( 'NONE',  ( 77.10067130038136440, -139.0587715636908683, 247.5465134696939913 ) ) ;
#38944=LINE ( 'NONE', #67102, #41299 ) ;
#38952=CARTESIAN_POINT ( 'NONE',  ( 137.0667039024470739, -118.2784471599408960, 230.7030882296565721 ) ) ;
#38959=VERTEX_POINT ( 'NONE', #51740 ) ;
#38964=EDGE_CURVE ( 'NONE', #81381, #3053, #56731, .T. ) ;
#38983=FACE_OUTER_BOUND ( 'NONE', #29407, .T. ) ;
#38992=ORIENTED_EDGE ( 'NONE', *, *, #10072, .F. ) ;
#38995=DIRECTION ( 'NONE',  ( 1.000000000000000000, 1.000000000000000078E-15, 0.000000000000000000 ) ) ;
#39007=EDGE_LOOP ( 'NONE', ( #89531, #14122, #34807, #54570, #2587, #25597 ) ) ;
#39014=CARTESIAN_POINT ( 'NONE',  ( 121.2542869028164176, -94.96965202435542608, -19.23816181211529397 ) ) ;
#39022=ORIENTED_EDGE ( 'NONE', *, *, #37775, .T. ) ;
#39031=ORIENTED_EDGE ( 'NONE', *, *, #12561, .F. ) ;
#39045=ORIENTED_EDGE ( 'NONE', *, *, #31635, .T. ) ;
#39070=ORIENTED_EDGE ( 'NONE', *, *, #20270, .T. ) ;
#39073=CARTESIAN_POINT ( 'NONE',  ( 67.06670390244701707, -79.67844715994098692, 55.21780685541800437 ) ) ;
#39076=FACE_OUTER_BOUND ( 'NONE', #7891, .T. ) ;
#39080=DIRECTION ( 'NONE',  ( -3.100000000000000258E-29, 3.100000000000000044E-14, 1.000000000000000000 ) ) ;
#39084=VERTEX_POINT ( 'NONE', #6294 ) ;
#39097=DIRECTION ( 'NONE',  ( 1.000000000000000000, 8.953411488912556626E-16, 0.000000000000000000 ) ) ;
#39101=ORIENTED_EDGE ( 'NONE', *, *, #38245, .T. ) ;
#39104=CARTESIAN_POINT ( 'NONE',  ( 97.06670390244703128, -104.2784471599409244, 17.71780685541799016 ) ) ;
#39131=CARTESIAN_POINT ( 'NONE',  ( 71.69596173992542276, -99.94637129117697327, 248.3919653347779786 ) ) ;
#39134=CARTESIAN_POINT ( 'NONE',  ( 107.0667039024470313, -104.2784471599420755, -19.78219314458201694 ) ) ;
#39137=FACE_OUTER_BOUND ( 'NONE', #43802, .T. ) ;
#39140=CARTESIAN_POINT ( 'NONE',  ( 104.0667030381796963, -70.87844715994094713, 93.21780742166239975 ) ) ;
#39142=FACE_OUTER_BOUND ( 'NONE', #78045, .T. ) ;
#39147=DIRECTION ( 'NONE',  ( 0.000000000000000000, 0.000000000000000000, 1.000000000000000000 ) ) ;
#39152=EDGE_CURVE ( 'NONE', #45292, #66416, #35779, .T. ) ;
#39179=DIRECTION ( 'NONE',  ( -3.100000000000000258E-29, 3.100000000000000044E-14, 1.000000000000000000 ) ) ;
#39182=ORIENTED_EDGE ( 'NONE', *, *, #86849, .T. ) ;
#39197=ORIENTED_EDGE ( 'NONE', *, *, #86507, .T. ) ;
#39198=CARTESIAN_POINT ( 'NONE',  ( 111.1574783714308978, -73.49652949099265697, 249.3134381260879877 ) ) ;
#39227=EDGE_CURVE ( 'NONE', #87130, #44336, #36241, .T. ) ;
#39244=AXIS2_PLACEMENT_3D ( 'NONE', #13346, #60578, #41033 ) ;
#39248=ORIENTED_EDGE ( 'NONE', *, *, #68560, .T. ) ;
#39253=CARTESIAN_POINT ( 'NONE',  ( 143.5351098994992469, -139.6638757450721755, 247.2744478881182317 ) ) ;
#39261=CARTESIAN_POINT ( 'NONE',  ( 68.06364636000260759, -137.1614519753756838, 247.2373024094184188 ) ) ;
#39277=FACE_OUTER_BOUND ( 'NONE', #28484, .T. ) ;
#39288=CARTESIAN_POINT ( 'NONE',  ( 110.7536356736639220, -105.8297479413482733, -19.78219314458196010 ) ) ;
#39299=DIRECTION ( 'NONE',  ( -1.087812297297669405E-15, 1.000000000000000000, -3.100000000000000044E-14 ) ) ;
#39302=DIRECTION ( 'NONE',  ( 0.5000000000000016653, -0.8660254037844377084, 2.684678751731758716E-14 ) ) ;
#39306=CARTESIAN_POINT ( 'NONE',  ( 67.06801713577654311, -67.87892521913008181, 245.5556493635576487 ) ) ;
#39320=AXIS2_PLACEMENT_3D ( 'NONE', #27327, #73688, #66868 ) ;
#39331=EDGE_LOOP ( 'NONE', ( #73402, #78485, #20706, #24098 ) ) ;
#39333=ADVANCED_FACE ( 'NONE', ( #18018 ), #74338, .F. ) ;
#39342=B_SPLINE_SURFACE_WITH_KNOTS ( 'NONE', 3, 3, ( 
 ( #65549, #17405, #15629, #86016 ),
 ( #51453, #23789, #36520, #50572 ),
 ( #16960, #51888, #84678, #85575 ),
 ( #71047, #1992, #50117, #71494 ),
 ( #8822, #77853, #31025, #79647 ) ),
 .UNSPECIFIED., .F., .F., .F.,
 ( 4, 1, 4 ),
 ( 4, 4 ),
 ( -2.333654191434229903E-06, 0.5714285714285709528, 1.000000000000000000 ),
 ( 0.1538195221703859972, 0.4047106084325320374 ),
 .UNSPECIFIED. ) ;
#39343=LINE ( 'NONE', #51619, #65472 ) ;
#39356=LINE ( 'NONE', #73876, #2648 ) ;
#39371=CARTESIAN_POINT ( 'NONE',  ( 106.0667039024470455, -121.2010968907524529, -19.26696060647547881 ) ) ;
#39381=EDGE_CURVE ( 'NONE', #36556, #75352, #45269, .T. ) ;
#39388=AXIS2_PLACEMENT_3D ( 'NONE', #84992, #25750, #53427 ) ;
#39398=ORIENTED_EDGE ( 'NONE', *, *, #51410, .F. ) ;
#39400=EDGE_LOOP ( 'NONE', ( #52974, #4069, #64714, #14851 ) ) ;
#39406=DIRECTION ( 'NONE',  ( -1.000000000000000000, -1.206764157201257538E-15, 0.000000000000000000 ) ) ;
#39416=FACE_OUTER_BOUND ( 'NONE', #49066, .T. ) ;
#39438=CARTESIAN_POINT ( 'NONE',  ( 143.2674661430137917, -68.27559814658837922, 247.0029128788180230 ) ) ;
#39482=CARTESIAN_POINT ( 'NONE',  ( 107.9678037105606023, -87.30234574837474781, -19.18411693322955003 ) ) ;
#39484=VERTEX_POINT ( 'NONE', #27521 ) ;
#39497=DIRECTION ( 'NONE',  ( -1.000000000000000078E-15, 1.000000000000000000, 0.000000000000000000 ) ) ;
#39505=DIRECTION ( 'NONE',  ( 1.000000000000000000, 1.000000000000000078E-15, -0.000000000000000000 ) ) ;
#39510=LINE ( 'NONE', #13159, #5596 ) ;
#39531=DIRECTION ( 'NONE',  ( -1.000000000000000078E-15, 1.000000000000000000, 0.000000000000000000 ) ) ;
#39540=DIRECTION ( 'NONE',  ( -0.7759704746411383303, 0.6307692307692303046, 0.000000000000000000 ) ) ;
#39556=PLANE ( 'NONE',  #27734 ) ;
#39568=DIRECTION ( 'NONE',  ( 3.100000000000000258E-29, -3.100000000000000044E-14, -1.000000000000000000 ) ) ;
#39580=CARTESIAN_POINT ( 'NONE',  ( 139.2773854306074668, -133.5313011236452212, 248.4142799812389910 ) ) ;
#39581=CARTESIAN_POINT ( 'NONE',  ( 68.76551873680897131, -137.6861246176283942, 247.4844277398459838 ) ) ;
#39594=CARTESIAN_POINT ( 'NONE',  ( 145.3678890680851623, -137.6861246176283089, 247.4844277398459838 ) ) ;
#39619=DIRECTION ( 'NONE',  ( 1.000000000000000078E-15, -1.000000000000000000, 0.000000000000000000 ) ) ;
#39623=EDGE_CURVE ( 'NONE', #76096, #32183, #87370, .T. ) ;
#39628=VECTOR ( 'NONE', #72246, 1000.000000000000000 ) ;
#39632=CYLINDRICAL_SURFACE ( 'NONE', #42924, 2.000000000000001776 ) ;
#39644=DIRECTION ( 'NONE',  ( 0.4999999999999998335, 0.8660254037844387076, -2.684678751731758400E-14 ) ) ;
#39673=VECTOR ( 'NONE', #65391, 1000.000000000000000 ) ;
#39677=DIRECTION ( 'NONE',  ( -2.195856868753399715E-16, -1.000000000000000000, 0.000000000000000000 ) ) ;
#39695=CARTESIAN_POINT ( 'NONE',  ( 98.58946256649485917, -108.5954344580498514, -19.78219314458187839 ) ) ;
#39698=DIRECTION ( 'NONE',  ( 1.000000000000000078E-15, -1.000000000000000000, 0.000000000000000000 ) ) ;
#39700=DIRECTION ( 'NONE',  ( -1.000000000000000000, -8.163404592832032979E-16, 0.000000000000000000 ) ) ;
#39707=PLANE ( 'NONE',  #69246 ) ;
#39745=ORIENTED_EDGE ( 'NONE', *, *, #48437, .F. ) ;
#39752=AXIS2_PLACEMENT_3D ( 'NONE', #8044, #28944, #55267 ) ;
#39760=ORIENTED_EDGE ( 'NONE', *, *, #19731, .F. ) ;
#39768=ORIENTED_EDGE ( 'NONE', *, *, #11458, .F. ) ;
#39769=ORIENTED_EDGE ( 'NONE', *, *, #52457, .F. ) ;
#39777=DIRECTION ( 'NONE',  ( -3.100000000000000258E-29, 3.100000000000000044E-14, 1.000000000000000000 ) ) ;
#39800=DIRECTION ( 'NONE',  ( 1.000000000000000078E-15, -1.000000000000000000, 0.000000000000000000 ) ) ;
#39805=DIRECTION ( 'NONE',  ( -1.000000000000000078E-15, 1.000000000000000000, 0.000000000000000000 ) ) ;
#39810=ADVANCED_FACE ( 'NONE', ( #36596 ), #19530, .T. ) ;
#39819=EDGE_CURVE ( 'NONE', #37855, #80877, #62931, .T. ) ;
#39830=CARTESIAN_POINT ( 'NONE',  ( 145.3595637443018234, -69.45303146431501773, 247.4784022495120155 ) ) ;
#39831=CARTESIAN_POINT ( 'NONE',  ( 144.1872411114284773, -138.0587426716868151, 247.6570821702239869 ) ) ;
#39839=EDGE_CURVE ( 'NONE', #37337, #74190, #35981, .T. ) ;
#39843=VECTOR ( 'NONE', #22512, 1000.000000000000000 ) ;
#39852=ORIENTED_EDGE ( 'NONE', *, *, #87544, .T. ) ;
#39885=DIRECTION ( 'NONE',  ( 0.000000000000000000, 0.000000000000000000, 1.000000000000000000 ) ) ;
#39896=EDGE_CURVE ( 'NONE', #41501, #64928, #36919, .T. ) ;
#39926=AXIS2_PLACEMENT_3D ( 'NONE', #59997, #53168, #38234 ) ;
#39933=ORIENTED_EDGE ( 'NONE', *, *, #6124, .F. ) ;
#39934=ADVANCED_FACE ( 'NONE', ( #86532 ), #58786, .T. ) ;
#39939=DIRECTION ( 'NONE',  ( 0.5000000000000008882, -0.8660254037844382635, 2.684678751731760294E-14 ) ) ;
#39947=AXIS2_PLACEMENT_3D ( 'NONE', #31023, #51450, #87780 ) ;
#39950=DIRECTION ( 'NONE',  ( 0.000000000000000000, 0.000000000000000000, 1.000000000000000000 ) ) ;
#39954=EDGE_LOOP ( 'NONE', ( #47708, #49563, #74539, #10640 ) ) ;
#39988=CIRCLE ( 'NONE', #63212, 4.000000000000006217 ) ;
#39997=EDGE_LOOP ( 'NONE', ( #45468, #36459, #78252, #74112 ) ) ;
#40012=DIRECTION ( 'NONE',  ( 1.000000000000000000, 0.000000000000000000, 0.000000000000000000 ) ) ;
#40015=ORIENTED_EDGE ( 'NONE', *, *, #58094, .T. ) ;
#40027=ORIENTED_EDGE ( 'NONE', *, *, #15251, .F. ) ;
#40029=CARTESIAN_POINT ( 'NONE',  ( 89.89403304293395536, -132.3042147552770302, 249.3173333679100097 ) ) ;
#40042=CARTESIAN_POINT ( 'NONE',  ( 108.0667039024470455, -121.2010968907524529, -19.26696060647547881 ) ) ;
#40049=LINE ( 'NONE', #61388, #7335 ) ;
#40065=CARTESIAN_POINT ( 'NONE',  ( 63.06670390244699576, -67.87844715994098976, 120.2178068554179902 ) ) ;
#40083=PRODUCT_DEFINITION_SHAPE ( 'NONE', 'NONE',  #69989 ) ;
#40091=CARTESIAN_POINT ( 'NONE',  ( 95.83872823098278104, -90.36568251306732691, -9.274842254011060660 ) ) ;
#40108=LINE ( 'NONE', #80133, #84222 ) ;
#40112=EDGE_CURVE ( 'NONE', #29186, #70844, #7934, .T. ) ;
#40130=ORIENTED_EDGE ( 'NONE', *, *, #37613, .T. ) ;
#40141=DIRECTION ( 'NONE',  ( -1.000000000000000000, -1.000000000000000078E-15, 0.000000000000000000 ) ) ;
#40144=ADVANCED_FACE ( 'NONE', ( #8325 ), #14245, .T. ) ;
#40145=PLANE ( 'NONE',  #81163 ) ;
#40154=VECTOR ( 'NONE', #58656, 1000.000000000000000 ) ;
#40184=DIRECTION ( 'NONE',  ( 1.000000000000000078E-15, -1.000000000000000000, 0.000000000000000000 ) ) ;
#40216=EDGE_LOOP ( 'NONE', ( #13537, #73079, #70827, #77888, #30485, #35605 ) ) ;
#40220=ORIENTED_EDGE ( 'NONE', *, *, #35214, .T. ) ;
#40221=ORIENTED_EDGE ( 'NONE', *, *, #14758, .F. ) ;
#40224=EDGE_CURVE ( 'NONE', #56759, #69797, #7869, .T. ) ;
#40285=EDGE_CURVE ( 'NONE', #81699, #38611, #66235, .T. ) ;
#40328=VERTEX_POINT ( 'NONE', #88107 ) ;
#40334=EDGE_CURVE ( 'NONE', #52825, #45687, #67188, .T. ) ;
#40346=CIRCLE ( 'NONE', #33152, 4.000000000000002665 ) ;
#40348=EDGE_CURVE ( 'NONE', #85102, #35902, #60467, .T. ) ;
#40380=AXIS2_PLACEMENT_3D ( 'NONE', #16876, #44556, #85493 ) ;
#40386=PLANE ( 'NONE',  #55719 ) ;
#40391=CARTESIAN_POINT ( 'NONE',  ( 107.0667039024470313, -104.2784471599421323, -21.78219314458201694 ) ) ;
#40398=LINE ( 'NONE', #5893, #37067 ) ;
#40408=VECTOR ( 'NONE', #70621, 1000.000000000000000 ) ;
#40417=ORIENTED_EDGE ( 'NONE', *, *, #26882, .F. ) ;
#40436=LINE ( 'NONE', #82249, #53535 ) ;
#40443=DIRECTION ( 'NONE',  ( 0.000000000000000000, 0.000000000000000000, -1.000000000000000000 ) ) ;
#40469=VERTEX_POINT ( 'NONE', #75807 ) ;
#40493=CARTESIAN_POINT ( 'NONE',  ( 107.0667039024470313, -104.2784471599413934, 2.217806855418003043 ) ) ;
#40494=FACE_OUTER_BOUND ( 'NONE', #13097, .T. ) ;
#40500=CARTESIAN_POINT ( 'NONE',  ( 147.0662307635748220, -124.3843534097310055, 246.1014443220830117 ) ) ;
#40502=ORIENTED_EDGE ( 'NONE', *, *, #14423, .F. ) ;
#40520=CARTESIAN_POINT ( 'NONE',  ( 69.36073695985297149, -137.4541704093869043, 247.5777870314779818 ) ) ;
#40525=AXIS2_PLACEMENT_3D ( 'NONE', #73434, #31200, #9883 ) ;
#40528=EDGE_CURVE ( 'NONE', #86394, #71994, #56228, .T. ) ;
#40535=DIRECTION ( 'NONE',  ( -3.100000000000000258E-29, 3.100000000000000044E-14, 1.000000000000000000 ) ) ;
#40585=CIRCLE ( 'NONE', #14281, 3.500000000000003109 ) ;
#40586=AXIS2_PLACEMENT_3D ( 'NONE', #83721, #26181, #56438 ) ;
#40593=SURFACE_STYLE_FILL_AREA ( #12904 ) ;
#40601=CARTESIAN_POINT ( 'NONE',  ( 92.81932083335593120, -113.5527167097541934, -11.78219314458173272 ) ) ;
#40615=FACE_OUTER_BOUND ( 'NONE', #31841, .T. ) ;
#40618=CYLINDRICAL_SURFACE ( 'NONE', #12318, 3.499999999999996003 ) ;
#40622=MECHANICAL_DESIGN_GEOMETRIC_PRESENTATION_REPRESENTATION('',(#72532),#29029);
#40628=CARTESIAN_POINT ( 'NONE',  ( 107.5667039024470171, -95.29234678213566667, 2.217806855417725487 ) ) ;
#40667=EDGE_CURVE ( 'NONE', #11533, #70410, #56689, .T. ) ;
#40691=ORIENTED_EDGE ( 'NONE', *, *, #71641, .F. ) ;
#40694=ORIENTED_EDGE ( 'NONE', *, *, #86615, .F. ) ;
#40701=CARTESIAN_POINT ( 'NONE',  ( 107.0667039024470313, -104.2784471599413934, 2.217806855418003043 ) ) ;
#40710=CARTESIAN_POINT ( 'NONE',  ( 106.5667039024470171, -94.77844715994206126, -19.78219314458232247 ) ) ;
#40734=EDGE_LOOP ( 'NONE', ( #11605, #43279, #83406, #82299 ) ) ;
#40745=CIRCLE ( 'NONE', #39320, 3.999999999999992895 ) ;
#40748=VECTOR ( 'NONE', #35248, 1000.000000000000000 ) ;
#40769=VECTOR ( 'NONE', #69705, 1000.000000000000000 ) ;
#40773=CARTESIAN_POINT ( 'NONE',  ( 112.7927988201233944, -69.16395658370822730, 247.7076816059330042 ) ) ;
#40778=LINE ( 'NONE', #68502, #1934 ) ;
#40779=ORIENTED_EDGE ( 'NONE', *, *, #24991, .T. ) ;
#40788=CARTESIAN_POINT ( 'NONE',  ( 104.0667030381796963, -70.87844715994094713, 93.21780742166239975 ) ) ;
#40800=CARTESIAN_POINT ( 'NONE',  ( 96.67439905703392355, -92.77844715994214653, -21.78219314458237932 ) ) ;
#40802=CYLINDRICAL_SURFACE ( 'NONE', #1067, 3.499999999999996003 ) ;
#40810=DIRECTION ( 'NONE',  ( -0.8660254037844382635, -0.5000000000000008882, 1.550000000000000022E-14 ) ) ;
#40825=EDGE_LOOP ( 'NONE', ( #3082, #49952, #26685, #22722 ) ) ;
#40834=CARTESIAN_POINT ( 'NONE',  ( 56.06670390244699576, -67.87844715994098976, 120.2178068554179902 ) ) ;
#40836=DIRECTION ( 'NONE',  ( 0.000000000000000000, 0.000000000000000000, -1.000000000000000000 ) ) ;
#40843=AXIS2_PLACEMENT_3D ( 'NONE', #70319, #377, #43485 ) ;
#40852=DIRECTION ( 'NONE',  ( 1.000000000000000000, 1.000000000000000078E-15, -0.000000000000000000 ) ) ;
#40859=CARTESIAN_POINT ( 'NONE',  ( 121.3178890780284291, -95.01002112898649443, -11.78219314458228695 ) ) ;
#40883=ORIENTED_EDGE ( 'NONE', *, *, #30020, .T. ) ;
#40890=DIRECTION ( 'NONE',  ( -3.100000000000000258E-29, 3.100000000000000044E-14, 1.000000000000000000 ) ) ;
#40899=VERTEX_POINT ( 'NONE', #85224 ) ;
#40910=PLANE ( 'NONE',  #38189 ) ;
#40921=ORIENTED_EDGE ( 'NONE', *, *, #26709, .T. ) ;
#40925=CARTESIAN_POINT ( 'NONE',  ( 127.4153857849114644, -122.7425179094934151, 250.2203867545820231 ) ) ;
#40931=( BOUNDED_CURVE ( )  B_SPLINE_CURVE ( 3, ( #55585, #48782, #7023, #48324 ),
 .UNSPECIFIED., .F., .T. ) 
 B_SPLINE_CURVE_WITH_KNOTS ( ( 4, 4 ),
 ( 0.000000000000000000, 0.4701579599232050821 ),
 .UNSPECIFIED. ) 
 CURVE ( )  GEOMETRIC_REPRESENTATION_ITEM ( )  RATIONAL_B_SPLINE_CURVE ( ( 1.000000000000000000, 0.9816639655796102204, 0.9816639655796102204, 1.000000000000000000 ) ) 
 REPRESENTATION_ITEM ( '' )  );
#40933=LINE ( 'NONE', #13246, #29806 ) ;
#40934=DIRECTION ( 'NONE',  ( 0.000000000000000000, 0.000000000000000000, -1.000000000000000000 ) ) ;
#40938=CARTESIAN_POINT ( 'NONE',  ( 69.56670390244704549, -118.2784471599409812, 51.21780685541800437 ) ) ;
#40950=CARTESIAN_POINT ( 'NONE',  ( 140.3886392338172300, -80.20257156670452048, 248.3919668373590071 ) ) ;
#40962=AXIS2_PLACEMENT_3D ( 'NONE', #73268, #52354, #60991 ) ;
#40984=ORIENTED_EDGE ( 'NONE', *, *, #89792, .F. ) ;
#41011=EDGE_LOOP ( 'NONE', ( #64907, #25471, #62214 ) ) ;
#41033=DIRECTION ( 'NONE',  ( 1.000000000000000000, 8.953411488912556626E-16, 0.000000000000000000 ) ) ;
#41034=CIRCLE ( 'NONE', #49794, 17.00000000000000000 ) ;
#41042=CARTESIAN_POINT ( 'NONE',  ( 114.5988951105837259, -109.2045100507364594, 2.217806855418169576 ) ) ;
#41046=DIRECTION ( 'NONE',  ( -1.000000000000000000, -1.734723475976808672E-15, 0.000000000000000000 ) ) ;
#41047=VERTEX_POINT ( 'NONE', #24316 ) ;
#41057=AXIS2_PLACEMENT_3D ( 'NONE', #60380, #39939, #60830 ) ;
#41062=CYLINDRICAL_SURFACE ( 'NONE', #83430, 27.49999999999999645 ) ;
#41083=LINE ( 'NONE', #82899, #40769 ) ;
#41087=CARTESIAN_POINT ( 'NONE',  ( 67.28117739324572710, -68.08513503999283500, 246.4020950495498994 ) ) ;
#41090=ORIENTED_EDGE ( 'NONE', *, *, #48221, .F. ) ;
#41094=DIRECTION ( 'NONE',  ( 1.000000000000000078E-15, -1.000000000000000000, 0.000000000000000000 ) ) ;
#41109=ADVANCED_FACE ( 'NONE', ( #59697 ), #39707, .T. ) ;
#41113=ORIENTED_EDGE ( 'NONE', *, *, #80777, .T. ) ;
#41129=ORIENTED_EDGE ( 'NONE', *, *, #40112, .T. ) ;
#41140=FACE_BOUND ( 'NONE', #75568, .T. ) ;
#41144=CARTESIAN_POINT ( 'NONE',  ( 121.2221484686747459, -113.6057974291314423, -11.78219314458173272 ) ) ;
#41163=AXIS2_PLACEMENT_3D ( 'NONE', #50202, #9778, #64741 ) ;
#41206=ORIENTED_EDGE ( 'NONE', *, *, #61640, .T. ) ;
#41214=EDGE_LOOP ( 'NONE', ( #53726, #21653 ) ) ;
#41238=CARTESIAN_POINT ( 'NONE',  ( 140.0667039024470455, -118.2784471599408960, 230.7030882296565721 ) ) ;
#41249=VECTOR ( 'NONE', #72448, 1000.000000000000000 ) ;
#41276=CARTESIAN_POINT ( 'NONE',  ( 107.5667039024470171, -94.77844715994206126, -19.78219314458232247 ) ) ;
#41290=CARTESIAN_POINT ( 'NONE',  ( 86.72755763596094880, -122.7870702624433221, 250.2178068554179902 ) ) ;
#41296=DIRECTION ( 'NONE',  ( 0.000000000000000000, 0.000000000000000000, -1.000000000000000000 ) ) ;
#41299=VECTOR ( 'NONE', #18959, 1000.000000000000000 ) ;
#41319=CIRCLE ( 'NONE', #70394, 23.50000000000000711 ) ;
#41322=ORIENTED_EDGE ( 'NONE', *, *, #61454, .F. ) ;
#41346=CYLINDRICAL_SURFACE ( 'NONE', #46919, 3.499999999999996003 ) ;
#41354=LINE ( 'NONE', #20044, #4553 ) ;
#41364=CARTESIAN_POINT ( 'NONE',  ( 67.06670390244701707, -81.17316614790567542, 245.5580738794290028 ) ) ;
#41372=EDGE_CURVE ( 'NONE', #68199, #25814, #49651, .T. ) ;
#41391=CARTESIAN_POINT ( 'NONE',  ( 136.6924846587446609, -119.7509759656530122, 249.3055338466990065 ) ) ;
#41392=ORIENTED_EDGE ( 'NONE', *, *, #29582, .F. ) ;
#41401=EDGE_CURVE ( 'NONE', #41538, #23885, #83756, .T. ) ;
#41402=CARTESIAN_POINT ( 'NONE',  ( 68.36620405317147231, -138.5332053212122787, 246.9855906375420034 ) ) ;
#41406=ORIENTED_EDGE ( 'NONE', *, *, #78726, .T. ) ;
#41408=VECTOR ( 'NONE', #80374, 1000.000000000000000 ) ;
#41428=ORIENTED_EDGE ( 'NONE', *, *, #39152, .F. ) ;
#41462=VERTEX_POINT ( 'NONE', #20476 ) ;
#41463=B_SPLINE_CURVE_WITH_KNOTS ( 'NONE', 3,
 ( #69700, #62867, #28815, #63783, #64228, #83328, #56497, #28342, #7469, #56036, #83784, #84240, #70597, #29261, #56944, #84687, #22903, #22448 ),
 .UNSPECIFIED., .F., .F.,
 ( 4, 2, 2, 2, 2, 2, 2, 2, 4 ),
 ( 0.000000000000000000, 0.1250000000000000000, 0.2500000000000000000, 0.3750000000000000000, 0.5000000000000000000, 0.6250000000000000000, 0.7500000000000000000, 0.8750000000000000000, 1.000000000000000000 ),
 .UNSPECIFIED. ) ;
#41486=DIRECTION ( 'NONE',  ( -1.000000000000000078E-15, 1.000000000000000000, 0.000000000000000000 ) ) ;
#41501=VERTEX_POINT ( 'NONE', #14100 ) ;
#41515=ORIENTED_EDGE ( 'NONE', *, *, #5798, .T. ) ;
#41521=CARTESIAN_POINT ( 'NONE',  ( 137.0667039024470171, -90.27844715994091018, 222.2178068554179902 ) ) ;
#41525=CARTESIAN_POINT ( 'NONE',  ( 68.64392107045537728, -69.36643247059872408, 247.4587235857139831 ) ) ;
#41527=EDGE_LOOP ( 'NONE', ( #55710, #52152, #17159, #20728 ) ) ;
#41537=DIRECTION ( 'NONE',  ( 1.000000000000000078E-15, -1.000000000000000000, 0.000000000000000000 ) ) ;
#41538=VERTEX_POINT ( 'NONE', #26380 ) ;
#41539=ORIENTED_EDGE ( 'NONE', *, *, #58701, .F. ) ;
#41546=ORIENTED_EDGE ( 'NONE', *, *, #38123, .F. ) ;
#41569=ORIENTED_EDGE ( 'NONE', *, *, #40667, .T. ) ;
#41582=CARTESIAN_POINT ( 'NONE',  ( 68.91678303834669350, -69.56165394957326953, 247.5002289977139753 ) ) ;
#41583=DIRECTION ( 'NONE',  ( 1.000000000000000000, 0.000000000000000000, 0.000000000000000000 ) ) ;
#41589=CARTESIAN_POINT ( 'NONE',  ( 98.06670390244704549, -104.2784471599408818, 19.21780685541799016 ) ) ;
#41614=CARTESIAN_POINT ( 'NONE',  ( 145.2442745643976423, -139.1110834320304832, 246.6806061270391126 ) ) ;
#41635=DIRECTION ( 'NONE',  ( 0.000000000000000000, 0.000000000000000000, 1.000000000000000000 ) ) ;
#41656=LINE ( 'NONE', #21701, #85107 ) ;
#41679=DIRECTION ( 'NONE',  ( -0.8660254037844380415, -0.5000000000000012212, 1.550000000000001284E-14 ) ) ;
#41695=CARTESIAN_POINT ( 'NONE',  ( 147.0667039024469886, -67.87844715994090450, 222.2178068554179902 ) ) ;
#41716=ORIENTED_EDGE ( 'NONE', *, *, #63963, .F. ) ;
#41733=DIRECTION ( 'NONE',  ( 0.000000000000000000, 0.000000000000000000, -1.000000000000000000 ) ) ;
#41745=TOROIDAL_SURFACE ( 'NONE', #66392, 29.50000000000000000, 1.500000000000000000 ) ;
#41770=VERTEX_POINT ( 'NONE', #16788 ) ;
#41800=EDGE_CURVE ( 'NONE', #43325, #34061, #84513, .T. ) ;
#41804=ORIENTED_EDGE ( 'NONE', *, *, #74250, .F. ) ;
#41808=CARTESIAN_POINT ( 'NONE',  ( 68.92500634596476061, -138.9257026229574876, 247.5112265945679724 ) ) ;
#41809=CARTESIAN_POINT ( 'NONE',  ( 68.18539514011786196, -127.7157332097851850, 247.4308639981159956 ) ) ;
#41820=AXIS2_PLACEMENT_3D ( 'NONE', #37317, #32270, #53590 ) ;
#41821=CARTESIAN_POINT ( 'NONE',  ( 107.0667039024470313, -104.2784471599420755, -19.78219314458201694 ) ) ;
#41830=DIRECTION ( 'NONE',  ( -3.100000000000000258E-29, 3.100000000000000044E-14, 1.000000000000000000 ) ) ;
#41842=FACE_OUTER_BOUND ( 'NONE', #64310, .T. ) ;
#41855=EDGE_CURVE ( 'NONE', #9196, #88510, #44916, .T. ) ;
#41871=FACE_OUTER_BOUND ( 'NONE', #27481, .T. ) ;
#41875=EDGE_CURVE ( 'NONE', #20346, #12139, #70404, .T. ) ;
#41883=EDGE_CURVE ( 'NONE', #54294, #76096, #72256, .T. ) ;
#41886=DIRECTION ( 'NONE',  ( 1.000000000000000000, 0.000000000000000000, 0.000000000000000000 ) ) ;
#41887=ORIENTED_EDGE ( 'NONE', *, *, #60535, .T. ) ;
#41903=EDGE_CURVE ( 'NONE', #88510, #8874, #3596, .T. ) ;
#41911=CARTESIAN_POINT ( 'NONE',  ( 70.78827404651126187, -139.2284154368976488, 247.4607008287169094 ) ) ;
#41916=EDGE_LOOP ( 'NONE', ( #65258, #33562 ) ) ;
#41921=DIRECTION ( 'NONE',  ( 3.100000000000000258E-29, -3.100000000000000044E-14, -1.000000000000000000 ) ) ;
#41923=DIRECTION ( 'NONE',  ( 0.000000000000000000, 0.000000000000000000, 1.000000000000000000 ) ) ;
#41929=CARTESIAN_POINT ( 'NONE',  ( 96.20012047777625241, -115.5046222945366310, -11.78219314458164924 ) ) ;
#41968=EDGE_CURVE ( 'NONE', #22318, #61315, #33125, .T. ) ;
#41989=EDGE_CURVE ( 'NONE', #78359, #21095, #8500, .T. ) ;
#42007=VECTOR ( 'NONE', #28755, 1000.000000000000000 ) ;
#42009=CIRCLE ( 'NONE', #27494, 15.50000000000000000 ) ;
#42010=ORIENTED_EDGE ( 'NONE', *, *, #3023, .T. ) ;
#42027=EDGE_CURVE ( 'NONE', #58396, #45292, #25865, .T. ) ;
#42031=ADVANCED_FACE ( 'NONE', ( #67435 ), #19746, .T. ) ;
#42061=CARTESIAN_POINT ( 'NONE',  ( 144.0667039024470739, -140.6784471599409017, 245.4568581450700151 ) ) ;
#42064=CARTESIAN_POINT ( 'NONE',  ( 59.56670390244700997, -79.67844715994098692, 120.2178068554179902 ) ) ;
#42066=VERTEX_POINT ( 'NONE', #52869 ) ;
#42079=CARTESIAN_POINT ( 'NONE',  ( 70.06670417066791856, -83.77844715994098124, 55.21780685541800437 ) ) ;
#42090=EDGE_CURVE ( 'NONE', #60002, #56758, #18851, .T. ) ;
#42109=ORIENTED_EDGE ( 'NONE', *, *, #887, .T. ) ;
#42129=ORIENTED_EDGE ( 'NONE', *, *, #46892, .T. ) ;
#42130=LINE ( 'NONE', #20370, #46736 ) ;
#42135=DIRECTION ( 'NONE',  ( 2.195856868753399715E-16, 1.000000000000000000, 0.000000000000000000 ) ) ;
#42146=ORIENTED_EDGE ( 'NONE', *, *, #2224, .F. ) ;
#42150=FACE_OUTER_BOUND ( 'NONE', #66381, .T. ) ;
#42152=DIRECTION ( 'NONE',  ( -0.000000000000000000, -0.000000000000000000, 1.000000000000000000 ) ) ;
#42158=DIRECTION ( 'NONE',  ( -1.000000000000000000, 0.000000000000000000, 0.000000000000000000 ) ) ;
#42166=ORIENTED_EDGE ( 'NONE', *, *, #38492, .F. ) ;
#42174=CARTESIAN_POINT ( 'NONE',  ( 107.0667039024470313, -104.2784471599413934, 2.217806855418003043 ) ) ;
#42178=VERTEX_POINT ( 'NONE', #4333 ) ;
#42185=PLANE ( 'NONE',  #2324 ) ;
#42193=FACE_OUTER_BOUND ( 'NONE', #43171, .T. ) ;
#42205=CARTESIAN_POINT ( 'NONE',  ( 99.08946256649487339, -99.09543445804985140, -19.78219314458218392 ) ) ;
#42222=ORIENTED_EDGE ( 'NONE', *, *, #72995, .F. ) ;
#42228=PLANE ( 'NONE',  #16801 ) ;
#42230=ORIENTED_EDGE ( 'NONE', *, *, #3551, .F. ) ;
#42234=CARTESIAN_POINT ( 'NONE',  ( 106.5667039024470455, -113.7784471599413791, 2.217806855418308132 ) ) ;
#42261=DIRECTION ( 'NONE',  ( 1.000000000000000000, 0.000000000000000000, 0.000000000000000000 ) ) ;
#42263=PLANE ( 'NONE',  #11692 ) ;
#42271=CARTESIAN_POINT ( 'NONE',  ( 117.0667039024470313, -98.59953881414067212, 17.71780685541782319 ) ) ;
#42278=VECTOR ( 'NONE', #67969, 1000.000000000000000 ) ;
#42283=FACE_OUTER_BOUND ( 'NONE', #38110, .T. ) ;
#42315=EDGE_LOOP ( 'NONE', ( #81043, #2669, #10374, #87115, #10773 ) ) ;
#42321=CARTESIAN_POINT ( 'NONE',  ( 122.2189888861420286, -96.57077177933014411, -21.78219314458226918 ) ) ;
#42329=DIRECTION ( 'NONE',  ( 3.100000000000000258E-29, -3.100000000000000044E-14, -1.000000000000000000 ) ) ;
#42343=ORIENTED_EDGE ( 'NONE', *, *, #60901, .T. ) ;
#42356=CARTESIAN_POINT ( 'NONE',  ( 70.37150048485119669, -140.1555257716715630, 246.8822094458865308 ) ) ;
#42376=ADVANCED_FACE ( 'NONE', ( #3332 ), #39342, .F. ) ;
#42377=CARTESIAN_POINT ( 'NONE',  ( 92.87912752678322192, -94.96964819957989334, -19.23816774842029886 ) ) ;
#42389=CYLINDRICAL_SURFACE ( 'NONE', #1546, 8.999999999999994671 ) ;
#42399=ORIENTED_EDGE ( 'NONE', *, *, #12479, .T. ) ;
#42400=CARTESIAN_POINT ( 'NONE',  ( 103.3797721312301547, -105.8297479413482876, -19.78219314458196010 ) ) ;
#42422=CARTESIAN_POINT ( 'NONE',  ( 68.77377604071689632, -69.45229246467815187, 247.4784000562319761 ) ) ;
#42428=EDGE_CURVE ( 'NONE', #71019, #44246, #69442, .T. ) ;
#42435=DIRECTION ( 'NONE',  ( 1.000000000000000000, 1.000000000000000078E-15, 0.000000000000000000 ) ) ;
#42472=ADVANCED_FACE ( 'NONE', ( #31911 ), #86894, .F. ) ;
#42485=CIRCLE ( 'NONE', #3347, 8.999999999999994671 ) ;
#42534=VERTEX_POINT ( 'NONE', #26891 ) ;
#42535=ADVANCED_FACE ( 'NONE', ( #41842 ), #32826, .F. ) ;
#42555=VERTEX_POINT ( 'NONE', #6023 ) ;
#42560=PLANE ( 'NONE',  #30653 ) ;
#42569=ORIENTED_EDGE ( 'NONE', *, *, #40285, .F. ) ;
#42577=CARTESIAN_POINT ( 'NONE',  ( 127.0667052882549797, -71.37844715994091871, 55.21780685541800437 ) ) ;
#42579=ADVANCED_FACE ( 'NONE', ( #48210, #89134 ), #28226, .T. ) ;
#42611=DIRECTION ( 'NONE',  ( 3.100000000000000258E-29, -3.100000000000000044E-14, -1.000000000000000000 ) ) ;
#42613=DIRECTION ( 'NONE',  ( 1.000000000000000000, 0.000000000000000000, 0.000000000000000000 ) ) ;
#42628=LINE ( 'NONE', #41290, #60483 ) ;
#42665=AXIS2_PLACEMENT_3D ( 'NONE', #60144, #73797, #23444 ) ;
#42668=EDGE_LOOP ( 'NONE', ( #35539, #22691, #11416, #45422 ) ) ;
#42675=CARTESIAN_POINT ( 'NONE',  ( 145.5804755031010700, -139.1646755592869056, 245.6810956053649875 ) ) ;
#42678=PLANE ( 'NONE',  #69726 ) ;
#42705=CARTESIAN_POINT ( 'NONE',  ( 68.49250842242263104, -104.4395400694435807, 247.6452922128490002 ) ) ;
#42710=AXIS2_PLACEMENT_3D ( 'NONE', #49859, #77590, #43039 ) ;
#42711=CARTESIAN_POINT ( 'NONE',  ( 68.56670390244700286, -71.37844715994098976, 55.21780685541800437 ) ) ;
#42723=LINE ( 'NONE', #967, #84361 ) ;
#42738=CARTESIAN_POINT ( 'NONE',  ( 116.4407914430478570, -78.35517403977316064, 250.2178068554180470 ) ) ;
#42759=ORIENTED_EDGE ( 'NONE', *, *, #48854, .T. ) ;
#42784=VECTOR ( 'NONE', #39619, 1000.000000000000000 ) ;
#42799=LINE ( 'NONE', #70539, #71540 ) ;
#42805=CARTESIAN_POINT ( 'NONE',  ( 70.60950597247970961, -139.6386892047443951, 247.2886496850582887 ) ) ;
#42815=CIRCLE ( 'NONE', #45724, 17.00000000000000000 ) ;
#42828=CARTESIAN_POINT ( 'NONE',  ( 126.1218394983597335, -124.1980709993372187, 250.2178068554179902 ) ) ;
#42833=FACE_OUTER_BOUND ( 'NONE', #48346, .T. ) ;
#42836=VECTOR ( 'NONE', #18684, 1000.000000000000000 ) ;
#42846=CARTESIAN_POINT ( 'NONE',  ( 63.06670390244699576, -67.87844715994098976, 155.2178068554179902 ) ) ;
#42847=DIRECTION ( 'NONE',  ( 1.000000000000000000, 0.000000000000000000, 0.000000000000000000 ) ) ;
#42867=FACE_OUTER_BOUND ( 'NONE', #12961, .T. ) ;
#42869=CARTESIAN_POINT ( 'NONE',  ( 67.07045655335387835, -67.88107680039439629, 245.6130415843593937 ) ) ;
#42876=CARTESIAN_POINT ( 'NONE',  ( 134.0667039024469602, -40.87844715994091871, 55.21780685541800437 ) ) ;
#42878=CARTESIAN_POINT ( 'NONE',  ( 158.0667039024469886, -67.87844715994090450, 155.2178068554179902 ) ) ;
#42881=CARTESIAN_POINT ( 'NONE',  ( 103.3797721312301547, -105.8297479413476196, 2.217806855418058554 ) ) ;
#42914=ORIENTED_EDGE ( 'NONE', *, *, #25280, .F. ) ;
#42924=AXIS2_PLACEMENT_3D ( 'NONE', #18752, #40535, #46436 ) ;
#42925=CARTESIAN_POINT ( 'NONE',  ( 91.91125933621931665, -109.6038751290247006, -21.02845593540910230 ) ) ;
#42930=DIRECTION ( 'NONE',  ( 1.000000000000000000, 1.000000000000000078E-15, 0.000000000000000000 ) ) ;
#42938=CARTESIAN_POINT ( 'NONE',  ( 145.9273723978340342, -137.0953762339121340, 247.3295516745586440 ) ) ;
#42949=DIRECTION ( 'NONE',  ( 3.100000000000000258E-29, -3.100000000000000044E-14, -1.000000000000000000 ) ) ;
#42950=FACE_OUTER_BOUND ( 'NONE', #13609, .T. ) ;
#42965=ORIENTED_EDGE ( 'NONE', *, *, #71198, .F. ) ;
#43018=ORIENTED_EDGE ( 'NONE', *, *, #23475, .T. ) ;
#43019=CARTESIAN_POINT ( 'NONE',  ( 138.0667039024470171, -104.2784471599409244, 45.21780685541799727 ) ) ;
#43020=ORIENTED_EDGE ( 'NONE', *, *, #40224, .F. ) ;
#43024=DIRECTION ( 'NONE',  ( -1.000000000000000000, -1.000000000000000078E-15, 0.000000000000000000 ) ) ;
#43039=DIRECTION ( 'NONE',  ( -0.1250000000000000278, -0.9921567416492215186, 3.079134169858830699E-14 ) ) ;
#43066=DIRECTION ( 'NONE',  ( -0.7071067811865496822, 0.7071067811865453523, 0.000000000000000000 ) ) ;
#43067=DIRECTION ( 'NONE',  ( 3.100000000000000258E-29, -3.100000000000000044E-14, -1.000000000000000000 ) ) ;
#43080=LINE ( 'NONE', #58069, #22786 ) ;
#43082=CARTESIAN_POINT ( 'NONE',  ( 91.91125933621934507, -107.5284471599419049, -21.78219314458190681 ) ) ;
#43115=AXIS2_PLACEMENT_3D ( 'NONE', #41821, #69558, #508 ) ;
#43131=FACE_BOUND ( 'NONE', #41916, .T. ) ;
#43138=ORIENTED_EDGE ( 'NONE', *, *, #48916, .T. ) ;
#43157=DIRECTION ( 'NONE',  ( 1.000000000000000078E-15, -1.000000000000000000, 0.000000000000000000 ) ) ;
#43171=EDGE_LOOP ( 'NONE', ( #78500, #69738, #39022, #28603 ) ) ;
#43174=PLANE ( 'NONE',  #77735 ) ;
#43184=FACE_OUTER_BOUND ( 'NONE', #51790, .T. ) ;
#43186=CARTESIAN_POINT ( 'NONE',  ( 67.06670390244704549, -104.4389890505713936, 245.7240874041480083 ) ) ;
#43187=ORIENTED_EDGE ( 'NONE', *, *, #46724, .F. ) ;
#43188=AXIS2_PLACEMENT_3D ( 'NONE', #57966, #8950, #37092 ) ;
#43217=LINE ( 'NONE', #27808, #56076 ) ;
#43240=ORIENTED_EDGE ( 'NONE', *, *, #37285, .T. ) ;
#43242=AXIS2_PLACEMENT_3D ( 'NONE', #84431, #390, #42158 ) ;
#43244=VERTEX_POINT ( 'NONE', #650 ) ;
#43252=EDGE_LOOP ( 'NONE', ( #56258, #64818, #53662 ) ) ;
#43255=CYLINDRICAL_SURFACE ( 'NONE', #55079, 17.00000000000000000 ) ;
#43257=CIRCLE ( 'NONE', #5555, 3.000000864267354572 ) ;
#43279=ORIENTED_EDGE ( 'NONE', *, *, #5174, .T. ) ;
#43280=CARTESIAN_POINT ( 'NONE',  ( 116.4407914430480560, -130.2017202801087024, 250.2178068554180470 ) ) ;
#43317=DIRECTION ( 'NONE',  ( 1.000000000000000000, 5.440892098500631367E-15, -1.376676550535195643E-28 ) ) ;
#43325=VERTEX_POINT ( 'NONE', #55140 ) ;
#43330=CARTESIAN_POINT ( 'NONE',  ( 145.3984757889812442, -69.42761852215946305, 247.4725869789474473 ) ) ;
#43338=ORIENTED_EDGE ( 'NONE', *, *, #26709, .F. ) ;
#43383=DIRECTION ( 'NONE',  ( 0.7071067811865470176, 2.262741699796953369E-14, 0.7071067811865480168 ) ) ;
#43387=VECTOR ( 'NONE', #29439, 1000.000000000000000 ) ;
#43404=CARTESIAN_POINT ( 'NONE',  ( 144.0667039024470455, -124.7784471599409102, 55.21780685541800437 ) ) ;
#43413=EDGE_CURVE ( 'NONE', #35731, #11503, #62423, .T. ) ;
#43441=EDGE_LOOP ( 'NONE', ( #62851, #84110, #79582, #76079 ) ) ;
#43485=DIRECTION ( 'NONE',  ( 0.1250000000000000278, 0.9921567416492215186, -3.079134169858830699E-14 ) ) ;
#43487=DIRECTION ( 'NONE',  ( -1.000000000000000078E-15, 1.000000000000000000, 0.000000000000000000 ) ) ;
#43537=DIRECTION ( 'NONE',  ( -3.100000000000000258E-29, 3.100000000000000044E-14, 1.000000000000000000 ) ) ;
#43544=DIRECTION ( 'NONE',  ( 0.000000000000000000, 0.000000000000000000, -1.000000000000000000 ) ) ;
#43578=CARTESIAN_POINT ( 'NONE',  ( 144.5373894638221657, -140.2077779303688203, 245.9389812651000113 ) ) ;
#43584=CIRCLE ( 'NONE', #39244, 30.99999999999998579 ) ;
#43620=EDGE_CURVE ( 'NONE', #57999, #4381, #60982, .T. ) ;
#43634=EDGE_LOOP ( 'NONE', ( #16686, #24942, #61528, #63419 ) ) ;
#43635=DIRECTION ( 'NONE',  ( -0.000000000000000000, -0.000000000000000000, -1.000000000000000000 ) ) ;
#43639=DIRECTION ( 'NONE',  ( 1.000000000000000000, 0.000000000000000000, 0.000000000000000000 ) ) ;
#43673=CARTESIAN_POINT ( 'NONE',  ( 90.52001865076087483, -69.32858309805097008, 247.6470817344352895 ) ) ;
#43675=AXIS2_PLACEMENT_3D ( 'NONE', #86418, #46384, #73204 ) ;
#43686=CARTESIAN_POINT ( 'NONE',  ( 74.06670390244704549, -118.2784471599409812, 45.21780685541799727 ) ) ;
#43695=VERTEX_POINT ( 'NONE', #26023 ) ;
#43709=CARTESIAN_POINT ( 'NONE',  ( 107.0667039024470313, -104.2784471599414502, 0.2178068554180012661 ) ) ;
#43711=CARTESIAN_POINT ( 'NONE',  ( 70.75848861320156402, -139.2980388182697311, 247.4388078084867573 ) ) ;
#43715=ORIENTED_EDGE ( 'NONE', *, *, #13239, .T. ) ;
#43722=CARTESIAN_POINT ( 'NONE',  ( 69.09827022149127629, -138.9035152955028707, 247.0712714749913061 ) ) ;
#43729=DIRECTION ( 'NONE',  ( 1.000000000000000000, 0.000000000000000000, 0.000000000000000000 ) ) ;
#43769=DIRECTION ( 'NONE',  ( -1.000000000000000078E-15, 1.000000000000000000, 0.000000000000000000 ) ) ;
#43771=VECTOR ( 'NONE', #40810, 999.9999999999998863 ) ;
#43791=ORIENTED_EDGE ( 'NONE', *, *, #83989, .T. ) ;
#43802=EDGE_LOOP ( 'NONE', ( #83152, #47830 ) ) ;
#43839=CARTESIAN_POINT ( 'NONE',  ( 146.5623089610532759, -137.3886574699120615, 246.8356538633832997 ) ) ;
#43852=CARTESIAN_POINT ( 'NONE',  ( 144.0664521793745791, -140.6784471599409017, 245.4721420275650132 ) ) ;
#43859=ADVANCED_FACE ( 'NONE', ( #68700 ), #65223, .T. ) ;
#43873=LINE ( 'NONE', #42079, #55811 ) ;
#43879=FACE_OUTER_BOUND ( 'NONE', #53391, .T. ) ;
#43883=ORIENTED_EDGE ( 'NONE', *, *, #58531, .F. ) ;
#43884=LINE ( 'NONE', #70266, #82383 ) ;
#43923=AXIS2_PLACEMENT_3D ( 'NONE', #85050, #50493, #9618 ) ;
#43931=LINE ( 'NONE', #28069, #76843 ) ;
#43942=DIRECTION ( 'NONE',  ( -1.000000000000000078E-15, 1.000000000000000000, 0.000000000000000000 ) ) ;
#43958=ADVANCED_FACE ( 'NONE', ( #24131 ), #51802, .T. ) ;
#43977=VECTOR ( 'NONE', #15626, 1000.000000000000000 ) ;
#43980=ORIENTED_EDGE ( 'NONE', *, *, #18657, .F. ) ;
#43983=VERTEX_POINT ( 'NONE', #65015 ) ;
#44001=CARTESIAN_POINT ( 'NONE',  ( 69.56670390244701707, -90.27844715994098124, 45.21780685541799727 ) ) ;
#44002=LINE ( 'NONE', #77660, #47922 ) ;
#44012=CIRCLE ( 'NONE', #73067, 17.00000000000000000 ) ;
#44019=CARTESIAN_POINT ( 'NONE',  ( 91.91441891875203396, -96.57077177932983147, -11.78219314458225853 ) ) ;
#44035=ADVANCED_FACE ( 'NONE', ( #30937 ), #79554, .T. ) ;
#44043=ORIENTED_EDGE ( 'NONE', *, *, #32048, .F. ) ;
#44050=ORIENTED_EDGE ( 'NONE', *, *, #61588, .T. ) ;
#44063=ORIENTED_EDGE ( 'NONE', *, *, #86425, .T. ) ;
#44069=DIRECTION ( 'NONE',  ( 0.000000000000000000, 0.000000000000000000, 1.000000000000000000 ) ) ;
#44089=VERTEX_POINT ( 'NONE', #12283 ) ;
#44106=DIRECTION ( 'NONE',  ( 1.000000000000000000, 1.000000000000000078E-15, 0.000000000000000000 ) ) ;
#44133=AXIS2_PLACEMENT_3D ( 'NONE', #42064, #55668, #70233 ) ;
#44137=DIRECTION ( 'NONE',  ( 1.000000000000000000, 0.000000000000000000, 0.000000000000000000 ) ) ;
#44138=ADVANCED_FACE ( 'NONE', ( #11385 ), #24570, .F. ) ;
#44151=VECTOR ( 'NONE', #65906, 1000.000000000000000 ) ;
#44153=UNCERTAINTY_MEASURE_WITH_UNIT (LENGTH_MEASURE( 1.000000000000000082E-05 ), #50535, 'distance_accuracy_value', 'NONE');
#44161=CARTESIAN_POINT ( 'NONE',  ( 53.06670390244700286, -78.67844715994100113, 180.4678068554179902 ) ) ;
#44187=LINE ( 'NONE', #71922, #1125 ) ;
#44212=CARTESIAN_POINT ( 'NONE',  ( 146.5379504508059654, -68.38750913315759306, 246.8490270591256035 ) ) ;
#44227=ORIENTED_EDGE ( 'NONE', *, *, #35319, .T. ) ;
#44243=ORIENTED_EDGE ( 'NONE', *, *, #46034, .T. ) ;
#44246=VERTEX_POINT ( 'NONE', #56273 ) ;
#44247=ORIENTED_EDGE ( 'NONE', *, *, #34121, .T. ) ;
#44256=FACE_OUTER_BOUND ( 'NONE', #76971, .T. ) ;
#44257=CARTESIAN_POINT ( 'NONE',  ( 67.06670390244707392, -137.6784471599409869, 55.21780685541800437 ) ) ;
#44267=LINE ( 'NONE', #21625, #88487 ) ;
#44268=CARTESIAN_POINT ( 'NONE',  ( 143.7815414234198101, -140.1960747189870347, 246.8365688484822442 ) ) ;
#44277=CARTESIAN_POINT ( 'NONE',  ( 68.69171528984767860, -139.3034585473416769, 245.6607614303540004 ) ) ;
#44279=ORIENTED_EDGE ( 'NONE', *, *, #40348, .T. ) ;
#44334=EDGE_CURVE ( 'NONE', #74274, #38959, #62661, .T. ) ;
#44336=VERTEX_POINT ( 'NONE', #48114 ) ;
#44347=DIRECTION ( 'NONE',  ( 0.000000000000000000, 0.000000000000000000, -1.000000000000000000 ) ) ;
#44414=ORIENTED_EDGE ( 'NONE', *, *, #25390, .T. ) ;
#44434=CARTESIAN_POINT ( 'NONE',  ( 99.48898161933328765, -117.4034471599418197, -11.78219314458159239 ) ) ;
#44452=DIRECTION ( 'NONE',  ( 1.000000000000000000, 0.000000000000000000, 0.000000000000000000 ) ) ;
#44463=EDGE_CURVE ( 'NONE', #11800, #73928, #29049, .T. ) ;
#44473=ORIENTED_EDGE ( 'NONE', *, *, #51566, .F. ) ;
#44477=ORIENTED_EDGE ( 'NONE', *, *, #28661, .F. ) ;
#44481=LINE ( 'NONE', #37692, #39673 ) ;
#44484=AXIS2_PLACEMENT_3D ( 'NONE', #51153, #30281, #70730 ) ;
#44494=ORIENTED_EDGE ( 'NONE', *, *, #28687, .F. ) ;
#44553=AXIS2_PLACEMENT_3D ( 'NONE', #14000, #48939, #47604 ) ;
#44556=DIRECTION ( 'NONE',  ( -0.3535533905932746190, 0.6123724356958156756, 0.7071067811865288100 ) ) ;
#44563=ORIENTED_EDGE ( 'NONE', *, *, #88478, .T. ) ;
#44570=LINE ( 'NONE', #39104, #84002 ) ;
#44571=B_SPLINE_CURVE_WITH_KNOTS ( 'NONE', 3,
 ( #63271, #50074, #83724, #77809, #63725, #41911, #49173, #43711, #57337, #56440, #15127, #1507, #62811, #588, #8772, #64179, #71449, #36474, #42805, #55981, #8315, #1951, #21503, #14687, #84185, #36014, #42356, #21959, #56894, #7856, #29645, #9214, #62366, #149, #21045 ),
 .UNSPECIFIED., .F., .F.,
 ( 4, 2, 2, 1, 1, 1, 2, 2, 2, 1, 1, 2, 2, 2, 2, 1, 1, 2, 2, 2, 4 ),
 ( 0.000000000000000000, 0.06250000000034182379, 0.09375000000052836902, 0.1093750000006312451, 0.1171875000006843554, 0.1210937500007093492, 0.1230468750007258083, 0.1250000000007422951, 0.1875000000008925083, 0.2187500000009702517, 0.2343750000009904300, 0.2421875000010005330, 0.2500000000010105805, 0.3750000000010189627, 0.4375000000010146883, 0.4687500000010152434, 0.4843750000010160761, 0.4921875000010164647, 0.5000000000010168533, 0.7500000000005084821, 1.000000000000000000 ),
 .UNSPECIFIED. ) ;
#44582=VECTOR ( 'NONE', #84433, 1000.000000000000000 ) ;
#44583=EDGE_LOOP ( 'NONE', ( #45347, #34648, #52629, #3439, #71704, #82561, #24884, #78562, #48158, #85762 ) ) ;
#44608=CARTESIAN_POINT ( 'NONE',  ( 68.75114609266175592, -139.2473167355539374, 246.2273013858858803 ) ) ;
#44614=CARTESIAN_POINT ( 'NONE',  ( 147.0667039024469886, -67.87844715994090450, 247.2178068554179902 ) ) ;
#44621=VECTOR ( 'NONE', #26905, 1000.000000000000000 ) ;
#44628=EDGE_CURVE ( 'NONE', #54402, #24467, #27671, .T. ) ;
#44640=CARTESIAN_POINT ( 'NONE',  ( 108.0345654683053453, -121.2196520243554403, -19.23816181211449106 ) ) ;
#44641=EDGE_CURVE ( 'NONE', #48031, #26236, #73045, .T. ) ;
#44667=CARTESIAN_POINT ( 'NONE',  ( 146.4037250783899822, -68.51735678003049657, 246.9840931576174796 ) ) ;
#44678=ORIENTED_EDGE ( 'NONE', *, *, #22576, .F. ) ;
#44684=CARTESIAN_POINT ( 'NONE',  ( 120.2221484686747317, -111.8737466215625602, -11.78219314458178779 ) ) ;
#44688=DIRECTION ( 'NONE',  ( 1.000000000000000078E-15, -1.000000000000000000, 0.000000000000000000 ) ) ;
#44690=EDGE_CURVE ( 'NONE', #46794, #50049, #17650, .T. ) ;
#44693=CARTESIAN_POINT ( 'NONE',  ( 147.0667039024470171, -79.67844715994090166, 55.21780685541800437 ) ) ;
#44698=VERTEX_POINT ( 'NONE', #88490 ) ;
#44705=DIRECTION ( 'NONE',  ( 1.000000000000000078E-15, -1.000000000000000000, 0.000000000000000000 ) ) ;
#44706=CARTESIAN_POINT ( 'NONE',  ( 72.18555876632754575, -117.2313175559279728, 248.3919653347779786 ) ) ;
#44717=CARTESIAN_POINT ( 'NONE',  ( 143.3136118988180954, -139.1558145886066882, 247.4862956150515743 ) ) ;
#44724=CARTESIAN_POINT ( 'NONE',  ( 67.55791682848843038, -137.3945666130911150, 246.8203320373089582 ) ) ;
#44739=FACE_OUTER_BOUND ( 'NONE', #12529, .T. ) ;
#44759=CARTESIAN_POINT ( 'NONE',  ( 107.0667039024470313, -104.2784471599413934, 2.217806855418003043 ) ) ;
#44774=DIRECTION ( 'NONE',  ( 3.100000000000000258E-29, -3.100000000000000044E-14, -1.000000000000000000 ) ) ;
#44778=ADVANCED_FACE ( 'NONE', ( #18080, #58958 ), #29726, .F. ) ;
#44808=ORIENTED_EDGE ( 'NONE', *, *, #29907, .F. ) ;
#44819=CARTESIAN_POINT ( 'NONE',  ( 147.0667039024457665, -137.6758868153238780, 245.5072646551060132 ) ) ;
#44820=CARTESIAN_POINT ( 'NONE',  ( 91.91125933621933086, -96.64603743111524636, -19.23816181211526910 ) ) ;
#44851=EDGE_LOOP ( 'NONE', ( #655, #30178, #11548, #42010 ) ) ;
#44856=EDGE_CURVE ( 'NONE', #17803, #61315, #76075, .T. ) ;
#44857=ORIENTED_EDGE ( 'NONE', *, *, #10429, .F. ) ;
#44860=FACE_OUTER_BOUND ( 'NONE', #18104, .T. ) ;
#44872=ORIENTED_EDGE ( 'NONE', *, *, #4901, .T. ) ;
#44879=VECTOR ( 'NONE', #53715, 1000.000000000000114 ) ;
#44902=CARTESIAN_POINT ( 'NONE',  ( 74.68178297942419874, -67.87877198938119250, 246.0920795366729976 ) ) ;
#44916=LINE ( 'NONE', #58982, #6997 ) ;
#44927=DIRECTION ( 'NONE',  ( -0.8944271909999158554, 1.296919426949877873E-14, 0.4472135954999579277 ) ) ;
#44950=CARTESIAN_POINT ( 'NONE',  ( 99.48898161933324502, -91.15344715994181968, -11.78219314458242550 ) ) ;
#44951=DIRECTION ( 'NONE',  ( -0.4999999999999985567, -0.8660254037844395958, 2.688821387764040899E-14 ) ) ;
#44958=EDGE_LOOP ( 'NONE', ( #55249, #15539, #33074, #53541 ) ) ;
#44975=CARTESIAN_POINT ( 'NONE',  ( 115.0439452383992318, -109.4614598618335890, 2.217806855418169576 ) ) ;
#44983=ORIENTED_EDGE ( 'NONE', *, *, #53746, .F. ) ;
#44984=PLANE ( 'NONE',  #18230 ) ;
#45001=FACE_OUTER_BOUND ( 'NONE', #25634, .T. ) ;
#45002=DIRECTION ( 'NONE',  ( -0.7759704746411383303, 0.6307692307692303046, 0.000000000000000000 ) ) ;
#45019=CARTESIAN_POINT ( 'NONE',  ( 154.5667039024470171, -79.67844715994088745, 190.2178068554179902 ) ) ;
#45039=VECTOR ( 'NONE', #39302, 1000.000000000000000 ) ;
#45057=B_SPLINE_CURVE_WITH_KNOTS ( 'NONE', 3,
 ( #45949, #53205, #5559, #81862 ),
 .UNSPECIFIED., .F., .F.,
 ( 4, 4 ),
 ( -0.2154603786882610117, -0.01977385131020209519 ),
 .UNSPECIFIED. ) ;
#45062=ADVANCED_FACE ( 'NONE', ( #51919 ), #38311, .T. ) ;
#45094=VECTOR ( 'NONE', #53607, 1000.000000000000000 ) ;
#45101=CARTESIAN_POINT ( 'NONE',  ( 98.58946256649487339, -99.96145986183361742, 2.217806855417864043 ) ) ;
#45108=CARTESIAN_POINT ( 'NONE',  ( 80.76543358272510886, -80.39462547777496582, 249.3134381260879877 ) ) ;
#45122=DIRECTION ( 'NONE',  ( 1.000000000000000078E-15, -1.000000000000000000, 0.000000000000000000 ) ) ;
#45158=CARTESIAN_POINT ( 'NONE',  ( 143.8697414714609124, -140.3737278804164532, 246.5975155025261074 ) ) ;
#45165=CARTESIAN_POINT ( 'NONE',  ( 68.61434409300457560, -136.9218521013149541, 247.4649940182199828 ) ) ;
#45167=ADVANCED_FACE ( 'NONE', ( #67350 ), #4697, .T. ) ;
#45217=AXIS2_PLACEMENT_3D ( 'NONE', #38480, #17609, #65311 ) ;
#45221=CARTESIAN_POINT ( 'NONE',  ( 107.5667039024470171, -94.77844715994206126, -19.78219314458232247 ) ) ;
#45254=ORIENTED_EDGE ( 'NONE', *, *, #22463, .T. ) ;
#45269=LINE ( 'NONE', #4848, #38334 ) ;
#45274=ORIENTED_EDGE ( 'NONE', *, *, #61588, .F. ) ;
#45292=VERTEX_POINT ( 'NONE', #64617 ) ;
#45293=EDGE_LOOP ( 'NONE', ( #11909, #89760, #70655, #78256, #43138, #14161 ) ) ;
#45337=CARTESIAN_POINT ( 'NONE',  ( 143.2608543353592836, -67.87860957466101297, 246.0727973265990158 ) ) ;
#45347=ORIENTED_EDGE ( 'NONE', *, *, #87739, .F. ) ;
#45355=CARTESIAN_POINT ( 'NONE',  ( 143.2570438357147964, -67.87844715994090450, 245.5376130947089734 ) ) ;
#45361=DIRECTION ( 'NONE',  ( 1.000000000000000078E-15, -1.000000000000000000, 0.000000000000000000 ) ) ;
#45363=ADVANCED_FACE ( 'NONE', ( #50980 ), #8319, .F. ) ;
#45369=CARTESIAN_POINT ( 'NONE',  ( 99.48898161933328765, -117.4034471599418197, -11.78219314458159239 ) ) ;
#45378=ORIENTED_EDGE ( 'NONE', *, *, #27404, .F. ) ;
#45386=CARTESIAN_POINT ( 'NONE',  ( 91.91125933621943034, -104.2784471599418339, -11.78219314458200984 ) ) ;
#45395=AXIS2_PLACEMENT_3D ( 'NONE', #76260, #48977, #1309 ) ;
#45400=EDGE_LOOP ( 'NONE', ( #72328, #30265 ) ) ;
#45413=ORIENTED_EDGE ( 'NONE', *, *, #26843, .T. ) ;
#45420=DIRECTION ( 'NONE',  ( -3.100000000000000258E-29, 3.100000000000000044E-14, 1.000000000000000000 ) ) ;
#45422=ORIENTED_EDGE ( 'NONE', *, *, #85700, .F. ) ;
#45424=VECTOR ( 'NONE', #28424, 1000.000000000000000 ) ;
#45437=VERTEX_POINT ( 'NONE', #52731 ) ;
#45441=FACE_OUTER_BOUND ( 'NONE', #11387, .T. ) ;
#45453=ADVANCED_FACE ( 'NONE', ( #39142 ), #51854, .F. ) ;
#45456=CARTESIAN_POINT ( 'NONE',  ( 125.5177273812784762, -131.0330679306342461, 55.21780685541800437 ) ) ;
#45466=LINE ( 'NONE', #86837, #85131 ) ;
#45468=ORIENTED_EDGE ( 'NONE', *, *, #51478, .F. ) ;
#45495=CARTESIAN_POINT ( 'NONE',  ( 145.9875769262907284, -101.1106333528077954, 247.5368628348080051 ) ) ;
#45499=CARTESIAN_POINT ( 'NONE',  ( 63.06670390244700997, -79.67844715994098692, 85.21780685541799016 ) ) ;
#45531=CARTESIAN_POINT ( 'NONE',  ( 107.0667039024470739, -133.7784471599409528, 24.21780685541800082 ) ) ;
#45547=VERTEX_POINT ( 'NONE', #67289 ) ;
#45569=CARTESIAN_POINT ( 'NONE',  ( 107.0667039024470029, -74.77844715994095282, 24.21780685541800082 ) ) ;
#45581=ORIENTED_EDGE ( 'NONE', *, *, #63341, .T. ) ;
#45597=CARTESIAN_POINT ( 'NONE',  ( 67.37732175900356424, -137.4831949855723110, 246.5806332000785233 ) ) ;
#45608=CYLINDRICAL_SURFACE ( 'NONE', #81207, 17.00000000000000000 ) ;
#45612=CARTESIAN_POINT ( 'NONE',  ( 107.0667039024470313, -104.2784471599418197, -11.78219314458200984 ) ) ;
#45613=VECTOR ( 'NONE', #58813, 1000.000000000000000 ) ;
#45648=VERTEX_POINT ( 'NONE', #47735 ) ;
#45661=EDGE_LOOP ( 'NONE', ( #86697, #78894, #64649, #73494 ) ) ;
#45679=CARTESIAN_POINT ( 'NONE',  ( 90.06670390244703128, -104.2784471599417770, -9.937637710810031777 ) ) ;
#45683=EDGE_CURVE ( 'NONE', #31932, #35863, #49074, .T. ) ;
#45687=VERTEX_POINT ( 'NONE', #14591 ) ;
#45689=LINE ( 'NONE', #24834, #5356 ) ;
#45691=AXIS2_PLACEMENT_3D ( 'NONE', #2337, #58611, #64558 ) ;
#45701=DIRECTION ( 'NONE',  ( -0.4999999999999931166, -0.8660254037844425934, 2.684678751731770391E-14 ) ) ;
#45720=CIRCLE ( 'NONE', #55833, 7.999999999999992895 ) ;
#45724=AXIS2_PLACEMENT_3D ( 'NONE', #25184, #81074, #39700 ) ;
#45732=CARTESIAN_POINT ( 'NONE',  ( 129.9732689015971516, -140.6782641201739352, 246.0176313805619941 ) ) ;
#45734=CARTESIAN_POINT ( 'NONE',  ( 69.89223516763907185, -140.0675090405642891, 246.8991749143359868 ) ) ;
#45751=EDGE_CURVE ( 'NONE', #14487, #70410, #21985, .T. ) ;
#45768=DIRECTION ( 'NONE',  ( 0.000000000000000000, 0.000000000000000000, 1.000000000000000000 ) ) ;
#45769=CARTESIAN_POINT ( 'NONE',  ( 82.56670390244703128, -104.2784471599409670, 23.21780685541800082 ) ) ;
#45770=EDGE_CURVE ( 'NONE', #20355, #56758, #24882, .T. ) ;
#45780=CARTESIAN_POINT ( 'NONE',  ( 112.7890892452997917, -68.16618858916433510, 247.0964967658709952 ) ) ;
#45781=VECTOR ( 'NONE', #61289, 1000.000000000000114 ) ;
#45791=EDGE_CURVE ( 'NONE', #78823, #82481, #7767, .T. ) ;
#45809=CARTESIAN_POINT ( 'NONE',  ( 92.91125933621933086, -94.95109689075221127, -11.78219314458228695 ) ) ;
#45827=CIRCLE ( 'NONE', #26991, 15.50000000000000000 ) ;
#45831=EDGE_LOOP ( 'NONE', ( #37266, #74391, #58749 ) ) ;
#45839=B_SPLINE_SURFACE_WITH_KNOTS ( 'NONE', 3, 3, ( 
 ( #88671, #54101, #12815, #87761, #47298 ),
 ( #75023, #40500, #67300, #68218, #11459 ),
 ( #25981, #53195, #80966, #59141, #81422 ),
 ( #53650, #46397, #45495, #18714, #73219 ),
 ( #39594, #10998, #38699, #59580, #25078 ) ),
 .UNSPECIFIED., .F., .F., .F.,
 ( 4, 1, 4 ),
 ( 4, 1, 4 ),
 ( 0.000000000000000000, 0.5714285714285709528, 1.000000000000000000 ),
 ( 0.1438910682813590025, 4.132355267033809731, 7.123703416098150498 ),
 .UNSPECIFIED. ) ;
#45840=CARTESIAN_POINT ( 'NONE',  ( 144.0667039024470171, -102.7784471599409102, 55.21780685541800437 ) ) ;
#45841=LINE ( 'NONE', #79069, #39628 ) ;
#45864=EDGE_LOOP ( 'NONE', ( #79872, #47632, #73293, #84044 ) ) ;
#45914=CARTESIAN_POINT ( 'NONE',  ( 107.5667039024470313, -100.3098201933444926, 2.217806855417892020 ) ) ;
#45929=CARTESIAN_POINT ( 'NONE',  ( 59.56670390244699576, -67.87844715994098976, 120.2178068554179902 ) ) ;
#45949=CARTESIAN_POINT ( 'NONE',  ( 144.0667039004811443, -140.6784471619068029, 245.4415720117440003 ) ) ;
#45950=CIRCLE ( 'NONE', #21292, 11.49999999999999645 ) ;
#45981=DIRECTION ( 'NONE',  ( -1.000000000000000078E-15, 1.000000000000000000, 0.000000000000000000 ) ) ;
#45992=DIRECTION ( 'NONE',  ( 1.000000000000000000, 1.000000000000000078E-15, 0.000000000000000000 ) ) ;
#45993=CARTESIAN_POINT ( 'NONE',  ( 146.5596880459861779, -68.36644973479313592, 246.8246830390798721 ) ) ;
#46000=DIRECTION ( 'NONE',  ( -1.000000000000000000, -1.000000000000000078E-15, 0.000000000000000000 ) ) ;
#46001=ORIENTED_EDGE ( 'NONE', *, *, #16404, .F. ) ;
#46004=LINE ( 'NONE', #47802, #35541 ) ;
#46010=EDGE_CURVE ( 'NONE', #638, #13040, #68458, .T. ) ;
#46012=LINE ( 'NONE', #19237, #21287 ) ;
#46020=ORIENTED_EDGE ( 'NONE', *, *, #44856, .T. ) ;
#46034=EDGE_CURVE ( 'NONE', #66921, #39084, #72684, .T. ) ;
#46047=DIRECTION ( 'NONE',  ( 3.100000000000000258E-29, -3.100000000000000044E-14, -1.000000000000000000 ) ) ;
#46050=FACE_OUTER_BOUND ( 'NONE', #16617, .T. ) ;
#46053=ORIENTED_EDGE ( 'NONE', *, *, #47530, .T. ) ;
#46060=LINE ( 'NONE', #31111, #84116 ) ;
#46071=CARTESIAN_POINT ( 'NONE',  ( 145.4416927396864878, -139.3034583227001804, 245.6607614918409865 ) ) ;
#46075=ADVANCED_FACE ( 'NONE', ( #19949 ), #27652, .T. ) ;
#46085=CIRCLE ( 'NONE', #12728, 2.000000000000001776 ) ;
#46149=FACE_OUTER_BOUND ( 'NONE', #3464, .T. ) ;
#46152=DIRECTION ( 'NONE',  ( 1.000000000000000078E-15, -1.000000000000000000, 0.000000000000000000 ) ) ;
#46153=DIRECTION ( 'NONE',  ( -0.8660254037844425934, 0.4999999999999931166, -1.549999999999981405E-14 ) ) ;
#46164=CIRCLE ( 'NONE', #7034, 7.999999999999992895 ) ;
#46178=ORIENTED_EDGE ( 'NONE', *, *, #46010, .F. ) ;
#46204=ORIENTED_EDGE ( 'NONE', *, *, #69069, .T. ) ;
#46226=AXIS2_PLACEMENT_3D ( 'NONE', #29895, #42152, #30340 ) ;
#46232=EDGE_LOOP ( 'NONE', ( #11422, #67315, #60993, #44872 ) ) ;
#46236=EDGE_CURVE ( 'NONE', #69797, #48853, #65529, .T. ) ;
#46241=CARTESIAN_POINT ( 'NONE',  ( 124.0667039024470313, -104.2784471599417486, -9.937637710810031777 ) ) ;
#46281=ORIENTED_EDGE ( 'NONE', *, *, #51344, .T. ) ;
#46309=CARTESIAN_POINT ( 'NONE',  ( 69.94830149775677341, -138.0565978109353864, 247.6574394596379989 ) ) ;
#46313=PLANE ( 'NONE',  #86389 ) ;
#46317=AXIS2_PLACEMENT_3D ( 'NONE', #104, #6466, #35055 ) ;
#46332=VECTOR ( 'NONE', #61165, 999.9999999999998863 ) ;
#46340=ORIENTED_EDGE ( 'NONE', *, *, #86717, .T. ) ;
#46342=CARTESIAN_POINT ( 'NONE',  ( 107.0667039024470313, -104.2784471599409528, 25.71780685541800437 ) ) ;
#46348=CARTESIAN_POINT ( 'NONE',  ( 122.2221484686747459, -108.0760968907521828, -11.78219314458189793 ) ) ;
#46360=EDGE_CURVE ( 'NONE', #33131, #75751, #21290, .T. ) ;
#46366=LINE ( 'NONE', #74101, #5459 ) ;
#46370=CARTESIAN_POINT ( 'NONE',  ( 72.90080881784491851, -85.71128516271417652, 248.3919653347779786 ) ) ;
#46382=AXIS2_PLACEMENT_3D ( 'NONE', #54024, #87250, #31372 ) ;
#46384=DIRECTION ( 'NONE',  ( 3.100000000000000258E-29, -3.100000000000000044E-14, -1.000000000000000000 ) ) ;
#46385=EDGE_LOOP ( 'NONE', ( #82828, #6068, #50237 ) ) ;
#46388=ADVANCED_FACE ( 'NONE', ( #10345 ), #73451, .F. ) ;
#46397=CARTESIAN_POINT ( 'NONE',  ( 145.8343148362385477, -124.3925565579663015, 247.4656831979029903 ) ) ;
#46412=CARTESIAN_POINT ( 'NONE',  ( 106.0667039024470171, -87.35579742913164125, -19.26696060647653397 ) ) ;
#46434=VECTOR ( 'NONE', #27520, 1000.000000000000114 ) ;
#46436=DIRECTION ( 'NONE',  ( -1.000000000000000000, 0.000000000000000000, 0.000000000000000000 ) ) ;
#46447=B_SPLINE_CURVE_WITH_KNOTS ( 'NONE', 3,
 ( #52643, #4081, #80854, #80401 ),
 .UNSPECIFIED., .F., .F.,
 ( 4, 4 ),
 ( -0.3974825557268100162, -0.3842043193313789962 ),
 .UNSPECIFIED. ) ;
#46448=ADVANCED_FACE ( 'NONE', ( #79404 ), #10772, .T. ) ;
#46466=EDGE_CURVE ( 'NONE', #84388, #73518, #66182, .T. ) ;
#46470=VERTEX_POINT ( 'NONE', #38931 ) ;
#46519=CARTESIAN_POINT ( 'NONE',  ( 59.56670390244699576, -67.87844715994098976, 190.2178068554179902 ) ) ;
#46528=CARTESIAN_POINT ( 'NONE',  ( 145.3595637443018234, -69.45303146431501773, 247.4784022495120155 ) ) ;
#46553=CIRCLE ( 'NONE', #65444, 4.500000000000003553 ) ;
#46560=EDGE_CURVE ( 'NONE', #18229, #40899, #88626, .T. ) ;
#46561=CARTESIAN_POINT ( 'NONE',  ( 110.7536356736639078, -102.7271463785358492, -19.78219314458207378 ) ) ;
#46566=ORIENTED_EDGE ( 'NONE', *, *, #54600, .F. ) ;
#46587=LINE ( 'NONE', #83713, #50374 ) ;
#46595=ORIENTED_EDGE ( 'NONE', *, *, #51843, .F. ) ;
#46596=CARTESIAN_POINT ( 'NONE',  ( 59.56670390244699576, -67.87844715994098976, 155.2178068554179902 ) ) ;
#46598=CIRCLE ( 'NONE', #32086, 3.499999999999996003 ) ;
#46601=CARTESIAN_POINT ( 'NONE',  ( 83.56670390244703128, -104.2784471599409670, 24.21780685541800082 ) ) ;
#46614=CARTESIAN_POINT ( 'NONE',  ( 91.91125933621933086, -96.68314769832107913, -11.78219314458223188 ) ) ;
#46627=DIRECTION ( 'NONE',  ( -1.000000000000000000, -8.538276166416950255E-16, -4.531343884107452465E-30 ) ) ;
#46633=CIRCLE ( 'NONE', #69876, 4.500000000000003553 ) ;
#46638=DIRECTION ( 'NONE',  ( 0.000000000000000000, 0.000000000000000000, -1.000000000000000000 ) ) ;
#46639=CARTESIAN_POINT ( 'NONE',  ( 145.3524573197677228, -139.2182000785689411, 246.3670265245609983 ) ) ;
#46645=ORIENTED_EDGE ( 'NONE', *, *, #64316, .F. ) ;
#46651=EDGE_CURVE ( 'NONE', #5243, #54294, #77214, .T. ) ;
#46655=CARTESIAN_POINT ( 'NONE',  ( 122.2221484686747317, -96.68314769832130651, -19.26696060647622843 ) ) ;
#46658=DIRECTION ( 'NONE',  ( -3.100000000000000258E-29, 3.100000000000000044E-14, 1.000000000000000000 ) ) ;
#46672=DIRECTION ( 'NONE',  ( 0.000000000000000000, 0.000000000000000000, 1.000000000000000000 ) ) ;
#46678=CIRCLE ( 'NONE', #64153, 30.99999999999998579 ) ;
#46682=DIRECTION ( 'NONE',  ( 1.000000000000000078E-15, -1.000000000000000000, 0.000000000000000000 ) ) ;
#46692=LINE ( 'NONE', #12197, #55685 ) ;
#46708=CYLINDRICAL_SURFACE ( 'NONE', #57109, 3.500000000000003109 ) ;
#46724=EDGE_CURVE ( 'NONE', #1745, #701, #52323, .T. ) ;
#46728=CARTESIAN_POINT ( 'NONE',  ( 98.58946256649487339, -99.96145986183361742, 2.217806855417864043 ) ) ;
#46736=VECTOR ( 'NONE', #76217, 1000.000000000000000 ) ;
#46742=DIRECTION ( 'NONE',  ( 0.8660254037844380415, 0.5000000000000012212, -1.550000000000001284E-14 ) ) ;
#46745=DIRECTION ( 'NONE',  ( 0.4999999999999989453, 0.8660254037844392627, -2.684678751731760294E-14 ) ) ;
#46750=( BOUNDED_CURVE ( )  B_SPLINE_CURVE ( 3, ( #2572, #51141, #85697, #71614 ),
 .UNSPECIFIED., .F., .F. ) 
 B_SPLINE_CURVE_WITH_KNOTS ( ( 4, 4 ),
 ( 2.669330456947324848, 2.679444341124444851 ),
 .UNSPECIFIED. ) 
 CURVE ( )  GEOMETRIC_REPRESENTATION_ITEM ( )  RATIONAL_B_SPLINE_CURVE ( ( 1.000000000000000000, 0.9999914757970698176, 0.9999914757970698176, 1.000000000000000000 ) ) 
 REPRESENTATION_ITEM ( '' )  );
#46773=DIRECTION ( 'NONE',  ( 0.000000000000000000, 0.000000000000000000, -1.000000000000000000 ) ) ;
#46780=EDGE_CURVE ( 'NONE', #37337, #47465, #75291, .T. ) ;
#46785=DIRECTION ( 'NONE',  ( -0.8660254037844379305, -0.5000000000000012212, 1.550000000000001284E-14 ) ) ;
#46794=VERTEX_POINT ( 'NONE', #49323 ) ;
#46798=CARTESIAN_POINT ( 'NONE',  ( 162.0667039024470171, -77.67844715994088745, 55.21780685541800437 ) ) ;
#46802=DIRECTION ( 'NONE',  ( -1.000000000000000078E-15, 1.000000000000000000, 0.000000000000000000 ) ) ;
#46803=ORIENTED_EDGE ( 'NONE', *, *, #46994, .T. ) ;
#46806=ORIENTED_EDGE ( 'NONE', *, *, #38123, .T. ) ;
#46809=ORIENTED_EDGE ( 'NONE', *, *, #41372, .F. ) ;
#46816=CARTESIAN_POINT ( 'NONE',  ( 68.77555146766027860, -139.1540193827811152, 247.4783998280180128 ) ) ;
#46827=EDGE_CURVE ( 'NONE', #88034, #9965, #77054, .T. ) ;
#46828=CARTESIAN_POINT ( 'NONE',  ( 128.9945611041196685, -130.4030827564308197, 249.3173333679100097 ) ) ;
#46829=DIRECTION ( 'NONE',  ( 0.000000000000000000, 0.000000000000000000, 1.000000000000000000 ) ) ;
#46859=DIRECTION ( 'NONE',  ( 0.7349399772593249169, 0.6687953793059874252, 0.1121426343770439288 ) ) ;
#46865=ORIENTED_EDGE ( 'NONE', *, *, #52378, .T. ) ;
#46877=DIRECTION ( 'NONE',  ( 0.000000000000000000, 0.000000000000000000, -1.000000000000000000 ) ) ;
#46886=EDGE_CURVE ( 'NONE', #32183, #13040, #36159, .T. ) ;
#46892=EDGE_CURVE ( 'NONE', #20155, #18276, #8004, .T. ) ;
#46900=ORIENTED_EDGE ( 'NONE', *, *, #27108, .F. ) ;
#46909=ORIENTED_EDGE ( 'NONE', *, *, #21390, .F. ) ;
#46919=AXIS2_PLACEMENT_3D ( 'NONE', #82281, #33659, #74544 ) ;
#46925=ADVANCED_FACE ( 'NONE', ( #44739 ), #17058, .T. ) ;
#46945=FACE_OUTER_BOUND ( 'NONE', #35606, .T. ) ;
#46975=ORIENTED_EDGE ( 'NONE', *, *, #21162, .F. ) ;
#46990=DIRECTION ( 'NONE',  ( 0.000000000000000000, 0.000000000000000000, 1.000000000000000000 ) ) ;
#46992=ORIENTED_EDGE ( 'NONE', *, *, #28129, .F. ) ;
#46993=EDGE_LOOP ( 'NONE', ( #44414, #84453, #22509, #5639 ) ) ;
#46994=EDGE_CURVE ( 'NONE', #85940, #37406, #17935, .T. ) ;
#47002=AXIS2_PLACEMENT_3D ( 'NONE', #79132, #16898, #38995 ) ;
#47007=EDGE_LOOP ( 'NONE', ( #89504, #38922, #61240, #52605 ) ) ;
#47010=CARTESIAN_POINT ( 'NONE',  ( 144.1763536145585647, -138.0482283979624185, 247.6588381036639817 ) ) ;
#47013=CARTESIAN_POINT ( 'NONE',  ( 151.0667039024469886, -67.87844715994090450, 120.2178068554179902 ) ) ;
#47029=DIRECTION ( 'NONE',  ( -1.000000000000000000, -1.000000000000000078E-15, 0.000000000000000000 ) ) ;
#47045=AXIS2_PLACEMENT_3D ( 'NONE', #82634, #34447, #68085 ) ;
#47074=AXIS2_PLACEMENT_3D ( 'NONE', #29928, #57614, #85356 ) ;
#47076=ORIENTED_EDGE ( 'NONE', *, *, #4901, .F. ) ;
#47095=CARTESIAN_POINT ( 'NONE',  ( 90.06670420047025516, -131.9777253117771636, 55.21780685541800437 ) ) ;
#47129=VECTOR ( 'NONE', #9807, 1000.000000000000000 ) ;
#47149=DIRECTION ( 'NONE',  ( -1.087812297297669405E-15, 1.000000000000000000, -3.100000000000000044E-14 ) ) ;
#47153=DIRECTION ( 'NONE',  ( 0.000000000000000000, 0.000000000000000000, 1.000000000000000000 ) ) ;
#47195=VECTOR ( 'NONE', #4675, 999.9999999999998863 ) ;
#47208=EDGE_CURVE ( 'NONE', #85102, #69134, #25369, .T. ) ;
#47232=DIRECTION ( 'NONE',  ( -0.06842228117015292099, 0.06842228117823027922, 0.9953073811028629869 ) ) ;
#47255=ORIENTED_EDGE ( 'NONE', *, *, #73590, .F. ) ;
#47258=EDGE_CURVE ( 'NONE', #17863, #27883, #46692, .T. ) ;
#47260=ORIENTED_EDGE ( 'NONE', *, *, #63963, .T. ) ;
#47270=ADVANCED_FACE ( 'NONE', ( #67603 ), #30521, .F. ) ;
#47272=DIRECTION ( 'NONE',  ( -1.000000000000000078E-15, 1.000000000000000000, -3.100000000000000044E-14 ) ) ;
#47276=ORIENTED_EDGE ( 'NONE', *, *, #8, .F. ) ;
#47286=ORIENTED_EDGE ( 'NONE', *, *, #83858, .T. ) ;
#47287=ADVANCED_FACE ( 'NONE', ( #81702 ), #88513, .F. ) ;
#47291=CIRCLE ( 'NONE', #64760, 4.500000000000003553 ) ;
#47293=CARTESIAN_POINT ( 'NONE',  ( 113.7313622454166904, -99.85325460238200890, -19.78219314458215550 ) ) ;
#47298=CARTESIAN_POINT ( 'NONE',  ( 147.0667039024469886, -67.87844715994090450, 245.4920193514479934 ) ) ;
#47337=ADVANCED_FACE ( 'NONE', ( #75320, #37335, #65040, #85952, #23723 ), #51383, .T. ) ;
#47340=ORIENTED_EDGE ( 'NONE', *, *, #25280, .T. ) ;
#47367=DIRECTION ( 'NONE',  ( 0.7071067811865487940, -0.7071067811865463515, 0.000000000000000000 ) ) ;
#47402=EDGE_LOOP ( 'NONE', ( #66000, #37932, #57994, #41206 ) ) ;
#47408=LINE ( 'NONE', #26539, #29473 ) ;
#47409=B_SPLINE_CURVE_WITH_KNOTS ( 'NONE', 3,
 ( #54689, #47883, #75625, #13392, #8371, #70143 ),
 .UNSPECIFIED., .F., .F.,
 ( 4, 2, 4 ),
 ( -0.009174681380988100945, -0.004588847231327390468, -7.778521765323606618E-06 ),
 .UNSPECIFIED. ) ;
#47429=DIRECTION ( 'NONE',  ( 1.000000000000000078E-15, -1.000000000000000000, 0.000000000000000000 ) ) ;
#47435=CARTESIAN_POINT ( 'NONE',  ( 145.3728389244185450, -136.8603515927981107, 247.4879652615099985 ) ) ;
#47439=CARTESIAN_POINT ( 'NONE',  ( 132.2857443282840393, -124.7784471599409102, 55.21780685541800437 ) ) ;
#47445=ORIENTED_EDGE ( 'NONE', *, *, #32031, .F. ) ;
#47447=VERTEX_POINT ( 'NONE', #83938 ) ;
#47465=VERTEX_POINT ( 'NONE', #21707 ) ;
#47466=ORIENTED_EDGE ( 'NONE', *, *, #72788, .F. ) ;
#47484=DIRECTION ( 'NONE',  ( -3.100000000000000258E-29, 3.100000000000000044E-14, 1.000000000000000000 ) ) ;
#47487=ORIENTED_EDGE ( 'NONE', *, *, #71938, .T. ) ;
#47520=DIRECTION ( 'NONE',  ( 0.000000000000000000, 0.000000000000000000, 1.000000000000000000 ) ) ;
#47522=LINE ( 'NONE', #82091, #46332 ) ;
#47523=DIRECTION ( 'NONE',  ( 3.100000000000000258E-29, -3.100000000000000044E-14, -1.000000000000000000 ) ) ;
#47525=DIRECTION ( 'NONE',  ( 1.000000000000000000, 0.000000000000000000, 0.000000000000000000 ) ) ;
#47528=AXIS2_PLACEMENT_3D ( 'NONE', #30357, #58054, #87109 ) ;
#47530=EDGE_CURVE ( 'NONE', #46470, #61847, #55353, .T. ) ;
#47534=ORIENTED_EDGE ( 'NONE', *, *, #7458, .F. ) ;
#47537=CARTESIAN_POINT ( 'NONE',  ( 70.06029815369576852, -140.3870298840350870, 246.8745206071880034 ) ) ;
#47573=PLANE ( 'NONE',  #70614 ) ;
#47575=CARTESIAN_POINT ( 'NONE',  ( 74.67117555236049498, -69.13001345503671757, 247.4595024958179863 ) ) ;
#47582=EDGE_LOOP ( 'NONE', ( #41539, #3792 ) ) ;
#47595=DIRECTION ( 'NONE',  ( 3.100000000000000258E-29, -3.100000000000000044E-14, -1.000000000000000000 ) ) ;
#47600=VERTEX_POINT ( 'NONE', #89923 ) ;
#47604=DIRECTION ( 'NONE',  ( 1.000000000000000000, 0.000000000000000000, 0.000000000000000000 ) ) ;
#47617=CARTESIAN_POINT ( 'NONE',  ( 92.81932083335591699, -95.00417761012948858, -11.78219314458228695 ) ) ;
#47632=ORIENTED_EDGE ( 'NONE', *, *, #50272, .T. ) ;
#47635=EDGE_CURVE ( 'NONE', #80549, #40328, #12712, .T. ) ;
#47649=ORIENTED_EDGE ( 'NONE', *, *, #41401, .T. ) ;
#47658=DIRECTION ( 'NONE',  ( -3.100000000000000258E-29, 3.100000000000000044E-14, 1.000000000000000000 ) ) ;
#47659=CARTESIAN_POINT ( 'NONE',  ( 69.95929469538076262, -138.0461895383713795, 247.6591799766680140 ) ) ;
#47660=AXIS2_PLACEMENT_3D ( 'NONE', #2677, #43537, #71280 ) ;
#47674=ORIENTED_EDGE ( 'NONE', *, *, #20873, .T. ) ;
#47689=VERTEX_POINT ( 'NONE', #29026 ) ;
#47708=ORIENTED_EDGE ( 'NONE', *, *, #87304, .F. ) ;
#47735=CARTESIAN_POINT ( 'NONE',  ( 158.0667039024469886, -67.87844715994090450, 155.2178068554179902 ) ) ;
#47747=DIRECTION ( 'NONE',  ( -0.7071067811865473507, -0.7071067811865477948, 0.000000000000000000 ) ) ;
#47764=DIRECTION ( 'NONE',  ( 0.7071067811865477948, -0.7071067811865473507, 0.000000000000000000 ) ) ;
#47771=EDGE_CURVE ( 'NONE', #75678, #33892, #57199, .T. ) ;
#47787=VERTEX_POINT ( 'NONE', #16294 ) ;
#47794=ORIENTED_EDGE ( 'NONE', *, *, #42428, .T. ) ;
#47802=CARTESIAN_POINT ( 'NONE',  ( 70.56670390244700286, -67.87844715994098976, 180.4678068554179902 ) ) ;
#47829=ORIENTED_EDGE ( 'NONE', *, *, #54065, .T. ) ;
#47830=ORIENTED_EDGE ( 'NONE', *, *, #28833, .F. ) ;
#47835=EDGE_LOOP ( 'NONE', ( #27927, #40921 ) ) ;
#47851=DIRECTION ( 'NONE',  ( 3.100000000000000258E-29, -3.100000000000000044E-14, -1.000000000000000000 ) ) ;
#47883=CARTESIAN_POINT ( 'NONE',  ( 70.06670390244707392, -140.6784471599409869, 245.4568581461520012 ) ) ;
#47922=VECTOR ( 'NONE', #2254, 1000.000000000000000 ) ;
#47931=CARTESIAN_POINT ( 'NONE',  ( 106.1318753153733070, -87.31936784520605954, -19.21046202161352667 ) ) ;
#47939=CARTESIAN_POINT ( 'NONE',  ( 107.0667039024470313, -104.2784471599409528, 25.71780685541800437 ) ) ;
#47947=CARTESIAN_POINT ( 'NONE',  ( 67.06670390244701707, -79.67844715994098692, 222.2178068554179902 ) ) ;
#47951=EDGE_CURVE ( 'NONE', #75555, #55721, #38069, .T. ) ;
#47989=DIRECTION ( 'NONE',  ( 1.000000000000000078E-15, -1.000000000000000000, 0.000000000000000000 ) ) ;
#48018=CARTESIAN_POINT ( 'NONE',  ( 145.2601077436562207, -69.52476574176742474, 247.4934834993690060 ) ) ;
#48020=ADVANCED_FACE ( 'NONE', ( #13056 ), #26222, .F. ) ;
#48025=CIRCLE ( 'NONE', #68416, 8.999999999999994671 ) ;
#48031=VERTEX_POINT ( 'NONE', #89361 ) ;
#48038=CARTESIAN_POINT ( 'NONE',  ( 110.0324702783101571, -120.0661611444839991, -21.02845593540760305 ) ) ;
#48044=ORIENTED_EDGE ( 'NONE', *, *, #71641, .T. ) ;
#48060=LINE ( 'NONE', #88977, #43771 ) ;
#48088=LINE ( 'NONE', #62180, #79157 ) ;
#48089=ORIENTED_EDGE ( 'NONE', *, *, #88602, .T. ) ;
#48090=AXIS2_PLACEMENT_3D ( 'NONE', #170, #21527, #63751 ) ;
#48102=ORIENTED_EDGE ( 'NONE', *, *, #43413, .T. ) ;
#48114=CARTESIAN_POINT ( 'NONE',  ( 144.0667052733537901, -71.37844715994090450, 222.2178068554179902 ) ) ;
#48122=LINE ( 'NONE', #30393, #50382 ) ;
#48140=EDGE_CURVE ( 'NONE', #35902, #22318, #22546, .T. ) ;
#48141=CARTESIAN_POINT ( 'NONE',  ( 99.08946256649485917, -109.4614598618343138, -19.78219314458184996 ) ) ;
#48142=CARTESIAN_POINT ( 'NONE',  ( 137.0667039024470739, -118.2784471599408960, 51.21780685541800437 ) ) ;
#48154=VECTOR ( 'NONE', #57141, 1000.000000000000000 ) ;
#48158=ORIENTED_EDGE ( 'NONE', *, *, #31514, .T. ) ;
#48199=CARTESIAN_POINT ( 'NONE',  ( 138.8356781741756265, -107.9363541596096212, 249.3055338466990065 ) ) ;
#48200=VERTEX_POINT ( 'NONE', #57052 ) ;
#48202=DIRECTION ( 'NONE',  ( 0.000000000000000000, 0.000000000000000000, 1.000000000000000000 ) ) ;
#48210=FACE_BOUND ( 'NONE', #84389, .T. ) ;
#48216=CIRCLE ( 'NONE', #1835, 7.999999999999992895 ) ;
#48220=CARTESIAN_POINT ( 'NONE',  ( 147.0667039024470739, -137.6773508071221954, 245.4788300746780010 ) ) ;
#48221=EDGE_CURVE ( 'NONE', #8011, #80877, #32621, .T. ) ;
#48243=EDGE_CURVE ( 'NONE', #3381, #63429, #43873, .T. ) ;
#48291=CARTESIAN_POINT ( 'NONE',  ( 110.7536356736639078, -102.7271463785351528, 2.217806855417947531 ) ) ;
#48302=ORIENTED_EDGE ( 'NONE', *, *, #16515, .F. ) ;
#48324=CARTESIAN_POINT ( 'NONE',  ( 91.91125933621954402, -111.9799080603168449, -11.78219314458175937 ) ) ;
#48329=CARTESIAN_POINT ( 'NONE',  ( 67.66273711577628092, -68.45061131148345623, 246.9170789443036824 ) ) ;
#48346=EDGE_LOOP ( 'NONE', ( #19182, #38649, #20561, #49657 ) ) ;
#48348=CARTESIAN_POINT ( 'NONE',  ( 144.1741131095133994, -138.0461895383712942, 247.6591799766680140 ) ) ;
#48361=CIRCLE ( 'NONE', #12153, 1.500000000000001332 ) ;
#48383=EDGE_CURVE ( 'NONE', #34061, #51923, #87012, .T. ) ;
#48384=CARTESIAN_POINT ( 'NONE',  ( 97.81670390244700286, -67.87844715994096134, 55.21780685541800437 ) ) ;
#48409=ORIENTED_EDGE ( 'NONE', *, *, #3850, .F. ) ;
#48418=PLANE ( 'NONE',  #78890 ) ;
#48419=CARTESIAN_POINT ( 'NONE',  ( 145.3807741851185824, -139.2458688871068375, 246.2343294490942753 ) ) ;
#48437=EDGE_CURVE ( 'NONE', #76266, #30286, #52446, .T. ) ;
#48438=CARTESIAN_POINT ( 'NONE',  ( 107.0667039024470313, -104.2784471599420755, -19.78219314458201694 ) ) ;
#48475=CARTESIAN_POINT ( 'NONE',  ( 107.5667039024470313, -100.3098201933444926, 2.217806855417892020 ) ) ;
#48478=CYLINDRICAL_SURFACE ( 'NONE', #54723, 23.50000000000000711 ) ;
#48484=AXIS2_PLACEMENT_3D ( 'NONE', #52834, #31539, #16589 ) ;
#48494=CARTESIAN_POINT ( 'NONE',  ( 115.5439452383991892, -99.96145986183427112, -19.78219314458215550 ) ) ;
#48519=ADVANCED_FACE ( 'NONE', ( #33377 ), #68355, .F. ) ;
#48522=CARTESIAN_POINT ( 'NONE',  ( 52.56670390244699576, -68.37844715994100397, 180.4678068554179902 ) ) ;
#48548=AXIS2_PLACEMENT_3D ( 'NONE', #48522, #43066, #7233 ) ;
#48557=EDGE_CURVE ( 'NONE', #53716, #49237, #60945, .T. ) ;
#48558=VECTOR ( 'NONE', #36845, 1000.000000000000000 ) ;
#48600=DIRECTION ( 'NONE',  ( -1.000000000000000000, -1.000000000000000078E-15, 0.000000000000000000 ) ) ;
#48630=AXIS2_PLACEMENT_3D ( 'NONE', #36157, #29353, #49766 ) ;
#48633=AXIS2_PLACEMENT_3D ( 'NONE', #15400, #43067, #6329 ) ;
#48636=ADVANCED_FACE ( 'NONE', ( #7911 ), #69249, .F. ) ;
#48646=CARTESIAN_POINT ( 'NONE',  ( 145.9305329516949143, -89.25781324566730746, 247.4783998280190076 ) ) ;
#48648=ORIENTED_EDGE ( 'NONE', *, *, #60323, .F. ) ;
#48654=DIRECTION ( 'NONE',  ( -0.000000000000000000, -0.000000000000000000, -1.000000000000000000 ) ) ;
#48656=AXIS2_PLACEMENT_3D ( 'NONE', #19252, #19694, #87846 ) ;
#48664=EDGE_CURVE ( 'NONE', #30086, #78255, #77715, .T. ) ;
#48673=DIRECTION ( 'NONE',  ( 0.000000000000000000, 0.000000000000000000, -1.000000000000000000 ) ) ;
#48684=VECTOR ( 'NONE', #29481, 999.9999999999998863 ) ;
#48702=ORIENTED_EDGE ( 'NONE', *, *, #19973, .T. ) ;
#48704=EDGE_CURVE ( 'NONE', #61361, #37855, #41463, .T. ) ;
#48717=CARTESIAN_POINT ( 'NONE',  ( 94.87702571208353675, -93.81616114448341648, -21.02845593540959968 ) ) ;
#48730=CARTESIAN_POINT ( 'NONE',  ( 68.69170846778827411, -139.3034517252403930, 245.6607681749549386 ) ) ;
#48757=EDGE_LOOP ( 'NONE', ( #65145, #84960 ) ) ;
#48762=CARTESIAN_POINT ( 'NONE',  ( 91.91125933621930244, -98.95301919085837028, -21.02845593540826741 ) ) ;
#48763=VERTEX_POINT ( 'NONE', #37860 ) ;
#48782=CARTESIAN_POINT ( 'NONE',  ( 90.06670390244703128, -106.9675116026789539, -9.937637710809946512 ) ) ;
#48791=CARTESIAN_POINT ( 'NONE',  ( 145.7412724758569027, -69.14289728258658840, 247.3817316427832793 ) ) ;
#48792=CARTESIAN_POINT ( 'NONE',  ( 92.91125933621933086, -94.95109689075250969, -21.78219314458229405 ) ) ;
#48802=ORIENTED_EDGE ( 'NONE', *, *, #46827, .T. ) ;
#48807=AXIS2_PLACEMENT_3D ( 'NONE', #10289, #3476, #44347 ) ;
#48844=PLANE ( 'NONE',  #6177 ) ;
#48848=CARTESIAN_POINT ( 'NONE',  ( 110.0667047667142953, -67.87844715994094713, 93.21780685541800437 ) ) ;
#48853=VERTEX_POINT ( 'NONE', #80099 ) ;
#48854=EDGE_CURVE ( 'NONE', #55635, #86394, #85583, .T. ) ;
#48859=CARTESIAN_POINT ( 'NONE',  ( 107.0667039024470313, -104.2784471599421323, -21.78219314458201694 ) ) ;
#48874=DIRECTION ( 'NONE',  ( 1.000000000000000000, 1.150535366796005147E-15, -4.666596370676151832E-30 ) ) ;
#48879=ORIENTED_EDGE ( 'NONE', *, *, #46651, .F. ) ;
#48886=LINE ( 'NONE', #70710, #30368 ) ;
#48894=ORIENTED_EDGE ( 'NONE', *, *, #16873, .T. ) ;
#48916=EDGE_CURVE ( 'NONE', #75012, #74274, #86902, .T. ) ;
#48931=VECTOR ( 'NONE', #19140, 1000.000000000000114 ) ;
#48935=LINE ( 'NONE', #14458, #70724 ) ;
#48939=DIRECTION ( 'NONE',  ( 1.000000000000000078E-15, -1.000000000000000000, 0.000000000000000000 ) ) ;
#48940=CARTESIAN_POINT ( 'NONE',  ( 107.0667039024470313, -104.2784471599420897, -20.48315503890502143 ) ) ;
#48962=CARTESIAN_POINT ( 'NONE',  ( 99.08946256649485917, -109.4614598618336174, 2.217806855418169576 ) ) ;
#48969=ORIENTED_EDGE ( 'NONE', *, *, #70347, .T. ) ;
#48972=EDGE_LOOP ( 'NONE', ( #4207, #68750, #18548, #6282 ) ) ;
#48977=DIRECTION ( 'NONE',  ( 0.000000000000000000, 0.000000000000000000, 1.000000000000000000 ) ) ;
#48992=ORIENTED_EDGE ( 'NONE', *, *, #54781, .F. ) ;
#49003=EDGE_CURVE ( 'NONE', #9196, #82603, #11490, .T. ) ;
#49066=EDGE_LOOP ( 'NONE', ( #18050, #82095, #34371 ) ) ;
#49068=CARTESIAN_POINT ( 'NONE',  ( 74.06670390244704549, -118.2784471599409812, 45.21780685541799727 ) ) ;
#49070=FACE_OUTER_BOUND ( 'NONE', #12244, .T. ) ;
#49074=LINE ( 'NONE', #61815, #77092 ) ;
#49105=LINE ( 'NONE', #86, #89590 ) ;
#49149=CARTESIAN_POINT ( 'NONE',  ( 107.0667039024470313, -104.2784471599408676, 19.21780685541799016 ) ) ;
#49153=DIRECTION ( 'NONE',  ( 0.000000000000000000, 0.000000000000000000, 1.000000000000000000 ) ) ;
#49173=CARTESIAN_POINT ( 'NONE',  ( 70.77521666129561595, -139.2590457508245265, 247.4515711584743087 ) ) ;
#49185=CARTESIAN_POINT ( 'NONE',  ( 68.70527646626339902, -139.2915593431212358, 245.9274751462549204 ) ) ;
#49196=CARTESIAN_POINT ( 'NONE',  ( 124.6905118036816305, -125.4749327540681492, 250.2178068554179902 ) ) ;
#49237=VERTEX_POINT ( 'NONE', #63214 ) ;
#49239=ORIENTED_EDGE ( 'NONE', *, *, #5940, .T. ) ;
#49251=CARTESIAN_POINT ( 'NONE',  ( 107.0667039024470313, -104.2784471599413934, 2.217806855418003043 ) ) ;
#49274=VERTEX_POINT ( 'NONE', #50016 ) ;
#49290=EDGE_CURVE ( 'NONE', #43695, #65034, #77775, .T. ) ;
#49292=AXIS2_PLACEMENT_3D ( 'NONE', #61118, #51719, #24051 ) ;
#49323=CARTESIAN_POINT ( 'NONE',  ( 143.5667039024469886, -68.87844715994090450, 55.21780685541800437 ) ) ;
#49332=AXIS2_PLACEMENT_3D ( 'NONE', #83305, #29673, #21986 ) ;
#49333=CARTESIAN_POINT ( 'NONE',  ( 68.06670390244701707, -86.77844715994098124, 55.21780685541800437 ) ) ;
#49341=ORIENTED_EDGE ( 'NONE', *, *, #38492, .T. ) ;
#49360=DIRECTION ( 'NONE',  ( 3.100000000000000258E-29, -3.100000000000000044E-14, -1.000000000000000000 ) ) ;
#49367=EDGE_CURVE ( 'NONE', #49424, #33950, #65452, .T. ) ;
#49377=VERTEX_POINT ( 'NONE', #24565 ) ;
#49378=ORIENTED_EDGE ( 'NONE', *, *, #47208, .T. ) ;
#49388=CARTESIAN_POINT ( 'NONE',  ( 107.5667039024470313, -100.3098201933451605, -19.78219314458212708 ) ) ;
#49395=CARTESIAN_POINT ( 'NONE',  ( 115.5439452383992176, -108.5954344580491551, 2.217806855418142042 ) ) ;
#49410=DIRECTION ( 'NONE',  ( -1.000000000000000000, 0.000000000000000000, 0.000000000000000000 ) ) ;
#49420=DIRECTION ( 'NONE',  ( -3.100000000000000258E-29, 3.100000000000000044E-14, 1.000000000000000000 ) ) ;
#49424=VERTEX_POINT ( 'NONE', #52232 ) ;
#49431=CARTESIAN_POINT ( 'NONE',  ( 110.2536356736639078, -101.8611209747507189, 2.217806855417919998 ) ) ;
#49443=DIRECTION ( 'NONE',  ( -0.7759704746411383303, 0.6307692307692303046, 0.000000000000000000 ) ) ;
#49471=VECTOR ( 'NONE', #75564, 1000.000000000000000 ) ;
#49478=CARTESIAN_POINT ( 'NONE',  ( 68.80140062917963917, -69.47028513356498536, 247.4826175141195108 ) ) ;
#49520=VECTOR ( 'NONE', #75172, 1000.000000000000000 ) ;
#49525=CARTESIAN_POINT ( 'NONE',  ( 67.06683615445079738, -81.17077867087118648, 245.9554665702709997 ) ) ;
#49527=DIRECTION ( 'NONE',  ( -1.000000000000000078E-15, 1.000000000000000000, 0.000000000000000000 ) ) ;
#49531=CARTESIAN_POINT ( 'NONE',  ( 67.06670390210777555, -137.6784471596019728, 245.4218662566959779 ) ) ;
#49544=DIRECTION ( 'NONE',  ( 0.000000000000000000, 0.000000000000000000, 1.000000000000000000 ) ) ;
#49549=LINE ( 'NONE', #84565, #21046 ) ;
#49550=ORIENTED_EDGE ( 'NONE', *, *, #78959, .F. ) ;
#49563=ORIENTED_EDGE ( 'NONE', *, *, #22226, .T. ) ;
#49569=EDGE_CURVE ( 'NONE', #48031, #77074, #53573, .T. ) ;
#49580=DIRECTION ( 'NONE',  ( -1.000000000000000078E-15, 1.000000000000000000, 0.000000000000000000 ) ) ;
#49583=LINE ( 'NONE', #42321, #1252 ) ;
#49629=VERTEX_POINT ( 'NONE', #40859 ) ;
#49638=DIRECTION ( 'NONE',  ( -3.100000000000000258E-29, 3.100000000000000044E-14, 1.000000000000000000 ) ) ;
#49642=CYLINDRICAL_SURFACE ( 'NONE', #34374, 3.500000000000003109 ) ;
#49651=LINE ( 'NONE', #28313, #38877 ) ;
#49657=ORIENTED_EDGE ( 'NONE', *, *, #63577, .T. ) ;
#49670=CARTESIAN_POINT ( 'NONE',  ( 107.0667039024470313, -104.2784471599409528, 22.21780685541800082 ) ) ;
#49677=ORIENTED_EDGE ( 'NONE', *, *, #56375, .F. ) ;
#49679=ADVANCED_FACE ( 'NONE', ( #34943 ), #27238, .F. ) ;
#49681=DIRECTION ( 'NONE',  ( 1.000000000000000078E-15, -1.000000000000000000, 0.000000000000000000 ) ) ;
#49715=ADVANCED_FACE ( 'NONE', ( #54916 ), #11151, .T. ) ;
#49719=ADVANCED_FACE ( 'NONE', ( #87029 ), #31152, .T. ) ;
#49736=DIRECTION ( 'NONE',  ( 0.000000000000000000, 0.000000000000000000, 1.000000000000000000 ) ) ;
#49756=CARTESIAN_POINT ( 'NONE',  ( 146.5585094824388648, -137.3868253791688687, 246.8399677638830667 ) ) ;
#49766=DIRECTION ( 'NONE',  ( 1.000000000000000000, 8.953411488912556626E-16, 0.000000000000000000 ) ) ;
#49788=EDGE_CURVE ( 'NONE', #78225, #11071, #73382, .T. ) ;
#49794=AXIS2_PLACEMENT_3D ( 'NONE', #37346, #30533, #65053 ) ;
#49850=CARTESIAN_POINT ( 'NONE',  ( 63.06670390244699576, -67.87844715994098976, 85.21780685541799016 ) ) ;
#49859=CARTESIAN_POINT ( 'NONE',  ( 107.0667039024470313, -104.2784471599413934, 2.217806855418003043 ) ) ;
#49881=DIRECTION ( 'NONE',  ( 1.777766061779359009E-15, -1.000000000000000000, 3.100000000000000044E-14 ) ) ;
#49888=PLANE ( 'NONE',  #48633 ) ;
#49945=DIRECTION ( 'NONE',  ( 0.7071067811865483499, 0.7071067811865466846, 0.000000000000000000 ) ) ;
#49952=ORIENTED_EDGE ( 'NONE', *, *, #15251, .T. ) ;
#49973=CARTESIAN_POINT ( 'NONE',  ( 67.35067855263200443, -81.16520196425757661, 246.8834897342799763 ) ) ;
#50009=CARTESIAN_POINT ( 'NONE',  ( 126.1218394983595630, -84.35882332054457322, 250.2178068554179333 ) ) ;
#50016=CARTESIAN_POINT ( 'NONE',  ( 63.06670390244699576, -67.87844715994098976, 120.2178068554179902 ) ) ;
#50024=CARTESIAN_POINT ( 'NONE',  ( 104.1009375265838486, -88.49073317540022288, -21.02845593540859426 ) ) ;
#50027=DIRECTION ( 'NONE',  ( -1.000000000000000000, -1.000000000000000078E-15, 0.000000000000000000 ) ) ;
#50037=DIRECTION ( 'NONE',  ( 1.000000000000000078E-15, -1.000000000000000000, 0.000000000000000000 ) ) ;
#50049=VERTEX_POINT ( 'NONE', #62880 ) ;
#50074=CARTESIAN_POINT ( 'NONE',  ( 70.87602654543734104, -139.0212896760968420, 247.5093344598249701 ) ) ;
#50075=AXIS2_PLACEMENT_3D ( 'NONE', #27441, #71037, #83769 ) ;
#50085=CARTESIAN_POINT ( 'NONE',  ( 68.71873216121885264, -139.2787739119035280, 246.0441243801330700 ) ) ;
#50111=CARTESIAN_POINT ( 'NONE',  ( 99.08946256649487339, -99.09543445804985140, -19.78219314458218392 ) ) ;
#50114=ADVANCED_FACE ( 'NONE', ( #10164 ), #74171, .F. ) ;
#50115=DIRECTION ( 'NONE',  ( -1.000000000000000078E-15, 1.000000000000000000, 0.000000000000000000 ) ) ;
#50117=CARTESIAN_POINT ( 'NONE',  ( 145.9203257412752919, -138.8248129988771211, 246.0151717635989996 ) ) ;
#50122=VECTOR ( 'NONE', #33155, 1000.000000000000000 ) ;
#50124=AXIS2_PLACEMENT_3D ( 'NONE', #22438, #50115, #42847 ) ;
#50134=CARTESIAN_POINT ( 'NONE',  ( 67.06980256514445671, -67.88054560554753891, 245.6023804759829829 ) ) ;
#50136=ORIENTED_EDGE ( 'NONE', *, *, #17389, .T. ) ;
#50137=EDGE_LOOP ( 'NONE', ( #19652, #32081, #57439, #46595, #74840, #38345 ) ) ;
#50148=ADVANCED_FACE ( 'NONE', ( #79672 ), #66002, .T. ) ;
#50187=AXIS2_PLACEMENT_3D ( 'NONE', #53106, #47658, #60846 ) ;
#50190=VECTOR ( 'NONE', #66781, 1000.000000000000000 ) ;
#50201=DIRECTION ( 'NONE',  ( 1.000000000000000078E-15, -1.000000000000000000, 0.000000000000000000 ) ) ;
#50202=CARTESIAN_POINT ( 'NONE',  ( 140.0667039024470455, -118.2784471599408960, 45.21780685541799727 ) ) ;
#50205=EDGE_CURVE ( 'NONE', #76783, #43325, #18308, .T. ) ;
#50217=LINE ( 'NONE', #77952, #15337 ) ;
#50221=DIRECTION ( 'NONE',  ( 3.100000000000000258E-29, -3.100000000000000044E-14, -1.000000000000000000 ) ) ;
#50223=EDGE_LOOP ( 'NONE', ( #39031, #80194, #24817, #12793 ) ) ;
#50224=ORIENTED_EDGE ( 'NONE', *, *, #25267, .T. ) ;
#50237=ORIENTED_EDGE ( 'NONE', *, *, #68135, .F. ) ;
#50239=DIRECTION ( 'NONE',  ( 0.000000000000000000, 0.000000000000000000, -1.000000000000000000 ) ) ;
#50249=DIRECTION ( 'NONE',  ( -1.000000000000000000, 0.000000000000000000, 0.000000000000000000 ) ) ;
#50260=CYLINDRICAL_SURFACE ( 'NONE', #85975, 30.99999999999998579 ) ;
#50272=EDGE_CURVE ( 'NONE', #86794, #61024, #5592, .T. ) ;
#50297=EDGE_CURVE ( 'NONE', #4100, #63429, #43217, .T. ) ;
#50303=CARTESIAN_POINT ( 'NONE',  ( 140.0667039024470455, -118.2784471599408960, 45.21780685541799727 ) ) ;
#50306=CARTESIAN_POINT ( 'NONE',  ( 154.5667039024469886, -67.87844715994090450, 85.21780685541799016 ) ) ;
#50324=AXIS2_PLACEMENT_3D ( 'NONE', #80903, #54031, #47232 ) ;
#50325=CIRCLE ( 'NONE', #44484, 27.49999999999999645 ) ;
#50334=AXIS2_PLACEMENT_3D ( 'NONE', #15642, #71063, #8834 ) ;
#50337=EDGE_CURVE ( 'NONE', #56758, #20355, #69199, .T. ) ;
#50358=EDGE_CURVE ( 'NONE', #22506, #25248, #56848, .T. ) ;
#50364=LINE ( 'NONE', #85821, #80369 ) ;
#50374=VECTOR ( 'NONE', #39777, 1000.000000000000000 ) ;
#50382=VECTOR ( 'NONE', #50831, 1000.000000000000000 ) ;
#50385=ORIENTED_EDGE ( 'NONE', *, *, #79357, .T. ) ;
#50393=CARTESIAN_POINT ( 'NONE',  ( 110.0667047667142953, -67.87844715994094713, 173.2178068554179902 ) ) ;
#50410=CARTESIAN_POINT ( 'NONE',  ( 103.3797721312301547, -105.8297479413482876, -19.78219314458196010 ) ) ;
#50411=PLANE ( 'NONE',  #27461 ) ;
#50440=DIRECTION ( 'NONE',  ( 3.100000000000000258E-29, -3.100000000000000044E-14, -1.000000000000000000 ) ) ;
#50458=CARTESIAN_POINT ( 'NONE',  ( 121.5948191693370717, -80.85146542362632260, 250.2178068554179902 ) ) ;
#50460=ADVANCED_FACE ( 'NONE', ( #51367, #58632, #79561, #31827, #45001 ), #57753, .T. ) ;
#50463=CIRCLE ( 'NONE', #62078, 17.00000000000000000 ) ;
#50465=ORIENTED_EDGE ( 'NONE', *, *, #4803, .T. ) ;
#50493=DIRECTION ( 'NONE',  ( 3.100000000000000258E-29, -3.100000000000000044E-14, -1.000000000000000000 ) ) ;
#50499=CARTESIAN_POINT ( 'NONE',  ( 99.48898161933323081, -117.4034471599418197, -11.78219314458159239 ) ) ;
#50512=EDGE_CURVE ( 'NONE', #65273, #22589, #3905, .T. ) ;
#50525=ORIENTED_EDGE ( 'NONE', *, *, #60431, .F. ) ;
#50535=( LENGTH_UNIT ( ) NAMED_UNIT ( * ) SI_UNIT ( .MILLI., .METRE. ) );
#50545=DIRECTION ( 'NONE',  ( 3.100000000000000258E-29, -3.100000000000000044E-14, -1.000000000000000000 ) ) ;
#50571=AXIS2_PLACEMENT_3D ( 'NONE', #14811, #28418, #8439 ) ;
#50572=CARTESIAN_POINT ( 'NONE',  ( 144.5619505544954393, -138.4421194277352924, 247.5996269027399990 ) ) ;
#50625=ORIENTED_EDGE ( 'NONE', *, *, #50808, .T. ) ;
#50631=DIRECTION ( 'NONE',  ( 3.100000000000000258E-29, -3.100000000000000044E-14, -1.000000000000000000 ) ) ;
#50656=AXIS2_PLACEMENT_3D ( 'NONE', #89656, #19265, #5642 ) ;
#50661=DIRECTION ( 'NONE',  ( 0.7071067811865473507, 0.7071067811865477948, 0.000000000000000000 ) ) ;
#50668=PLANE ( 'NONE',  #7269 ) ;
#50671=CARTESIAN_POINT ( 'NONE',  ( 144.0654454572467671, -140.6784471599409017, 245.5026818079589930 ) ) ;
#50674=EDGE_CURVE ( 'NONE', #10101, #36821, #32269, .T. ) ;
#50698=CARTESIAN_POINT ( 'NONE',  ( 145.5667039024470739, -139.1784471599409017, 228.4678068554179902 ) ) ;
#50699=AXIS2_PLACEMENT_3D ( 'NONE', #88368, #5692, #4789 ) ;
#50707=CARTESIAN_POINT ( 'NONE',  ( 82.78637150392543731, -91.25622735614753367, 250.2178068554179902 ) ) ;
#50709=AXIS2_PLACEMENT_3D ( 'NONE', #21502, #1506, #76906 ) ;
#50711=EDGE_CURVE ( 'NONE', #84863, #61024, #6883, .T. ) ;
#50717=FACE_OUTER_BOUND ( 'NONE', #9075, .T. ) ;
#50726=FACE_OUTER_BOUND ( 'NONE', #62921, .T. ) ;
#50795=ORIENTED_EDGE ( 'NONE', *, *, #71198, .T. ) ;
#50808=EDGE_CURVE ( 'NONE', #15323, #86096, #48122, .T. ) ;
#50809=ORIENTED_EDGE ( 'NONE', *, *, #16917, .F. ) ;
#50831=DIRECTION ( 'NONE',  ( -1.000000000000000000, -1.000000000000000078E-15, 0.000000000000000000 ) ) ;
#50833=DIRECTION ( 'NONE',  ( 0.000000000000000000, 0.000000000000000000, -1.000000000000000000 ) ) ;
#50859=EDGE_CURVE ( 'NONE', #24431, #68999, #6712, .T. ) ;
#50886=ORIENTED_EDGE ( 'NONE', *, *, #61878, .T. ) ;
#50906=DIRECTION ( 'NONE',  ( -1.000000000000000078E-15, 1.000000000000000000, 0.000000000000000000 ) ) ;
#50911=CARTESIAN_POINT ( 'NONE',  ( 127.0667052882549797, -78.66107132697005966, 55.21780685541800437 ) ) ;
#50944=CIRCLE ( 'NONE', #18981, 3.500000000000003109 ) ;
#50959=ORIENTED_EDGE ( 'NONE', *, *, #20900, .T. ) ;
#50980=FACE_OUTER_BOUND ( 'NONE', #88040, .T. ) ;
#50987=CARTESIAN_POINT ( 'NONE',  ( 69.02879735949464646, -138.9723707447056142, 246.9664177707386159 ) ) ;
#51007=EDGE_LOOP ( 'NONE', ( #27015, #7938, #76531, #17795 ) ) ;
#51036=AXIS2_PLACEMENT_3D ( 'NONE', #7202, #6300, #5868 ) ;
#51044=CARTESIAN_POINT ( 'NONE',  ( 107.0667039024470739, -140.6784471599409301, 55.21780685541800437 ) ) ;
#51068=CIRCLE ( 'NONE', #9021, 11.49999999999999645 ) ;
#51078=CARTESIAN_POINT ( 'NONE',  ( 79.84748767001921976, -82.36537145558867223, 249.3055308415380011 ) ) ;
#51088=CARTESIAN_POINT ( 'NONE',  ( 121.2221484686747317, -94.95109689075241022, -19.26696060647628528 ) ) ;
#51113=VERTEX_POINT ( 'NONE', #19890 ) ;
#51116=EDGE_LOOP ( 'NONE', ( #44563, #83400, #84440, #51263, #32731 ) ) ;
#51124=PLANE ( 'NONE',  #13461 ) ;
#51127=CARTESIAN_POINT ( 'NONE',  ( 59.56670390244699576, -67.87844715994098976, 85.21780685541799016 ) ) ;
#51135=CARTESIAN_POINT ( 'NONE',  ( 106.5667039024470313, -100.3098201933451747, -19.78219314458212708 ) ) ;
#51139=CARTESIAN_POINT ( 'NONE',  ( 147.0667039024469886, -67.87844715994090450, 222.2178068554179902 ) ) ;
#51141=CARTESIAN_POINT ( 'NONE',  ( 67.06674172433055503, -67.87844715943892027, 245.5060123894820379 ) ) ;
#51143=EDGE_CURVE ( 'NONE', #65875, #35035, #89389, .T. ) ;
#51145=VECTOR ( 'NONE', #39644, 1000.000000000000114 ) ;
#51153=CARTESIAN_POINT ( 'NONE',  ( 107.0667039024470313, -104.2784471599409528, 249.2178068554179902 ) ) ;
#51162=EDGE_CURVE ( 'NONE', #34428, #53716, #29365, .T. ) ;
#51163=DIRECTION ( 'NONE',  ( 1.000000000000000000, 1.000000000000000078E-15, -0.000000000000000000 ) ) ;
#51197=PLANE ( 'NONE',  #51264 ) ;
#51203=ORIENTED_EDGE ( 'NONE', *, *, #29367, .F. ) ;
#51218=CARTESIAN_POINT ( 'NONE',  ( 144.5667039024470171, -90.27844715994091018, 51.21780685541800437 ) ) ;
#51228=VERTEX_POINT ( 'NONE', #46071 ) ;
#51239=DIRECTION ( 'NONE',  ( 0.000000000000000000, 0.000000000000000000, 1.000000000000000000 ) ) ;
#51263=ORIENTED_EDGE ( 'NONE', *, *, #14113, .T. ) ;
#51264=AXIS2_PLACEMENT_3D ( 'NONE', #31657, #29892, #43487 ) ;
#51265=DIRECTION ( 'NONE',  ( -1.000000000000000000, -8.953411488912552682E-16, 0.000000000000000000 ) ) ;
#51312=ADVANCED_FACE ( 'NONE', ( #59711 ), #87445, .F. ) ;
#51344=EDGE_CURVE ( 'NONE', #73928, #69134, #77391, .T. ) ;
#51345=VERTEX_POINT ( 'NONE', #36052 ) ;
#51367=FACE_BOUND ( 'NONE', #58819, .T. ) ;
#51370=CARTESIAN_POINT ( 'NONE',  ( 112.7927988201233944, -69.16395658370818467, 247.7076816059330042 ) ) ;
#51383=PLANE ( 'NONE',  #47002 ) ;
#51391=ORIENTED_EDGE ( 'NONE', *, *, #63660, .T. ) ;
#51404=EDGE_CURVE ( 'NONE', #80549, #17803, #14727, .T. ) ;
#51410=EDGE_CURVE ( 'NONE', #88510, #37203, #7897, .T. ) ;
#51419=DIRECTION ( 'NONE',  ( 0.8660254037844392627, -0.4999999999999990008, 1.549999999999999706E-14 ) ) ;
#51422=CARTESIAN_POINT ( 'NONE',  ( 69.24472453127575022, -138.7583646271384055, 247.2489375779490501 ) ) ;
#51440=ORIENTED_EDGE ( 'NONE', *, *, #68548, .F. ) ;
#51445=ORIENTED_EDGE ( 'NONE', *, *, #72767, .T. ) ;
#51446=DIRECTION ( 'NONE',  ( -8.953411488912552682E-16, 1.000000000000000000, 0.000000000000000000 ) ) ;
#51450=DIRECTION ( 'NONE',  ( -3.100000000000000258E-29, 3.100000000000000044E-14, 1.000000000000000000 ) ) ;
#51451=DIRECTION ( 'NONE',  ( 1.777766061779359009E-15, -1.000000000000000000, 3.100000000000000044E-14 ) ) ;
#51453=CARTESIAN_POINT ( 'NONE',  ( 146.3532711110487980, -136.6656657599555160, 247.3338320286590033 ) ) ;
#51466=CARTESIAN_POINT ( 'NONE',  ( 70.06670390244707392, -137.6784471599409869, 55.21780685541800437 ) ) ;
#51473=ORIENTED_EDGE ( 'NONE', *, *, #61511, .T. ) ;
#51478=EDGE_CURVE ( 'NONE', #42555, #59958, #29685, .T. ) ;
#51480=VECTOR ( 'NONE', #21766, 1000.000000000000000 ) ;
#51506=ADVANCED_FACE ( 'NONE', ( #36944 ), #41745, .T. ) ;
#51527=CARTESIAN_POINT ( 'NONE',  ( 143.7940362993692531, -140.2217314834169315, 246.8063787849100095 ) ) ;
#51531=DIRECTION ( 'NONE',  ( 1.000000000000000000, 0.000000000000000000, 0.000000000000000000 ) ) ;
#51535=CARTESIAN_POINT ( 'NONE',  ( 67.56422611121462296, -137.3915314758240811, 246.8274931754388604 ) ) ;
#51560=CARTESIAN_POINT ( 'NONE',  ( 140.0667039024470455, -118.2784471599408960, 51.21780685541800437 ) ) ;
#51561=ORIENTED_EDGE ( 'NONE', *, *, #79471, .T. ) ;
#51566=EDGE_CURVE ( 'NONE', #8767, #67043, #44187, .T. ) ;
#51575=DIRECTION ( 'NONE',  ( 1.000000000000000000, 1.000000000000000078E-15, 0.000000000000000000 ) ) ;
#51584=ORIENTED_EDGE ( 'NONE', *, *, #72483, .T. ) ;
#51596=ORIENTED_EDGE ( 'NONE', *, *, #9367, .F. ) ;
#51597=DIRECTION ( 'NONE',  ( 1.000000000000000000, 1.000000000000000078E-15, 0.000000000000000000 ) ) ;
#51601=CARTESIAN_POINT ( 'NONE',  ( 106.1656040943334460, -121.2545485715094316, -21.78219314458149114 ) ) ;
#51610=EDGE_LOOP ( 'NONE', ( #5264, #82151, #85639, #54715 ) ) ;
#51619=CARTESIAN_POINT ( 'NONE',  ( 103.2030832344709381, -107.0864598618342995, -19.78219314458193168 ) ) ;
#51638=DIRECTION ( 'NONE',  ( 1.000000000000000000, 1.000000000000000078E-15, 0.000000000000000000 ) ) ;
#51648=CARTESIAN_POINT ( 'NONE',  ( 74.85599922111907745, -133.5313194959603607, 248.4142799812389910 ) ) ;
#51667=CARTESIAN_POINT ( 'NONE',  ( 69.56670390244701707, -85.27844715994098124, 55.21780685541800437 ) ) ;
#51708=CARTESIAN_POINT ( 'NONE',  ( 91.91125933621951560, -96.57698625956682292, -11.78219314458225853 ) ) ;
#51719=DIRECTION ( 'NONE',  ( -1.000000000000000078E-15, 1.000000000000000000, 0.000000000000000000 ) ) ;
#51720=CARTESIAN_POINT ( 'NONE',  ( 91.91441891875214765, -111.9861225405541632, -21.78219314458176825 ) ) ;
#51732=VECTOR ( 'NONE', #80173, 1000.000000000000000 ) ;
#51739=FACE_OUTER_BOUND ( 'NONE', #10505, .T. ) ;
#51740=CARTESIAN_POINT ( 'NONE',  ( 107.9747653995834753, -121.2541776101292186, -11.78219314458148226 ) ) ;
#51752=EDGE_CURVE ( 'NONE', #19525, #20491, #24621, .T. ) ;
#51754=EDGE_LOOP ( 'NONE', ( #1708, #30942, #34088, #28639, #68378, #76245 ) ) ;
#51760=DIRECTION ( 'NONE',  ( 3.100000000000000258E-29, -3.100000000000000044E-14, -1.000000000000000000 ) ) ;
#51767=CARTESIAN_POINT ( 'NONE',  ( 96.67439905703393777, -115.7784471599421323, -21.78219314458165812 ) ) ;
#51790=EDGE_LOOP ( 'NONE', ( #15620, #70756, #108, #10725 ) ) ;
#51802=CYLINDRICAL_SURFACE ( 'NONE', #26122, 2.000000000000007550 ) ;
#51807=VERTEX_POINT ( 'NONE', #79606 ) ;
#51812=PLANE ( 'NONE',  #2634 ) ;
#51825=CARTESIAN_POINT ( 'NONE',  ( 70.06670390244707392, -140.6784471599409869, 228.4678068554179902 ) ) ;
#51843=EDGE_CURVE ( 'NONE', #68139, #4100, #19156, .T. ) ;
#51850=PLANE ( 'NONE',  #29131 ) ;
#51854=PLANE ( 'NONE',  #43675 ) ;
#51855=ORIENTED_EDGE ( 'NONE', *, *, #50512, .F. ) ;
#51860=DIRECTION ( 'NONE',  ( -0.000000000000000000, -0.000000000000000000, 1.000000000000000000 ) ) ;
#51861=CARTESIAN_POINT ( 'NONE',  ( 68.92834633064059346, -139.0720971569717221, 246.7691504559092550 ) ) ;
#51886=CARTESIAN_POINT ( 'NONE',  ( 107.0667039024470313, -104.2784471599420755, -19.78219314458201694 ) ) ;
#51888=CARTESIAN_POINT ( 'NONE',  ( 146.3607517370862752, -137.9410632998380208, 246.8967281812609826 ) ) ;
#51897=ADVANCED_FACE ( 'NONE', ( #11897 ), #66901, .F. ) ;
#51913=CARTESIAN_POINT ( 'NONE',  ( 127.4144167604540030, -85.80981773760922238, 250.2201230397200220 ) ) ;
#51919=FACE_OUTER_BOUND ( 'NONE', #39331, .T. ) ;
#51923=VERTEX_POINT ( 'NONE', #55878 ) ;
#51932=DIRECTION ( 'NONE',  ( 0.000000000000000000, 0.000000000000000000, -1.000000000000000000 ) ) ;
#51934=CIRCLE ( 'NONE', #66409, 3.999999999999992895 ) ;
#51948=DIRECTION ( 'NONE',  ( 0.000000000000000000, 0.000000000000000000, -1.000000000000000000 ) ) ;
#51963=DIRECTION ( 'NONE',  ( 3.100000000000000258E-29, -3.100000000000000044E-14, -1.000000000000000000 ) ) ;
#51964=CARTESIAN_POINT ( 'NONE',  ( 144.0637245237351749, -140.6784087391956746, 245.5331728883010101 ) ) ;
#51965=DIRECTION ( 'NONE',  ( 1.000000000000000000, 0.000000000000000000, 0.000000000000000000 ) ) ;
#51968=DIRECTION ( 'NONE',  ( 0.000000000000000000, 0.000000000000000000, 1.000000000000000000 ) ) ;
#52007=CARTESIAN_POINT ( 'NONE',  ( 78.56670390244701707, -90.27844715994098124, 45.21780685541799727 ) ) ;
#52022=DIRECTION ( 'NONE',  ( 0.000000000000000000, 0.000000000000000000, -1.000000000000000000 ) ) ;
#52041=FACE_OUTER_BOUND ( 'NONE', #42668, .T. ) ;
#52060=LINE ( 'NONE', #11192, #60715 ) ;
#52075=CARTESIAN_POINT ( 'NONE',  ( 86.72755763596096301, -122.7870702624433648, 250.2178068554179902 ) ) ;
#52079=CARTESIAN_POINT ( 'NONE',  ( 116.0667039024470739, -137.6784471599409301, 222.2178068554179902 ) ) ;
#52113=EDGE_CURVE ( 'NONE', #20491, #60190, #58577, .T. ) ;
#52144=CARTESIAN_POINT ( 'NONE',  ( 131.8431396993165947, -68.25097877586425454, 247.0389312302800136 ) ) ;
#52152=ORIENTED_EDGE ( 'NONE', *, *, #28129, .T. ) ;
#52158=CARTESIAN_POINT ( 'NONE',  ( 147.0665874381622018, -67.87844715994090450, 245.5130140176639770 ) ) ;
#52163=VECTOR ( 'NONE', #4317, 1000.000000000000000 ) ;
#52166=EDGE_LOOP ( 'NONE', ( #80856, #67056, #29176, #76204, #13389, #79156 ) ) ;
#52215=EDGE_CURVE ( 'NONE', #33892, #75678, #9941, .T. ) ;
#52217=ORIENTED_EDGE ( 'NONE', *, *, #64878, .T. ) ;
#52220=EDGE_CURVE ( 'NONE', #51113, #86385, #14482, .T. ) ;
#52231=AXIS2_PLACEMENT_3D ( 'NONE', #81840, #60925, #62719 ) ;
#52232=CARTESIAN_POINT ( 'NONE',  ( 91.91441891875203396, -96.57077177933005885, -19.18411693322927292 ) ) ;
#52240=EDGE_CURVE ( 'NONE', #74190, #68597, #72388, .T. ) ;
#52244=ORIENTED_EDGE ( 'NONE', *, *, #61301, .T. ) ;
#52245=CARTESIAN_POINT ( 'NONE',  ( 107.0667039024470171, -79.67844715994094429, 138.7178068554180186 ) ) ;
#52247=PLANE ( 'NONE',  #40380 ) ;
#52265=VECTOR ( 'NONE', #45768, 1000.000000000000000 ) ;
#52279=DIRECTION ( 'NONE',  ( -3.100000000000000258E-29, 3.100000000000000044E-14, 1.000000000000000000 ) ) ;
#52284=ORIENTED_EDGE ( 'NONE', *, *, #36276, .T. ) ;
#52323=CIRCLE ( 'NONE', #63987, 3.000000000000002665 ) ;
#52336=DIRECTION ( 'NONE',  ( -1.000000000000000078E-15, 1.000000000000000000, 0.000000000000000000 ) ) ;
#52338=FACE_OUTER_BOUND ( 'NONE', #38140, .T. ) ;
#52349=AXIS2_PLACEMENT_3D ( 'NONE', #1226, #14409, #77081 ) ;
#52350=CARTESIAN_POINT ( 'NONE',  ( 139.3215235511330263, -74.97943253980591294, 248.4067532124560103 ) ) ;
#52351=CARTESIAN_POINT ( 'NONE',  ( 147.0528210869385077, -67.88961359424753539, 245.7502281596648288 ) ) ;
#52354=DIRECTION ( 'NONE',  ( -1.000000000000000078E-15, 1.000000000000000000, 0.000000000000000000 ) ) ;
#52378=EDGE_CURVE ( 'NONE', #11503, #20018, #22646, .T. ) ;
#52397=CARTESIAN_POINT ( 'NONE',  ( 144.0179926818975673, -140.6397677690979151, 245.9888717887127427 ) ) ;
#52407=LINE ( 'NONE', #17922, #51732 ) ;
#52446=LINE ( 'NONE', #80209, #74718 ) ;
#52450=PLANE ( 'NONE',  #16161 ) ;
#52457=EDGE_CURVE ( 'NONE', #42555, #40469, #82088, .T. ) ;
#52465=CARTESIAN_POINT ( 'NONE',  ( 80.34435516212752759, -110.9887994459054994, 250.2178068554180470 ) ) ;
#52491=DIRECTION ( 'NONE',  ( 1.000000000000000000, 1.000000000000000078E-15, 0.000000000000000000 ) ) ;
#52499=CARTESIAN_POINT ( 'NONE',  ( 147.0667039024470171, -101.1152277505316164, 245.7200377504910023 ) ) ;
#52500=CARTESIAN_POINT ( 'NONE',  ( 91.91441891875203396, -96.57077177933005885, -19.18411693322927292 ) ) ;
#52517=CARTESIAN_POINT ( 'NONE',  ( 116.0667039024470313, -104.2784471599411091, 2.217806855418003043 ) ) ;
#52525=VERTEX_POINT ( 'NONE', #28900 ) ;
#52533=DIRECTION ( 'NONE',  ( -1.000000000000000078E-15, 1.000000000000000000, 0.000000000000000000 ) ) ;
#52590=EDGE_CURVE ( 'NONE', #17172, #84388, #79395, .T. ) ;
#52599=CARTESIAN_POINT ( 'NONE',  ( 67.06681736700808472, -67.87844715931913697, 245.5130139978070076 ) ) ;
#52605=ORIENTED_EDGE ( 'NONE', *, *, #6176, .F. ) ;
#52606=AXIS2_PLACEMENT_3D ( 'NONE', #5416, #26736, #81733 ) ;
#52607=FACE_OUTER_BOUND ( 'NONE', #89402, .T. ) ;
#52608=DIRECTION ( 'NONE',  ( -1.000000000000000000, -1.000000000000000078E-15, 0.000000000000000000 ) ) ;
#52612=EDGE_CURVE ( 'NONE', #25238, #30354, #19914, .T. ) ;
#52629=ORIENTED_EDGE ( 'NONE', *, *, #37801, .T. ) ;
#52643=CARTESIAN_POINT ( 'NONE',  ( 91.91441891875204817, -111.9861225405540637, -19.18411693322877198 ) ) ;
#52644=ORIENTED_EDGE ( 'NONE', *, *, #51410, .T. ) ;
#52667=ORIENTED_EDGE ( 'NONE', *, *, #69463, .T. ) ;
#52691=EDGE_LOOP ( 'NONE', ( #66607, #62848, #59155, #82351, #57086, #59218, #2921, #30215, #14610, #34466 ) ) ;
#52731=CARTESIAN_POINT ( 'NONE',  ( 107.5667039024470313, -108.2470741265389620, -19.78219314458190681 ) ) ;
#52735=VECTOR ( 'NONE', #77703, 999.9999999999998863 ) ;
#52736=FACE_OUTER_BOUND ( 'NONE', #87399, .T. ) ;
#52738=CARTESIAN_POINT ( 'NONE',  ( 107.0667039024470313, -104.2784471599418197, -11.78219314458200984 ) ) ;
#52753=EDGE_LOOP ( 'NONE', ( #55824, #52217, #76394, #8414 ) ) ;
#52755=EDGE_LOOP ( 'NONE', ( #78564, #38417, #23686, #4139 ) ) ;
#52759=VECTOR ( 'NONE', #72495, 1000.000000000000000 ) ;
#52761=CARTESIAN_POINT ( 'NONE',  ( 107.0667039024470313, -104.2784471599420471, -19.18411693322902423 ) ) ;
#52763=CARTESIAN_POINT ( 'NONE',  ( 161.0667039024470171, -78.67844715994088745, 96.96780685541800437 ) ) ;
#52772=CARTESIAN_POINT ( 'NONE',  ( 111.3555650440039528, -119.3022720253470226, -11.78219314458153733 ) ) ;
#52818=CONICAL_SURFACE ( 'NONE', #60108, 24.50000000000000711, 0.7419472680059182590 ) ;
#52825=VERTEX_POINT ( 'NONE', #80182 ) ;
#52834=CARTESIAN_POINT ( 'NONE',  ( 74.06670390244704549, -118.2784471599409812, 51.21780685541800437 ) ) ;
#52835=LINE ( 'NONE', #11096, #76649 ) ;
#52836=DIRECTION ( 'NONE',  ( 0.000000000000000000, 0.000000000000000000, 1.000000000000000000 ) ) ;
#52844=DIRECTION ( 'NONE',  ( -1.000000000000000000, -1.206764157201257538E-15, 0.000000000000000000 ) ) ;
#52869=CARTESIAN_POINT ( 'NONE',  ( 106.5667039024470455, -113.7784471599420613, -19.78219314458171141 ) ) ;
#52890=ORIENTED_EDGE ( 'NONE', *, *, #69690, .T. ) ;
#52917=EDGE_LOOP ( 'NONE', ( #22585, #3289, #65553, #48102, #84010, #26704 ) ) ;
#52926=CARTESIAN_POINT ( 'NONE',  ( 103.8797721312301547, -106.6957733451327215, -19.78219314458193168 ) ) ;
#52929=CARTESIAN_POINT ( 'NONE',  ( 115.0667039024470313, -104.2784471599420897, -19.78219314458201694 ) ) ;
#52933=ORIENTED_EDGE ( 'NONE', *, *, #86409, .T. ) ;
#52936=ORIENTED_EDGE ( 'NONE', *, *, #5499, .T. ) ;
#52958=EDGE_CURVE ( 'NONE', #17260, #65590, #88993, .T. ) ;
#52974=ORIENTED_EDGE ( 'NONE', *, *, #72767, .F. ) ;
#52976=VERTEX_POINT ( 'NONE', #88338 ) ;
#52979=CYLINDRICAL_SURFACE ( 'NONE', #26252, 32.50000000000001421 ) ;
#52982=CARTESIAN_POINT ( 'NONE',  ( 77.11671781838086304, -140.6784471615123664, 245.5822703020409961 ) ) ;
#52995=CARTESIAN_POINT ( 'NONE',  ( 122.2189888861420286, -96.57077177933004464, -19.18411693322927292 ) ) ;
#52998=DIRECTION ( 'NONE',  ( -1.000000000000000000, -1.206764157201257538E-15, 0.000000000000000000 ) ) ;
#53013=EDGE_CURVE ( 'NONE', #54044, #19525, #67194, .T. ) ;
#53019=EDGE_CURVE ( 'NONE', #88126, #33837, #47408, .T. ) ;
#53034=ORIENTED_EDGE ( 'NONE', *, *, #87828, .T. ) ;
#53037=CARTESIAN_POINT ( 'NONE',  ( 107.0667039024469886, -67.87844715994094713, 173.2178068554179902 ) ) ;
#53051=DIRECTION ( 'NONE',  ( -1.000000000000000078E-15, 1.000000000000000000, 0.000000000000000000 ) ) ;
#53064=ORIENTED_EDGE ( 'NONE', *, *, #922, .F. ) ;
#53088=CARTESIAN_POINT ( 'NONE',  ( 74.06670390244704549, -118.2784471599409812, 222.2178068554179902 ) ) ;
#53089=B_SPLINE_SURFACE_WITH_KNOTS ( 'NONE', 3, 3, ( 
 ( #16286, #21089, #80745, #34707 ),
 ( #53894, #83319, #76497, #73464 ),
 ( #88461, #45734, #18502, #12598 ),
 ( #74821, #4882, #66651, #66193 ),
 ( #4439, #32127, #11702, #32574 ) ),
 .UNSPECIFIED., .F., .F., .F.,
 ( 4, 1, 4 ),
 ( 4, 4 ),
 ( 0.000000000000000000, 0.5714285714285709528, 1.000000000000000000 ),
 ( 0.1481392554759810021, 0.3635576785635249997 ),
 .UNSPECIFIED. ) ;
#53098=ORIENTED_EDGE ( 'NONE', *, *, #86717, .F. ) ;
#53106=CARTESIAN_POINT ( 'NONE',  ( 107.0667039024470313, -104.2784471599413934, 2.217806855418003043 ) ) ;
#53126=VERTEX_POINT ( 'NONE', #10462 ) ;
#53135=VECTOR ( 'NONE', #37449, 1000.000000000000000 ) ;
#53151=LINE ( 'NONE', #46348, #73211 ) ;
#53168=DIRECTION ( 'NONE',  ( 3.100000000000000258E-29, -3.100000000000000044E-14, -1.000000000000000000 ) ) ;
#53176=DIRECTION ( 'NONE',  ( -1.000000000000000078E-15, 1.000000000000000000, 0.000000000000000000 ) ) ;
#53180=EDGE_CURVE ( 'NONE', #86096, #69445, #45841, .T. ) ;
#53194=LINE ( 'NONE', #24196, #73598 ) ;
#53195=CARTESIAN_POINT ( 'NONE',  ( 146.6849323694283669, -124.3898625509450966, 247.0153898053430055 ) ) ;
#53205=CARTESIAN_POINT ( 'NONE',  ( 144.5245849510534697, -140.2205661113345911, 245.5201220521130097 ) ) ;
#53252=ORIENTED_EDGE ( 'NONE', *, *, #70817, .F. ) ;
#53275=ORIENTED_EDGE ( 'NONE', *, *, #2106, .F. ) ;
#53307=DIRECTION ( 'NONE',  ( 0.000000000000000000, 0.000000000000000000, 1.000000000000000000 ) ) ;
#53319=CARTESIAN_POINT ( 'NONE',  ( 70.06670390244707392, -137.6784471599409869, 55.21780685541800437 ) ) ;
#53321=CARTESIAN_POINT ( 'NONE',  ( 59.56670390244699576, -67.87844715994098976, 190.2178068554179902 ) ) ;
#53351=DIRECTION ( 'NONE',  ( -1.000000000000000078E-15, 1.000000000000000000, 0.000000000000000000 ) ) ;
#53354=ADVANCED_FACE ( 'NONE', ( #25422 ), #4984, .T. ) ;
#53380=VERTEX_POINT ( 'NONE', #53547 ) ;
#53391=EDGE_LOOP ( 'NONE', ( #57620, #6419, #77402, #22694, #25867 ) ) ;
#53427=DIRECTION ( 'NONE',  ( 1.000000000000000000, 1.000000000000000078E-15, 0.000000000000000000 ) ) ;
#53438=DIRECTION ( 'NONE',  ( 1.000000000000000078E-15, -1.000000000000000000, 0.000000000000000000 ) ) ;
#53457=EDGE_CURVE ( 'NONE', #14490, #58962, #33807, .T. ) ;
#53461=DIRECTION ( 'NONE',  ( -3.100000000000000258E-29, 3.100000000000000044E-14, 1.000000000000000000 ) ) ;
#53466=CARTESIAN_POINT ( 'NONE',  ( 158.0667039024470171, -79.67844715994088745, 85.21780685541799016 ) ) ;
#53470=EDGE_CURVE ( 'NONE', #37134, #30354, #48361, .T. ) ;
#53484=CARTESIAN_POINT ( 'NONE',  ( 131.8479104382178946, -69.08669111203026603, 247.4970909970599848 ) ) ;
#53489=ORIENTED_EDGE ( 'NONE', *, *, #6176, .T. ) ;
#53494=DIRECTION ( 'NONE',  ( -0.8660254037844392627, 0.4999999999999990008, -1.549999999999999706E-14 ) ) ;
#53503=DIRECTION ( 'NONE',  ( 0.000000000000000000, 0.000000000000000000, -1.000000000000000000 ) ) ;
#53507=DIRECTION ( 'NONE',  ( 1.000000000000000078E-15, -1.000000000000000000, 0.000000000000000000 ) ) ;
#53515=DIRECTION ( 'NONE',  ( 0.8660254037844392627, -0.4999999999999990008, 1.549999999999999706E-14 ) ) ;
#53535=VECTOR ( 'NONE', #62672, 1000.000000000000000 ) ;
#53536=EDGE_CURVE ( 'NONE', #40328, #43983, #405, .T. ) ;
#53541=ORIENTED_EDGE ( 'NONE', *, *, #58975, .T. ) ;
#53543=EDGE_CURVE ( 'NONE', #86794, #83222, #75955, .T. ) ;
#53547=CARTESIAN_POINT ( 'NONE',  ( 158.0667039024470171, -79.67844715994088745, 120.2178068554179902 ) ) ;
#53564=CARTESIAN_POINT ( 'NONE',  ( 147.0667039024469886, -67.87844716047348470, 245.4920193514540188 ) ) ;
#53573=LINE ( 'NONE', #39073, #50190 ) ;
#53590=DIRECTION ( 'NONE',  ( 1.000000000000000000, 8.953411488912556626E-16, 0.000000000000000000 ) ) ;
#53606=DIRECTION ( 'NONE',  ( 7.076552332833900719E-16, -1.000000000000000000, 3.100000000000000044E-14 ) ) ;
#53607=DIRECTION ( 'NONE',  ( 0.000000000000000000, 0.000000000000000000, 1.000000000000000000 ) ) ;
#53610=LINE ( 'NONE', #19123, #21820 ) ;
#53622=FACE_OUTER_BOUND ( 'NONE', #60101, .T. ) ;
#53626=CARTESIAN_POINT ( 'NONE',  ( 107.0667039024470029, -74.77844715994095282, 25.71780685541800437 ) ) ;
#53631=ORIENTED_EDGE ( 'NONE', *, *, #36586, .T. ) ;
#53637=ORIENTED_EDGE ( 'NONE', *, *, #20357, .F. ) ;
#53644=DIRECTION ( 'NONE',  ( -1.000000000000000000, -8.163404592832032979E-16, 0.000000000000000000 ) ) ;
#53645=ADVANCED_FACE ( 'NONE', ( #86218 ), #9461, .T. ) ;
#53650=CARTESIAN_POINT ( 'NONE',  ( 145.7688716652828873, -137.6858083443213161, 247.4233469738189797 ) ) ;
#53662=ORIENTED_EDGE ( 'NONE', *, *, #18937, .F. ) ;
#53676=CYLINDRICAL_SURFACE ( 'NONE', #21098, 3.999999999999992895 ) ;
#53685=LINE ( 'NONE', #33725, #1435 ) ;
#53690=DIRECTION ( 'NONE',  ( -3.100000000000000258E-29, 3.100000000000000044E-14, 1.000000000000000000 ) ) ;
#53702=FACE_OUTER_BOUND ( 'NONE', #11057, .T. ) ;
#53709=CARTESIAN_POINT ( 'NONE',  ( 121.3140869715381456, -113.5527167097541508, -11.78219314458173272 ) ) ;
#53715=DIRECTION ( 'NONE',  ( -0.8660254037844389297, 0.4999999999999993894, -1.550000000000000968E-14 ) ) ;
#53716=VERTEX_POINT ( 'NONE', #39830 ) ;
#53717=EDGE_CURVE ( 'NONE', #45547, #63478, #33920, .T. ) ;
#53721=CIRCLE ( 'NONE', #14609, 15.50000000000000000 ) ;
#53722=ORIENTED_EDGE ( 'NONE', *, *, #24527, .T. ) ;
#53726=ORIENTED_EDGE ( 'NONE', *, *, #55739, .F. ) ;
#53746=EDGE_CURVE ( 'NONE', #38959, #71019, #62961, .T. ) ;
#53750=EDGE_CURVE ( 'NONE', #52976, #52525, #18496, .T. ) ;
#53752=AXIS2_PLACEMENT_3D ( 'NONE', #81038, #59212, #11066 ) ;
#53758=DIRECTION ( 'NONE',  ( -0.8660254037844381525, -0.5000000000000007772, 1.549999999999999706E-14 ) ) ;
#53770=PLANE ( 'NONE',  #89119 ) ;
#53775=ORIENTED_EDGE ( 'NONE', *, *, #17599, .T. ) ;
#53777=ADVANCED_FACE ( 'NONE', ( #73919 ), #12541, .F. ) ;
#53780=ORIENTED_EDGE ( 'NONE', *, *, #30139, .T. ) ;
#53787=CARTESIAN_POINT ( 'NONE',  ( 107.0667039024470313, -104.2784471599413934, 2.217806855418003043 ) ) ;
#53793=CARTESIAN_POINT ( 'NONE',  ( 145.3595637443018234, -69.45303146431501773, 247.4784022495120155 ) ) ;
#53795=DIRECTION ( 'NONE',  ( -3.100000000000000258E-29, 3.100000000000000044E-14, 1.000000000000000000 ) ) ;
#53801=CARTESIAN_POINT ( 'NONE',  ( 67.06723304023354615, -67.87844715994098976, 245.5215440408323104 ) ) ;
#53828=ADVANCED_FACE ( 'NONE', ( #28916 ), #48418, .T. ) ;
#53831=ORIENTED_EDGE ( 'NONE', *, *, #31285, .F. ) ;
#53842=ORIENTED_EDGE ( 'NONE', *, *, #34908, .F. ) ;
#53847=AXIS2_PLACEMENT_3D ( 'NONE', #10661, #2534, #72896 ) ;
#53869=CARTESIAN_POINT ( 'NONE',  ( 98.58946256649487339, -99.96145986183429955, -19.78219314458215550 ) ) ;
#53884=EDGE_LOOP ( 'NONE', ( #69957, #68064, #35380, #35391 ) ) ;
#53890=EDGE_CURVE ( 'NONE', #46794, #69984, #77065, .T. ) ;
#53892=CARTESIAN_POINT ( 'NONE',  ( 145.4284892259529727, -139.2918928890854886, 245.9245030021744753 ) ) ;
#53894=CARTESIAN_POINT ( 'NONE',  ( 71.07979490493546848, -139.9914422477621656, 247.3423811826519909 ) ) ;
#53898=ORIENTED_EDGE ( 'NONE', *, *, #27108, .T. ) ;
#53948=CARTESIAN_POINT ( 'NONE',  ( 107.0667039024470313, -104.2784471599420755, -19.78219314458201694 ) ) ;
#53975=DIRECTION ( 'NONE',  ( -3.100000000000000258E-29, 3.100000000000000044E-14, 1.000000000000000000 ) ) ;
#54024=CARTESIAN_POINT ( 'NONE',  ( 74.06670390244704549, -118.2784471599409812, 230.7030882296565721 ) ) ;
#54031=DIRECTION ( 'NONE',  ( 0.7071067811869833353, 0.7071067811861116992, -5.678536605557180514E-12 ) ) ;
#54044=VERTEX_POINT ( 'NONE', #27559 ) ;
#54047=ORIENTED_EDGE ( 'NONE', *, *, #27740, .F. ) ;
#54052=LINE ( 'NONE', #45456, #45094 ) ;
#54061=CARTESIAN_POINT ( 'NONE',  ( 82.56670390244703128, -104.2784471599409670, 22.21780685541800082 ) ) ;
#54063=ORIENTED_EDGE ( 'NONE', *, *, #18, .T. ) ;
#54065=EDGE_CURVE ( 'NONE', #37203, #34061, #72036, .T. ) ;
#54067=ORIENTED_EDGE ( 'NONE', *, *, #5816, .F. ) ;
#54069=LINE ( 'NONE', #54517, #86129 ) ;
#54094=DIRECTION ( 'NONE',  ( 1.000000000000000000, 0.000000000000000000, 0.000000000000000000 ) ) ;
#54101=CARTESIAN_POINT ( 'NONE',  ( 147.0667039024470455, -124.3811837900075972, 245.5761017658709875 ) ) ;
#54132=DIRECTION ( 'NONE',  ( 1.000000000000000000, 1.000000000000000078E-15, 0.000000000000000000 ) ) ;
#54134=DIRECTION ( 'NONE',  ( 1.000000000000000000, 1.276118419109374860E-15, 0.000000000000000000 ) ) ;
#54143=CARTESIAN_POINT ( 'NONE',  ( 143.5667039024469886, -67.87844715994090450, 55.21780685541800437 ) ) ;
#54152=ADVANCED_FACE ( 'NONE', ( #22555 ), #51124, .F. ) ;
#54180=LINE ( 'NONE', #11993, #89856 ) ;
#54182=ADVANCED_FACE ( 'NONE', ( #32913 ), #25205, .T. ) ;
#54218=VERTEX_POINT ( 'NONE', #40628 ) ;
#54219=VERTEX_POINT ( 'NONE', #18389 ) ;
#54235=CARTESIAN_POINT ( 'NONE',  ( 145.4167568336388001, -78.89489531512775500, 247.5190035850939125 ) ) ;
#54238=AXIS2_PLACEMENT_3D ( 'NONE', #85530, #16464, #2394 ) ;
#54272=B_SPLINE_CURVE_WITH_KNOTS ( 'NONE', 3,
 ( #26215, #55676, #5785, #53892, #55242, #33921, #20748, #75273, #33475, #81653, #82994, #61179, #74818, #76157, #27115, #48419, #46639, #61618, #13936, #41614, #33026, #69351, #89354, #12596, #34819, #28001, #62529, #74372, #12144, #39831 ),
 .UNSPECIFIED., .F., .F.,
 ( 4, 2, 2, 2, 1, 1, 1, 1, 1, 2, 2, 2, 2, 1, 1, 1, 2, 2, 4 ),
 ( 0.000000000000000000, 0.1250000000002037537, 0.1406250000002256251, 0.1484375000002365330, 0.1562500000002474687, 0.1875000000002649825, 0.2187500000002825240, 0.2343750000002711997, 0.2421875000002656209, 0.2460937500002628453, 0.2500000000002600142, 0.3749999999996757039, 0.4374999999993836042, 0.4687499999992374988, 0.4843749999991791566, 0.4921874999991500133, 0.4960937499991504018, 0.4999999999991508459, 1.000000000000000000 ),
 .UNSPECIFIED. ) ;
#54294=VERTEX_POINT ( 'NONE', #73357 ) ;
#54311=CARTESIAN_POINT ( 'NONE',  ( 106.1586424053105873, -87.30271670975442078, -11.78219314458253741 ) ) ;
#54319=EDGE_CURVE ( 'NONE', #54218, #69445, #42485, .T. ) ;
#54337=CARTESIAN_POINT ( 'NONE',  ( 70.05650175495836152, -139.5326789363696776, 247.4193337233699879 ) ) ;
#54343=EDGE_LOOP ( 'NONE', ( #56520, #73898, #88150, #61893 ) ) ;
#54348=AXIS2_PLACEMENT_3D ( 'NONE', #9770, #4738, #25167 ) ;
#54377=DIRECTION ( 'NONE',  ( -1.000000000000000000, -9.999999999999862726E-16, 4.440892098500630106E-16 ) ) ;
#54402=VERTEX_POINT ( 'NONE', #13823 ) ;
#54404=CARTESIAN_POINT ( 'NONE',  ( 154.5667039024469886, -67.87844715994090450, 155.2178068554179902 ) ) ;
#54489=DIRECTION ( 'NONE',  ( 0.000000000000000000, 0.000000000000000000, 1.000000000000000000 ) ) ;
#54509=ORIENTED_EDGE ( 'NONE', *, *, #1907, .T. ) ;
#54510=VERTEX_POINT ( 'NONE', #42846 ) ;
#54513=CARTESIAN_POINT ( 'NONE',  ( 74.06670390244704549, -118.2784471599409812, 51.21780685541800437 ) ) ;
#54517=CARTESIAN_POINT ( 'NONE',  ( 54.06670390244700997, -79.67844715994098692, 180.4678068554179902 ) ) ;
#54531=CARTESIAN_POINT ( 'NONE',  ( 133.5122728224967830, -134.8238870115027055, 248.4142799812389910 ) ) ;
#54540=CARTESIAN_POINT ( 'NONE',  ( 90.06670420047028358, -137.6784471599409585, 55.21780685541800437 ) ) ;
#54566=DIRECTION ( 'NONE',  ( 0.000000000000000000, 0.000000000000000000, -1.000000000000000000 ) ) ;
#54570=ORIENTED_EDGE ( 'NONE', *, *, #30789, .F. ) ;
#54572=VECTOR ( 'NONE', #71890, 1000.000000000000000 ) ;
#54599=ORIENTED_EDGE ( 'NONE', *, *, #44628, .T. ) ;
#54600=EDGE_CURVE ( 'NONE', #2833, #60027, #77850, .T. ) ;
#54609=ORIENTED_EDGE ( 'NONE', *, *, #69091, .F. ) ;
#54615=VECTOR ( 'NONE', #84877, 1000.000000000000000 ) ;
#54644=DIRECTION ( 'NONE',  ( 1.000000000000000000, 8.953411488912556626E-16, 0.000000000000000000 ) ) ;
#54645=PLANE ( 'NONE',  #399 ) ;
#54671=FACE_OUTER_BOUND ( 'NONE', #21955, .T. ) ;
#54685=EDGE_LOOP ( 'NONE', ( #63768, #13324, #50385, #39070, #51473, #79710 ) ) ;
#54689=CARTESIAN_POINT ( 'NONE',  ( 70.06670390441306040, -140.6784471619069734, 245.4415720117440003 ) ) ;
#54692=CARTESIAN_POINT ( 'NONE',  ( 116.0667039024470313, -104.2784471599411091, 19.21780685541799016 ) ) ;
#54713=FACE_OUTER_BOUND ( 'NONE', #39954, .T. ) ;
#54715=ORIENTED_EDGE ( 'NONE', *, *, #57133, .F. ) ;
#54723=AXIS2_PLACEMENT_3D ( 'NONE', #68069, #47153, #25840 ) ;
#54736=DIRECTION ( 'NONE',  ( -0.7349399772593249169, -0.6687953793059874252, 0.1121426343770439288 ) ) ;
#54781=EDGE_CURVE ( 'NONE', #9096, #56828, #25117, .T. ) ;
#54797=ORIENTED_EDGE ( 'NONE', *, *, #48383, .F. ) ;
#54830=CONICAL_SURFACE ( 'NONE', #60621, 16.25000000000000000, 0.5235987755982992597 ) ;
#54853=CARTESIAN_POINT ( 'NONE',  ( 111.8298436232616240, -89.52844715994213232, -21.78219314458246103 ) ) ;
#54856=FACE_OUTER_BOUND ( 'NONE', #37670, .T. ) ;
#54857=DIRECTION ( 'NONE',  ( -1.087812297297669405E-15, 1.000000000000000000, -3.100000000000000044E-14 ) ) ;
#54869=DIRECTION ( 'NONE',  ( 0.1250000000000000278, 0.9921567416492215186, -3.035766082959410522E-14 ) ) ;
#54870=ORIENTED_EDGE ( 'NONE', *, *, #89868, .T. ) ;
#54879=DIRECTION ( 'NONE',  ( 0.000000000000000000, 0.000000000000000000, -1.000000000000000000 ) ) ;
#54907=AXIS2_PLACEMENT_3D ( 'NONE', #80539, #45981, #73714 ) ;
#54916=FACE_OUTER_BOUND ( 'NONE', #9169, .T. ) ;
#54957=CIRCLE ( 'NONE', #62249, 32.50000000000000711 ) ;
#54959=ADVANCED_FACE ( 'NONE', ( #29578, #85467 ), #15515, .T. ) ;
#54974=CARTESIAN_POINT ( 'NONE',  ( 127.0667052882549797, -71.37844715994091871, 222.2178068554179902 ) ) ;
#54982=FILL_AREA_STYLE_COLOUR ( '', #8667 ) ;
#54998=DIRECTION ( 'NONE',  ( 1.000000000000000078E-15, -1.000000000000000000, 0.000000000000000000 ) ) ;
#55020=ORIENTED_EDGE ( 'NONE', *, *, #29907, .T. ) ;
#55021=AXIS2_PLACEMENT_3D ( 'NONE', #5863, #83069, #61250 ) ;
#55033=DIRECTION ( 'NONE',  ( 3.100000000000000258E-29, -3.100000000000000044E-14, -1.000000000000000000 ) ) ;
#55038=VERTEX_POINT ( 'NONE', #36843 ) ;
#55066=ORIENTED_EDGE ( 'NONE', *, *, #79635, .T. ) ;
#55079=AXIS2_PLACEMENT_3D ( 'NONE', #43709, #15583, #70997 ) ;
#55090=B_SPLINE_CURVE_WITH_KNOTS ( 'NONE', 3,
 ( #62749, #50009, #29580, #50458, #36409, #42738, #525, #63658, #22783, #83216, #981, #63204, #8708, #56374, #20981, #7794, #84114, #14165 ),
 .UNSPECIFIED., .F., .F.,
 ( 4, 2, 2, 2, 2, 2, 2, 2, 4 ),
 ( 0.000000000000000000, 0.1250000000000000000, 0.2500000000000000000, 0.3750000000000000000, 0.5000000000000000000, 0.6250000000000000000, 0.7500000000000000000, 0.8750000000000000000, 1.000000000000000000 ),
 .UNSPECIFIED. ) ;
#55101=DIRECTION ( 'NONE',  ( -0.5000000000000008882, 0.8660254037844382635, -2.684678751731760294E-14 ) ) ;
#55102=CARTESIAN_POINT ( 'NONE',  ( 107.0667039024469886, -67.87844715994094713, 93.21780685541800437 ) ) ;
#55130=AXIS2_PLACEMENT_3D ( 'NONE', #22348, #17316, #15982 ) ;
#55136=FACE_OUTER_BOUND ( 'NONE', #41214, .T. ) ;
#55140=CARTESIAN_POINT ( 'NONE',  ( 144.0667039024470739, -140.6784471599409017, 55.21780685541800437 ) ) ;
#55141=CARTESIAN_POINT ( 'NONE',  ( 67.06928294555038406, -67.88014341905780213, 245.5936337082227681 ) ) ;
#55171=ORIENTED_EDGE ( 'NONE', *, *, #20397, .T. ) ;
#55172=ORIENTED_EDGE ( 'NONE', *, *, #15660, .F. ) ;
#55202=DIRECTION ( 'NONE',  ( 0.000000000000000000, 0.000000000000000000, -1.000000000000000000 ) ) ;
#55203=DIRECTION ( 'NONE',  ( -3.100000000000000258E-29, 3.100000000000000044E-14, 1.000000000000000000 ) ) ;
#55208=LINE ( 'NONE', #13907, #45424 ) ;
#55242=CARTESIAN_POINT ( 'NONE',  ( 145.4263377285063257, -139.2898755805769326, 245.9459212860521404 ) ) ;
#55249=ORIENTED_EDGE ( 'NONE', *, *, #28247, .T. ) ;
#55260=FACE_OUTER_BOUND ( 'NONE', #27956, .T. ) ;
#55267=DIRECTION ( 'NONE',  ( -0.5000000000000015543, 0.8660254037844377084, -2.602085213965216006E-14 ) ) ;
#55291=ORIENTED_EDGE ( 'NONE', *, *, #75557, .T. ) ;
#55294=CARTESIAN_POINT ( 'NONE',  ( 111.8298436232616240, -119.0284471599421181, -21.78219314458157285 ) ) ;
#55301=ADVANCED_FACE ( 'NONE', ( #36184 ), #83005, .T. ) ;
#55319=DIRECTION ( 'NONE',  ( 1.000000000000000000, 0.000000000000000000, 0.000000000000000000 ) ) ;
#55323=ORIENTED_EDGE ( 'NONE', *, *, #60881, .T. ) ;
#55330=CARTESIAN_POINT ( 'NONE',  ( 87.93968657577623560, -139.1807631652558825, 247.6215491605419174 ) ) ;
#55334=DIRECTION ( 'NONE',  ( -1.000000000000000000, -1.206764157201257538E-15, 0.000000000000000000 ) ) ;
#55343=CARTESIAN_POINT ( 'NONE',  ( 74.06670390244704549, -118.2784471599409812, 45.21780685541799727 ) ) ;
#55353=LINE ( 'NONE', #4211, #12275 ) ;
#55359=AXIS2_PLACEMENT_3D ( 'NONE', #36486, #76466, #76920 ) ;
#55361=EDGE_LOOP ( 'NONE', ( #83558, #72668, #89022, #78662, #35414, #88601 ) ) ;
#55368=EDGE_CURVE ( 'NONE', #13876, #54219, #78436, .T. ) ;
#55372=CARTESIAN_POINT ( 'NONE',  ( 110.0667047667142953, -70.87844715994094713, 93.21780685541800437 ) ) ;
#55409=ORIENTED_EDGE ( 'NONE', *, *, #19328, .F. ) ;
#55416=ADVANCED_FACE ( 'NONE', ( #8943 ), #58838, .F. ) ;
#55428=ORIENTED_EDGE ( 'NONE', *, *, #74250, .T. ) ;
#55431=ORIENTED_EDGE ( 'NONE', *, *, #48664, .T. ) ;
#55456=CARTESIAN_POINT ( 'NONE',  ( 133.9812285940911067, -95.46118927874373128, 250.2191008560389776 ) ) ;
#55467=CARTESIAN_POINT ( 'NONE',  ( 68.83135239564657581, -139.4430956531405172, 245.6798494796449859 ) ) ;
#55511=AXIS2_PLACEMENT_3D ( 'NONE', #46342, #40443, #39097 ) ;
#55537=CARTESIAN_POINT ( 'NONE',  ( 69.56670390244701707, -90.27844715994098124, 45.21780685541799727 ) ) ;
#55555=CARTESIAN_POINT ( 'NONE',  ( 121.9571836895285486, -124.7784471599409386, 222.2178068554179902 ) ) ;
#55561=EDGE_LOOP ( 'NONE', ( #89886, #55066 ) ) ;
#55568=CARTESIAN_POINT ( 'NONE',  ( 107.0667039024470313, -104.2784471599413934, 2.217806855418003043 ) ) ;
#55576=EDGE_LOOP ( 'NONE', ( #4981, #53831, #299 ) ) ;
#55577=AXIS2_PLACEMENT_3D ( 'NONE', #33524, #26698, #76656 ) ;
#55585=CARTESIAN_POINT ( 'NONE',  ( 90.06670390244703128, -104.2784471599417770, -9.937637710810031777 ) ) ;
#55593=EDGE_CURVE ( 'NONE', #68597, #67104, #44571, .T. ) ;
#55613=CARTESIAN_POINT ( 'NONE',  ( 106.5667039024470313, -106.2627606432404974, -19.78219314458196010 ) ) ;
#55615=EDGE_LOOP ( 'NONE', ( #43980, #25821, #59105, #15431, #7013 ) ) ;
#55635=VERTEX_POINT ( 'NONE', #87971 ) ;
#55636=ORIENTED_EDGE ( 'NONE', *, *, #87795, .F. ) ;
#55653=CARTESIAN_POINT ( 'NONE',  ( 146.4162810824392125, -137.3184838880133611, 246.9859360010804039 ) ) ;
#55664=CARTESIAN_POINT ( 'NONE',  ( 74.06670390244701707, -90.27844715994098124, 45.21780685541799727 ) ) ;
#55668=DIRECTION ( 'NONE',  ( -1.000000000000000078E-15, 1.000000000000000000, 0.000000000000000000 ) ) ;
#55672=ORIENTED_EDGE ( 'NONE', *, *, #66498, .T. ) ;
#55673=ORIENTED_EDGE ( 'NONE', *, *, #70207, .T. ) ;
#55676=CARTESIAN_POINT ( 'NONE',  ( 145.4417903158968670, -139.3033607457884102, 245.6608632105124173 ) ) ;
#55685=VECTOR ( 'NONE', #39885, 1000.000000000000000 ) ;
#55698=EDGE_CURVE ( 'NONE', #69445, #85102, #76019, .T. ) ;
#55710=ORIENTED_EDGE ( 'NONE', *, *, #8100, .F. ) ;
#55719=AXIS2_PLACEMENT_3D ( 'NONE', #734, #50221, #62519 ) ;
#55721=VERTEX_POINT ( 'NONE', #68424 ) ;
#55725=EDGE_LOOP ( 'NONE', ( #20532, #18452, #35785 ) ) ;
#55739=EDGE_CURVE ( 'NONE', #25814, #960, #22412, .T. ) ;
#55748=DIRECTION ( 'NONE',  ( 1.000000000000000078E-15, -1.000000000000000000, 0.000000000000000000 ) ) ;
#55749=DIRECTION ( 'NONE',  ( -3.100000000000000258E-29, 3.100000000000000044E-14, 1.000000000000000000 ) ) ;
#55759=VECTOR ( 'NONE', #47764, 999.9999999999998863 ) ;
#55776=ORIENTED_EDGE ( 'NONE', *, *, #51752, .T. ) ;
#55777=ORIENTED_EDGE ( 'NONE', *, *, #25255, .F. ) ;
#55811=VECTOR ( 'NONE', #71607, 1000.000000000000000 ) ;
#55822=ORIENTED_EDGE ( 'NONE', *, *, #41883, .T. ) ;
#55824=ORIENTED_EDGE ( 'NONE', *, *, #887, .F. ) ;
#55833=AXIS2_PLACEMENT_3D ( 'NONE', #55908, #21427, #69123 ) ;
#55840=LINE ( 'NONE', #27266, #62793 ) ;
#55852=DIRECTION ( 'NONE',  ( 0.000000000000000000, 0.000000000000000000, -1.000000000000000000 ) ) ;
#55874=FACE_OUTER_BOUND ( 'NONE', #45864, .T. ) ;
#55877=DIRECTION ( 'NONE',  ( -1.000000000000000000, -8.163404592832032979E-16, 0.000000000000000000 ) ) ;
#55878=CARTESIAN_POINT ( 'NONE',  ( 147.0667039027857470, -137.6784471596013191, 245.4218662566959779 ) ) ;
#55887=CARTESIAN_POINT ( 'NONE',  ( 144.5667039024470171, -85.27844715994089597, 55.21780685541800437 ) ) ;
#55891=ORIENTED_EDGE ( 'NONE', *, *, #46034, .F. ) ;
#55894=CIRCLE ( 'NONE', #58755, 17.00000000000000000 ) ;
#55908=CARTESIAN_POINT ( 'NONE',  ( 107.0667039024470313, -104.2784471599420755, -19.78219314458201694 ) ) ;
#55910=ADVANCED_FACE ( 'NONE', ( #86086 ), #31095, .F. ) ;
#55918=CARTESIAN_POINT ( 'NONE',  ( 68.16498115913746858, -136.2709715552406635, 247.3967431772409782 ) ) ;
#55940=EDGE_CURVE ( 'NONE', #43695, #29186, #58789, .T. ) ;
#55971=CYLINDRICAL_SURFACE ( 'NONE', #1119, 1.999999999999995781 ) ;
#55981=CARTESIAN_POINT ( 'NONE',  ( 70.60763308006013972, -139.6429023009440016, 247.2863130087092429 ) ) ;
#55988=CARTESIAN_POINT ( 'NONE',  ( 74.06670390244704549, -118.2784471599409812, 222.2178068554179902 ) ) ;
#55997=FACE_OUTER_BOUND ( 'NONE', #20905, .T. ) ;
#56001=CARTESIAN_POINT ( 'NONE',  ( 108.9744791726667756, -131.7784471599409244, 250.2178068554180470 ) ) ;
#56011=VECTOR ( 'NONE', #53690, 1000.000000000000000 ) ;
#56024=DIRECTION ( 'NONE',  ( -3.100000000000000258E-29, 3.100000000000000044E-14, 1.000000000000000000 ) ) ;
#56033=ORIENTED_EDGE ( 'NONE', *, *, #16581, .F. ) ;
#56036=CARTESIAN_POINT ( 'NONE',  ( 134.5667039024469886, -102.5864808479222319, 250.2178068554180470 ) ) ;
#56045=CARTESIAN_POINT ( 'NONE',  ( 117.4590087478601390, -115.7784471599421181, -21.78219314458165812 ) ) ;
#56046=CARTESIAN_POINT ( 'NONE',  ( 67.07271190493912627, -67.88299602618702977, 245.6488590705319268 ) ) ;
#56065=VERTEX_POINT ( 'NONE', #17913 ) ;
#56075=VECTOR ( 'NONE', #84761, 1000.000000000000000 ) ;
#56076=VECTOR ( 'NONE', #50027, 1000.000000000000000 ) ;
#56078=ORIENTED_EDGE ( 'NONE', *, *, #64316, .T. ) ;
#56105=CARTESIAN_POINT ( 'NONE',  ( 106.5667039024470313, -108.2470741265389620, -19.78219314458190681 ) ) ;
#56111=CARTESIAN_POINT ( 'NONE',  ( 146.5617523730059872, -137.3883890306192939, 246.8362840236234490 ) ) ;
#56135=CARTESIAN_POINT ( 'NONE',  ( 107.5667039024470455, -113.7784471599420613, -19.78219314458171141 ) ) ;
#56148=LINE ( 'NONE', #70708, #65248 ) ;
#56149=VECTOR ( 'NONE', #66570, 999.9999999999998863 ) ;
#56163=CIRCLE ( 'NONE', #22811, 8.999999999999994671 ) ;
#56197=ORIENTED_EDGE ( 'NONE', *, *, #32658, .T. ) ;
#56199=CARTESIAN_POINT ( 'NONE',  ( 97.06670390244703128, -104.2784471599412228, 7.717806855417980394 ) ) ;
#56228=LINE ( 'NONE', #77156, #54615 ) ;
#56245=ORIENTED_EDGE ( 'NONE', *, *, #59230, .F. ) ;
#56257=DIRECTION ( 'NONE',  ( 0.000000000000000000, 0.000000000000000000, -1.000000000000000000 ) ) ;
#56258=ORIENTED_EDGE ( 'NONE', *, *, #68560, .F. ) ;
#56263=EDGE_LOOP ( 'NONE', ( #8189, #67844, #27071, #58174 ) ) ;
#56267=CARTESIAN_POINT ( 'NONE',  ( 140.0667039024470455, -118.2784471599408960, 230.7030882296565721 ) ) ;
#56273=CARTESIAN_POINT ( 'NONE',  ( 121.3178890780284434, -113.5468731908971165, -11.78219314458173272 ) ) ;
#56312=ORIENTED_EDGE ( 'NONE', *, *, #17367, .T. ) ;
#56317=DIRECTION ( 'NONE',  ( -1.000000000000000000, -8.540177112501204385E-16, 0.000000000000000000 ) ) ;
#56340=VECTOR ( 'NONE', #89464, 1000.000000000000000 ) ;
#56345=FILL_AREA_STYLE ('',( #54982 ) ) ;
#56365=DIRECTION ( 'NONE',  ( -1.000000000000000000, 0.000000000000000000, 0.000000000000000000 ) ) ;
#56372=DIRECTION ( 'NONE',  ( 0.000000000000000000, 0.000000000000000000, -1.000000000000000000 ) ) ;
#56374=CARTESIAN_POINT ( 'NONE',  ( 94.20285697596281693, -79.89790063748488080, 250.2178068554180470 ) ) ;
#56375=EDGE_CURVE ( 'NONE', #3973, #960, #8327, .T. ) ;
#56380=EDGE_CURVE ( 'NONE', #22589, #84959, #2390, .T. ) ;
#56388=CARTESIAN_POINT ( 'NONE',  ( 147.0667039024470739, -137.6782278159828934, 245.4503596475569793 ) ) ;
#56398=DIRECTION ( 'NONE',  ( 1.000000000000000000, 0.000000000000000000, 0.000000000000000000 ) ) ;
#56415=CIRCLE ( 'NONE', #54907, 3.500000000000003109 ) ;
#56417=CARTESIAN_POINT ( 'NONE',  ( 102.7030832344709523, -102.3364598618342853, -19.78219314458207378 ) ) ;
#56419=VECTOR ( 'NONE', #77827, 1000.000000000000114 ) ;
#56425=ORIENTED_EDGE ( 'NONE', *, *, #31463, .T. ) ;
#56438=DIRECTION ( 'NONE',  ( 1.000000000000000000, 0.000000000000000000, 0.000000000000000000 ) ) ;
#56440=CARTESIAN_POINT ( 'NONE',  ( 70.74592677485811976, -139.3271945191473833, 247.4287440493089605 ) ) ;
#56446=ORIENTED_EDGE ( 'NONE', *, *, #68135, .T. ) ;
#56450=CARTESIAN_POINT ( 'NONE',  ( 125.5177273812784762, -137.6784471599409301, 55.21780685541800437 ) ) ;
#56463=CARTESIAN_POINT ( 'NONE',  ( 94.20285697596305852, -128.6589936823971527, 250.2178068554179902 ) ) ;
#56487=LINE ( 'NONE', #84675, #31269 ) ;
#56497=CARTESIAN_POINT ( 'NONE',  ( 133.7890526427665634, -110.9887994459054710, 250.2178068554179902 ) ) ;
#56499=FACE_OUTER_BOUND ( 'NONE', #67312, .T. ) ;
#56520=ORIENTED_EDGE ( 'NONE', *, *, #50272, .F. ) ;
#56521=EDGE_LOOP ( 'NONE', ( #69959, #9063 ) ) ;
#56525=VERTEX_POINT ( 'NONE', #47293 ) ;
#56526=VERTEX_POINT ( 'NONE', #87754 ) ;
#56534=AXIS2_PLACEMENT_3D ( 'NONE', #67510, #55202, #70210 ) ;
#56550=DIRECTION ( 'NONE',  ( 1.000000000000000000, 1.000000000000000078E-15, 0.000000000000000000 ) ) ;
#56556=VERTEX_POINT ( 'NONE', #54540 ) ;
#56557=ADVANCED_FACE ( 'NONE', ( #67755 ), #81416, .F. ) ;
#56562=ADVANCED_FACE ( 'NONE', ( #66855 ), #81851, .F. ) ;
#56571=CARTESIAN_POINT ( 'NONE',  ( 140.0667039024470171, -90.27844715994091018, 51.21780685541800437 ) ) ;
#56573=ADVANCED_FACE ( 'NONE', ( #40494 ), #12807, .F. ) ;
#56590=CARTESIAN_POINT ( 'NONE',  ( 144.0637245237351749, -140.6784087391956746, 245.5331728883010101 ) ) ;
#56598=ORIENTED_EDGE ( 'NONE', *, *, #5809, .T. ) ;
#56612=CARTESIAN_POINT ( 'NONE',  ( 70.06670417066791856, -83.77844715994098124, 222.2178068554179902 ) ) ;
#56622=PLANE ( 'NONE',  #43188 ) ;
#56646=EDGE_CURVE ( 'NONE', #33311, #76266, #40933, .T. ) ;
#56688=CARTESIAN_POINT ( 'NONE',  ( 129.4373059489699926, -139.1238275029716362, 247.5908586209667988 ) ) ;
#56689=LINE ( 'NONE', #36262, #44582 ) ;
#56720=VERTEX_POINT ( 'NONE', #7328 ) ;
#56727=CIRCLE ( 'NONE', #17577, 17.00000000000000000 ) ;
#56731=B_SPLINE_CURVE_WITH_KNOTS ( 'NONE', 3,
 ( #11313, #39014, #66265, #25845 ),
 .UNSPECIFIED., .F., .F.,
 ( 4, 4 ),
 ( -0.6035999334370459879, -0.5903216970416090836 ),
 .UNSPECIFIED. ) ;
#56758=VERTEX_POINT ( 'NONE', #37610 ) ;
#56759=VERTEX_POINT ( 'NONE', #87098 ) ;
#56778=CARTESIAN_POINT ( 'NONE',  ( 68.76053423562146349, -136.8603496727827746, 247.4879725229279757 ) ) ;
#56786=EDGE_LOOP ( 'NONE', ( #24130, #53489 ) ) ;
#56803=ORIENTED_EDGE ( 'NONE', *, *, #37268, .F. ) ;
#56817=AXIS2_PLACEMENT_3D ( 'NONE', #35461, #40934, #958 ) ;
#56828=VERTEX_POINT ( 'NONE', #32113 ) ;
#56848=LINE ( 'NONE', #83242, #37241 ) ;
#56868=ADVANCED_FACE ( 'NONE', ( #3089 ), #58474, .T. ) ;
#56883=ADVANCED_FACE ( 'NONE', ( #86205 ), #31672, .F. ) ;
#56892=AXIS2_PLACEMENT_3D ( 'NONE', #6660, #82986, #47525 ) ;
#56893=CARTESIAN_POINT ( 'NONE',  ( 107.0667039024470171, -73.27844715994095282, 25.71780685541800437 ) ) ;
#56894=CARTESIAN_POINT ( 'NONE',  ( 70.36104920614575065, -140.1771413417756094, 246.8581798060137942 ) ) ;
#56897=B_SPLINE_CURVE_WITH_KNOTS ( 'NONE', 3,
 ( #80528, #44640, #18281, #30141 ),
 .UNSPECIFIED., .F., .F.,
 ( 4, 4 ),
 ( -0.6035999334370309999, -0.5903216970415989806 ),
 .UNSPECIFIED. ) ;
#56901=UNCERTAINTY_MEASURE_WITH_UNIT (LENGTH_MEASURE( 1.000000000000000082E-05 ), #69550, 'distance_accuracy_value', 'NONE');
#56907=DIRECTION ( 'NONE',  ( 1.000000000000000078E-15, -1.000000000000000000, 0.000000000000000000 ) ) ;
#56908=CARTESIAN_POINT ( 'NONE',  ( 68.70480626725813522, -139.2920007788289070, 245.9226302269273106 ) ) ;
#56928=ORIENTED_EDGE ( 'NONE', *, *, #1714, .F. ) ;
#56931=PLANE ( 'NONE',  #50075 ) ;
#56932=ORIENTED_EDGE ( 'NONE', *, *, #23863, .F. ) ;
#56944=CARTESIAN_POINT ( 'NONE',  ( 131.3470363009685684, -91.25622735614739156, 250.2178068554180470 ) ) ;
#56950=DIRECTION ( 'NONE',  ( 1.000000000000000000, 7.076552332833900719E-16, 9.062687768214910535E-30 ) ) ;
#56972=ORIENTED_EDGE ( 'NONE', *, *, #87739, .T. ) ;
#56976=ORIENTED_EDGE ( 'NONE', *, *, #61406, .T. ) ;
#56988=ORIENTED_EDGE ( 'NONE', *, *, #52590, .T. ) ;
#57004=ORIENTED_EDGE ( 'NONE', *, *, #41401, .F. ) ;
#57015=DIRECTION ( 'NONE',  ( -1.000000000000000000, -1.541976423090496028E-15, 0.000000000000000000 ) ) ;
#57024=CARTESIAN_POINT ( 'NONE',  ( 122.2221484686747459, -111.8737466215625602, -11.78219314458178779 ) ) ;
#57035=CIRCLE ( 'NONE', #71590, 8.999999999999994671 ) ;
#57039=ORIENTED_EDGE ( 'NONE', *, *, #66498, .F. ) ;
#57052=CARTESIAN_POINT ( 'NONE',  ( 158.0667039024469886, -67.87844715994090450, 190.2178068554179902 ) ) ;
#57055=CIRCLE ( 'NONE', #29454, 2.999999999999975131 ) ;
#57060=ADVANCED_FACE ( 'NONE', ( #42950 ), #63411, .T. ) ;
#57076=DIRECTION ( 'NONE',  ( 0.000000000000000000, 0.000000000000000000, -1.000000000000000000 ) ) ;
#57086=ORIENTED_EDGE ( 'NONE', *, *, #30132, .F. ) ;
#57098=CARTESIAN_POINT ( 'NONE',  ( 70.06670390244707392, -140.6784471599409869, 55.21780685541800437 ) ) ;
#57109=AXIS2_PLACEMENT_3D ( 'NONE', #54404, #53507, #60339 ) ;
#57120=DIRECTION ( 'NONE',  ( -3.100000000000000258E-29, 3.100000000000000044E-14, 1.000000000000000000 ) ) ;
#57133=EDGE_CURVE ( 'NONE', #78225, #23885, #50217, .T. ) ;
#57136=VECTOR ( 'NONE', #64398, 1000.000000000000000 ) ;
#57141=DIRECTION ( 'NONE',  ( -3.100000000000000258E-29, 3.100000000000000044E-14, 1.000000000000000000 ) ) ;
#57177=ORIENTED_EDGE ( 'NONE', *, *, #38964, .T. ) ;
#57184=CARTESIAN_POINT ( 'NONE',  ( 106.1586424053106299, -121.2541776101292186, -11.78219314458148226 ) ) ;
#57189=CARTESIAN_POINT ( 'NONE',  ( 68.89605193404321426, -69.54336780055659517, 247.4970672530039053 ) ) ;
#57194=AXIS2_PLACEMENT_3D ( 'NONE', #83918, #49360, #75746 ) ;
#57199=CIRCLE ( 'NONE', #47074, 2.999999999999975131 ) ;
#57208=CARTESIAN_POINT ( 'NONE',  ( 145.2600001062945978, -139.0446694607154257, 247.0600440238950171 ) ) ;
#57250=DIRECTION ( 'NONE',  ( 1.000000000000000078E-15, -1.000000000000000000, 0.000000000000000000 ) ) ;
#57252=CARTESIAN_POINT ( 'NONE',  ( 110.2536356736639220, -106.6957733451327215, -19.78219314458193168 ) ) ;
#57264=ADVANCED_FACE ( 'NONE', ( #32006 ), #10236, .F. ) ;
#57286=CARTESIAN_POINT ( 'NONE',  ( 103.8797721312301405, -101.8611209747507189, 2.217806855417919998 ) ) ;
#57303=DIRECTION ( 'NONE',  ( -1.000000000000000078E-15, 1.000000000000000000, 0.000000000000000000 ) ) ;
#57305=AXIS2_PLACEMENT_3D ( 'NONE', #37036, #57920, #64742 ) ;
#57326=ADVANCED_FACE ( 'NONE', ( #40615 ), #53770, .T. ) ;
#57337=CARTESIAN_POINT ( 'NONE',  ( 70.74975129634796644, -139.3183301492457247, 247.4318526551172113 ) ) ;
#57360=CARTESIAN_POINT ( 'NONE',  ( 71.06670390244701707, -83.77844715994098124, 45.21780685541799727 ) ) ;
#57391=AXIS2_PLACEMENT_3D ( 'NONE', #72270, #30922, #15067 ) ;
#57424=ORIENTED_EDGE ( 'NONE', *, *, #62807, .F. ) ;
#57439=ORIENTED_EDGE ( 'NONE', *, *, #50297, .F. ) ;
#57447=CARTESIAN_POINT ( 'NONE',  ( 77.44088674023640806, -88.80595668214708382, 249.3055308415380011 ) ) ;
#57462=CIRCLE ( 'NONE', #58870, 21.75000000000000711 ) ;
#57469=LINE ( 'NONE', #56105, #26340 ) ;
#57499=ORIENTED_EDGE ( 'NONE', *, *, #83230, .T. ) ;
#57514=LINE ( 'NONE', #51139, #27748 ) ;
#57518=ORIENTED_EDGE ( 'NONE', *, *, #49290, .F. ) ;
#57521=EDGE_CURVE ( 'NONE', #45437, #59268, #36042, .T. ) ;
#57531=VERTEX_POINT ( 'NONE', #21534 ) ;
#57535=ORIENTED_EDGE ( 'NONE', *, *, #55368, .F. ) ;
#57614=DIRECTION ( 'NONE',  ( 0.000000000000000000, 0.000000000000000000, -1.000000000000000000 ) ) ;
#57620=ORIENTED_EDGE ( 'NONE', *, *, #24160, .F. ) ;
#57634=VERTEX_POINT ( 'NONE', #73225 ) ;
#57644=CARTESIAN_POINT ( 'NONE',  ( 131.5667039024470455, -104.2784471599409244, 24.21780685541800082 ) ) ;
#57690=ORIENTED_EDGE ( 'NONE', *, *, #51752, .F. ) ;
#57731=CIRCLE ( 'NONE', #11302, 17.00000000000000000 ) ;
#57745=DIRECTION ( 'NONE',  ( 0.7071067811865417996, 0.7071067811865532349, 0.000000000000000000 ) ) ;
#57753=PLANE ( 'NONE',  #66258 ) ;
#57754=DIRECTION ( 'NONE',  ( 0.000000000000000000, 0.000000000000000000, 1.000000000000000000 ) ) ;
#57769=CARTESIAN_POINT ( 'NONE',  ( 117.0667039024470455, -109.9573555057410630, 19.21780685541815714 ) ) ;
#57772=FACE_OUTER_BOUND ( 'NONE', #17938, .T. ) ;
#57776=ORIENTED_EDGE ( 'NONE', *, *, #31318, .F. ) ;
#57814=FACE_BOUND ( 'NONE', #76671, .T. ) ;
#57827=ORIENTED_EDGE ( 'NONE', *, *, #83865, .T. ) ;
#57841=ORIENTED_EDGE ( 'NONE', *, *, #12479, .F. ) ;
#57862=CARTESIAN_POINT ( 'NONE',  ( 92.74792143564410196, -71.69957577635202028, 248.4067532124560103 ) ) ;
#57910=CARTESIAN_POINT ( 'NONE',  ( 158.0667039024470171, -79.67844715994088745, 155.2178068554179902 ) ) ;
#57920=DIRECTION ( 'NONE',  ( -0.7071067811875586528, 0.7071067811855363816, -1.379597263674634046E-11 ) ) ;
#57922=CARTESIAN_POINT ( 'NONE',  ( 144.0667039024470739, -140.6784471599409017, 228.4678068554179902 ) ) ;
#57954=DIRECTION ( 'NONE',  ( 0.000000000000000000, 0.000000000000000000, 1.000000000000000000 ) ) ;
#57966=CARTESIAN_POINT ( 'NONE',  ( 162.0667039024469886, -67.87844715994089029, 55.21780685541800437 ) ) ;
#57986=PLANE ( 'NONE',  #19152 ) ;
#57994=ORIENTED_EDGE ( 'NONE', *, *, #29229, .T. ) ;
#57999=VERTEX_POINT ( 'NONE', #76823 ) ;
#58015=CARTESIAN_POINT ( 'NONE',  ( 110.0324702783111661, -88.49073317540081973, -21.02845593540976310 ) ) ;
#58054=DIRECTION ( 'NONE',  ( -3.100000000000000258E-29, 3.100000000000000044E-14, 1.000000000000000000 ) ) ;
#58069=CARTESIAN_POINT ( 'NONE',  ( 110.0667047667142953, -70.87844715994094713, 173.2178068554179902 ) ) ;
#58070=ORIENTED_EDGE ( 'NONE', *, *, #1605, .T. ) ;
#58071=DIRECTION ( 'NONE',  ( -1.000000000000000000, 0.000000000000000000, 0.000000000000000000 ) ) ;
#58080=CARTESIAN_POINT ( 'NONE',  ( 138.0667039024470171, -104.2784471599409244, 45.21780685541799727 ) ) ;
#58081=ORIENTED_EDGE ( 'NONE', *, *, #28833, .T. ) ;
#58094=EDGE_CURVE ( 'NONE', #51807, #20018, #65947, .T. ) ;
#58114=CARTESIAN_POINT ( 'NONE',  ( 144.0667038965492566, -140.6784471658387190, 245.4415720115519832 ) ) ;
#58117=EDGE_CURVE ( 'NONE', #753, #49629, #21027, .T. ) ;
#58122=EDGE_CURVE ( 'NONE', #62435, #65273, #11859, .T. ) ;
#58125=PLANE ( 'NONE',  #65800 ) ;
#58142=VERTEX_POINT ( 'NONE', #30905 ) ;
#58146=DIRECTION ( 'NONE',  ( -3.100000000000000258E-29, 3.100000000000000044E-14, 1.000000000000000000 ) ) ;
#58148=DIRECTION ( 'NONE',  ( 0.8660254037844382635, 0.5000000000000008882, -1.550000000000000022E-14 ) ) ;
#58149=VECTOR ( 'NONE', #58518, 1000.000000000000000 ) ;
#58152=VECTOR ( 'NONE', #29180, 1000.000000000000000 ) ;
#58158=ORIENTED_EDGE ( 'NONE', *, *, #35842, .T. ) ;
#58165=CARTESIAN_POINT ( 'NONE',  ( 67.06670390210777555, -137.6784471596019728, 245.4218662566959779 ) ) ;
#58174=ORIENTED_EDGE ( 'NONE', *, *, #74700, .T. ) ;
#58176=DIRECTION ( 'NONE',  ( -1.000000000000000078E-15, 1.000000000000000000, 0.000000000000000000 ) ) ;
#58210=EDGE_CURVE ( 'NONE', #58962, #4111, #74029, .T. ) ;
#58211=ORIENTED_EDGE ( 'NONE', *, *, #8791, .F. ) ;
#58225=DIRECTION ( 'NONE',  ( 0.8660254037844392627, -0.4999999999999990008, 1.549999999999999706E-14 ) ) ;
#58282=DIRECTION ( 'NONE',  ( 0.7071067811865496822, -0.7071067811865453523, 0.000000000000000000 ) ) ;
#58283=CARTESIAN_POINT ( 'NONE',  ( 154.5667039024470171, -79.67844715994088745, 85.21780685541799016 ) ) ;
#58327=CARTESIAN_POINT ( 'NONE',  ( 63.06670390244699576, -67.87844715994098976, 155.2178068554179902 ) ) ;
#58346=ORIENTED_EDGE ( 'NONE', *, *, #76280, .F. ) ;
#58361=LINE ( 'NONE', #58791, #61156 ) ;
#58396=VERTEX_POINT ( 'NONE', #77171 ) ;
#58397=CIRCLE ( 'NONE', #55511, 30.99999999999998579 ) ;
#58409=ORIENTED_EDGE ( 'NONE', *, *, #80391, .T. ) ;
#58412=CARTESIAN_POINT ( 'NONE',  ( 80.80881079632696640, -112.6232539059703726, 250.2178068554180470 ) ) ;
#58416=AXIS2_PLACEMENT_3D ( 'NONE', #161, #49638, #29223 ) ;
#58426=LINE ( 'NONE', #51601, #10465 ) ;
#58474=PLANE ( 'NONE',  #35545 ) ;
#58475=CARTESIAN_POINT ( 'NONE',  ( 147.0667039024469886, -67.87844715994090450, 222.2178068554179902 ) ) ;
#58485=DIRECTION ( 'NONE',  ( 0.7759704746411385523, -0.6307692307692301936, 0.000000000000000000 ) ) ;
#58490=ADVANCED_FACE ( 'NONE', ( #14500 ), #83101, .T. ) ;
#58493=DIRECTION ( 'NONE',  ( 0.000000000000000000, 0.000000000000000000, 1.000000000000000000 ) ) ;
#58496=EDGE_CURVE ( 'NONE', #78823, #71994, #26857, .T. ) ;
#58518=DIRECTION ( 'NONE',  ( -0.8660254037844392627, 0.4999999999999990008, -1.549999999999999706E-14 ) ) ;
#58519=EDGE_CURVE ( 'NONE', #35863, #15323, #27214, .T. ) ;
#58531=EDGE_CURVE ( 'NONE', #34986, #33347, #74716, .T. ) ;
#58535=CIRCLE ( 'NONE', #41163, 4.500000000000003553 ) ;
#58546=CARTESIAN_POINT ( 'NONE',  ( 145.0753911212546825, -139.6697599411332078, 245.6076672521240027 ) ) ;
#58554=AXIS2_PLACEMENT_3D ( 'NONE', #81682, #6699, #334 ) ;
#58559=DIRECTION ( 'NONE',  ( 0.6757246285173468259, 6.757246285173467929E-16, 0.7371541402007408816 ) ) ;
#58577=LINE ( 'NONE', #44950, #62120 ) ;
#58578=CARTESIAN_POINT ( 'NONE',  ( 120.2221484686747317, -96.68314769832106492, -11.78219314458223188 ) ) ;
#58587=ADVANCED_FACE ( 'NONE', ( #78529 ), #53089, .F. ) ;
#58588=LINE ( 'NONE', #45840, #63485 ) ;
#58596=EDGE_CURVE ( 'NONE', #22318, #78255, #38944, .T. ) ;
#58611=DIRECTION ( 'NONE',  ( 0.000000000000000000, 0.000000000000000000, -1.000000000000000000 ) ) ;
#58632=FACE_BOUND ( 'NONE', #47835, .T. ) ;
#58656=DIRECTION ( 'NONE',  ( 0.000000000000000000, 0.000000000000000000, 1.000000000000000000 ) ) ;
#58665=PLANE ( 'NONE',  #54238 ) ;
#58680=AXIS2_PLACEMENT_3D ( 'NONE', #5188, #68757, #32881 ) ;
#58684=CARTESIAN_POINT ( 'NONE',  ( 69.94616667561825807, -138.0587426493221699, 247.6570821721479945 ) ) ;
#58690=EDGE_CURVE ( 'NONE', #28371, #54294, #69687, .T. ) ;
#58694=ADVANCED_FACE ( 'NONE', ( #14730 ), #77394, .F. ) ;
#58701=EDGE_CURVE ( 'NONE', #6676, #32654, #89313, .T. ) ;
#58702=ORIENTED_EDGE ( 'NONE', *, *, #83917, .T. ) ;
#58736=DIRECTION ( 'NONE',  ( 3.100000000000000258E-29, -3.100000000000000044E-14, -1.000000000000000000 ) ) ;
#58738=CARTESIAN_POINT ( 'NONE',  ( 143.0667039024470171, -90.27844715994091018, 51.21780685541800437 ) ) ;
#58739=DIRECTION ( 'NONE',  ( 0.000000000000000000, 0.000000000000000000, 1.000000000000000000 ) ) ;
#58749=ORIENTED_EDGE ( 'NONE', *, *, #6429, .F. ) ;
#58755=AXIS2_PLACEMENT_3D ( 'NONE', #20704, #63836, #35208 ) ;
#58759=AXIS2_PLACEMENT_3D ( 'NONE', #78651, #50906, #43639 ) ;
#58761=CARTESIAN_POINT ( 'NONE',  ( 106.5667039024470313, -108.2470741265382799, 2.217806855418114065 ) ) ;
#58763=ORIENTED_EDGE ( 'NONE', *, *, #67740, .F. ) ;
#58781=ORIENTED_EDGE ( 'NONE', *, *, #71159, .T. ) ;
#58786=PLANE ( 'NONE',  #71749 ) ;
#58789=LINE ( 'NONE', #72883, #41249 ) ;
#58791=CARTESIAN_POINT ( 'NONE',  ( 143.0667039024470171, -83.77844715994091018, 55.21780685541800437 ) ) ;
#58796=CARTESIAN_POINT ( 'NONE',  ( 68.10560579175795226, -137.1428242527968564, 247.2610778050800491 ) ) ;
#58808=B_SPLINE_CURVE_WITH_KNOTS ( 'NONE', 3,
 ( #52995, #87125, #18513, #46655 ),
 .UNSPECIFIED., .F., .F.,
 ( 4, 4 ),
 ( -0.3974825557268170106, -0.3842043193313839922 ),
 .UNSPECIFIED. ) ;
#58809=CARTESIAN_POINT ( 'NONE',  ( 132.2857443282840393, -124.7784471599409102, 45.21780685541799727 ) ) ;
#58813=DIRECTION ( 'NONE',  ( -1.000000000000000078E-15, 1.000000000000000000, 0.000000000000000000 ) ) ;
#58819=EDGE_LOOP ( 'NONE', ( #53034, #35755 ) ) ;
#58826=DIRECTION ( 'NONE',  ( -0.7071067811865480168, -2.262741699796950529E-14, -0.7071067811865470176 ) ) ;
#58838=PLANE ( 'NONE',  #36810 ) ;
#58849=CARTESIAN_POINT ( 'NONE',  ( 79.56670390244701707, -102.5864808479223456, 250.2178068554179902 ) ) ;
#58854=ADVANCED_FACE ( 'NONE', ( #65546 ), #38282, .F. ) ;
#58866=AXIS2_PLACEMENT_3D ( 'NONE', #25563, #6040, #61420 ) ;
#58870=AXIS2_PLACEMENT_3D ( 'NONE', #33728, #46877, #54134 ) ;
#58881=VERTEX_POINT ( 'NONE', #9691 ) ;
#58886=DIRECTION ( 'NONE',  ( 1.000000000000000078E-15, -1.000000000000000000, 0.000000000000000000 ) ) ;
#58891=CARTESIAN_POINT ( 'NONE',  ( 91.91125933621933086, -96.68314769832132072, -19.26696060647622843 ) ) ;
#58899=EDGE_CURVE ( 'NONE', #37650, #65590, #73702, .T. ) ;
#58952=( BOUNDED_CURVE ( )  B_SPLINE_CURVE ( 2, ( #37135, #58015, #79824 ),
 .UNSPECIFIED., .F., .T. ) 
 B_SPLINE_CURVE_WITH_KNOTS ( ( 3, 3 ),
 ( 0.01169420784673960018, 0.5170228498526568961 ),
 .UNSPECIFIED. ) 
 CURVE ( )  GEOMETRIC_REPRESENTATION_ITEM ( )  RATIONAL_B_SPLINE_CURVE ( ( 1.000420656333759872, 1.009299002520659849, 1.000000000000000000 ) ) 
 REPRESENTATION_ITEM ( '' )  );
#58958=FACE_OUTER_BOUND ( 'NONE', #71362, .T. ) ;
#58962=VERTEX_POINT ( 'NONE', #23786 ) ;
#58964=CARTESIAN_POINT ( 'NONE',  ( 95.83872823098280946, -118.1912118068161703, -9.274842254010202680 ) ) ;
#58968=CARTESIAN_POINT ( 'NONE',  ( 89.91697734863309677, -67.87849423282905548, 246.2109530912199773 ) ) ;
#58973=CARTESIAN_POINT ( 'NONE',  ( 107.0667039024470313, -104.2784471599421323, -21.78219314458201694 ) ) ;
#58975=EDGE_CURVE ( 'NONE', #18397, #12987, #60050, .T. ) ;
#58982=CARTESIAN_POINT ( 'NONE',  ( 162.0667039024470171, -79.67844715994088745, 222.2178068554179902 ) ) ;
#58987=EDGE_CURVE ( 'NONE', #61997, #56720, #32691, .T. ) ;
#58994=CARTESIAN_POINT ( 'NONE',  ( 67.06670390244701707, -79.67844715994098692, 222.2178068554179902 ) ) ;
#59018=LINE ( 'NONE', #87202, #3060 ) ;
#59026=DIRECTION ( 'NONE',  ( 1.075267683398002218E-15, -1.000000000000000000, 3.100000000000000044E-14 ) ) ;
#59036=ADVANCED_FACE ( 'NONE', ( #73239 ), #25101, .T. ) ;
#59038=DIRECTION ( 'NONE',  ( -0.4999999999999985567, -0.8660254037844395958, 2.688821387764040899E-14 ) ) ;
#59056=AXIS2_PLACEMENT_3D ( 'NONE', #59136, #86871, #79619 ) ;
#59105=ORIENTED_EDGE ( 'NONE', *, *, #20140, .F. ) ;
#59129=DIRECTION ( 'NONE',  ( -1.000000000000000000, 0.000000000000000000, 0.000000000000000000 ) ) ;
#59135=AXIS2_PLACEMENT_3D ( 'NONE', #12062, #27034, #81126 ) ;
#59136=CARTESIAN_POINT ( 'NONE',  ( 154.5667039024469886, -67.87844715994090450, 120.2178068554179902 ) ) ;
#59138=FACE_BOUND ( 'NONE', #9535, .T. ) ;
#59141=CARTESIAN_POINT ( 'NONE',  ( 146.6727020897380100, -77.84109957281390280, 247.0017837352540084 ) ) ;
#59148=VECTOR ( 'NONE', #6192, 1000.000000000000000 ) ;
#59155=ORIENTED_EDGE ( 'NONE', *, *, #58496, .F. ) ;
#59184=ORIENTED_EDGE ( 'NONE', *, *, #36164, .T. ) ;
#59189=CARTESIAN_POINT ( 'NONE',  ( 146.0667039024470455, -121.7784471599409102, 55.21780685541800437 ) ) ;
#59201=EDGE_CURVE ( 'NONE', #37855, #47447, #55090, .T. ) ;
#59212=DIRECTION ( 'NONE',  ( -0.7017307308175085856, -0.7121747104283100427, -0.01952340269210590604 ) ) ;
#59214=VERTEX_POINT ( 'NONE', #70478 ) ;
#59218=ORIENTED_EDGE ( 'NONE', *, *, #36053, .F. ) ;
#59230=EDGE_CURVE ( 'NONE', #61133, #75751, #76386, .T. ) ;
#59249=CARTESIAN_POINT ( 'NONE',  ( 67.41169775273984044, -137.4659453879007742, 246.6330592172282081 ) ) ;
#59268=VERTEX_POINT ( 'NONE', #14621 ) ;
#59272=LINE ( 'NONE', #30252, #76362 ) ;
#59299=CARTESIAN_POINT ( 'NONE',  ( 79.72329571771361145, -107.6623471058699835, 250.2178068554180470 ) ) ;
#59337=VERTEX_POINT ( 'NONE', #71819 ) ;
#59344=ORIENTED_EDGE ( 'NONE', *, *, #82134, .T. ) ;
#59356=VECTOR ( 'NONE', #58559, 1000.000000000000114 ) ;
#59362=ORIENTED_EDGE ( 'NONE', *, *, #23594, .T. ) ;
#59370=CARTESIAN_POINT ( 'NONE',  ( 115.0667039024470313, -104.2784471599421181, -21.78219314458201694 ) ) ;
#59377=PLANE ( 'NONE',  #76605 ) ;
#59400=VERTEX_POINT ( 'NONE', #50911 ) ;
#59403=VECTOR ( 'NONE', #32407, 1000.000000000000000 ) ;
#59405=CARTESIAN_POINT ( 'NONE',  ( 106.0667039024470455, -121.2010968907524529, -19.26696060647547881 ) ) ;
#59423=CYLINDRICAL_SURFACE ( 'NONE', #30968, 3.500000000000003109 ) ;
#59429=ORIENTED_EDGE ( 'NONE', *, *, #48557, .F. ) ;
#59446=CARTESIAN_POINT ( 'NONE',  ( 106.5667039024470171, -94.77844715994137914, 2.217806855417697953 ) ) ;
#59453=DIRECTION ( 'NONE',  ( -0.5000000000000015543, 0.8660254037844377084, -2.688821387764056676E-14 ) ) ;
#59459=ORIENTED_EDGE ( 'NONE', *, *, #9677, .F. ) ;
#59481=ORIENTED_EDGE ( 'NONE', *, *, #11458, .T. ) ;
#59519=EDGE_CURVE ( 'NONE', #77969, #34986, #76269, .T. ) ;
#59558=VECTOR ( 'NONE', #22452, 1000.000000000000000 ) ;
#59562=CARTESIAN_POINT ( 'NONE',  ( 135.5667039024470455, -118.2784471599408960, 45.21780685541799727 ) ) ;
#59580=CARTESIAN_POINT ( 'NONE',  ( 145.4065785358296239, -77.83818511938963525, 247.5132519919489766 ) ) ;
#59627=AXIS2_PLACEMENT_3D ( 'NONE', #1108, #28348, #28819 ) ;
#59629=CARTESIAN_POINT ( 'NONE',  ( 146.8914679696725329, -68.04425955369198675, 246.3066688845383965 ) ) ;
#59668=ORIENTED_EDGE ( 'NONE', *, *, #69816, .T. ) ;
#59686=CARTESIAN_POINT ( 'NONE',  ( 67.06673837846007302, -137.6758525980020806, 245.5072637273240161 ) ) ;
#59696=DIRECTION ( 'NONE',  ( -1.000000000000000000, 0.000000000000000000, 0.000000000000000000 ) ) ;
#59697=FACE_OUTER_BOUND ( 'NONE', #87293, .T. ) ;
#59711=FACE_OUTER_BOUND ( 'NONE', #1284, .T. ) ;
#59713=CARTESIAN_POINT ( 'NONE',  ( 107.0667039024470313, -104.2784471599418197, -11.78219314458200984 ) ) ;
#59733=DIRECTION ( 'NONE',  ( 0.08464269478575328631, -0.06148930273953279180, 0.9945122824118421967 ) ) ;
#59744=VECTOR ( 'NONE', #694, 1000.000000000000000 ) ;
#59745=CARTESIAN_POINT ( 'NONE',  ( 109.0351697880554696, -103.7193031201850744, -19.78219314458204536 ) ) ;
#59770=CARTESIAN_POINT ( 'NONE',  ( 99.08946256649485917, -109.4614598618343138, -19.78219314458184996 ) ) ;
#59782=EDGE_CURVE ( 'NONE', #36122, #18229, #86859, .T. ) ;
#59821=CARTESIAN_POINT ( 'NONE',  ( 87.68691565637547569, -140.6784471605521674, 245.6812520957089987 ) ) ;
#59829=EDGE_LOOP ( 'NONE', ( #44678, #42146, #54797, #29894, #39398, #69175, #77704 ) ) ;
#59842=ADVANCED_FACE ( 'NONE', ( #11896 ), #19802, .F. ) ;
#59845=CARTESIAN_POINT ( 'NONE',  ( 80.06670390244696023, -40.87844715994097555, 222.2178068554179902 ) ) ;
#59865=ORIENTED_EDGE ( 'NONE', *, *, #46651, .T. ) ;
#59866=CIRCLE ( 'NONE', #87457, 3.499999999999996003 ) ;
#59873=ORIENTED_EDGE ( 'NONE', *, *, #9500, .T. ) ;
#59917=AXIS2_PLACEMENT_3D ( 'NONE', #15502, #50440, #81972 ) ;
#59928=FACE_OUTER_BOUND ( 'NONE', #76876, .T. ) ;
#59942=CARTESIAN_POINT ( 'NONE',  ( 69.94616667561825807, -138.0587426493221699, 247.6570821721479945 ) ) ;
#59944=ORIENTED_EDGE ( 'NONE', *, *, #70287, .T. ) ;
#59958=VERTEX_POINT ( 'NONE', #23537 ) ;
#59964=LINE ( 'NONE', #26803, #72262 ) ;
#59970=EDGE_LOOP ( 'NONE', ( #67440, #21127, #55776, #63894, #89852, #80517 ) ) ;
#59975=EDGE_CURVE ( 'NONE', #70808, #16796, #11087, .T. ) ;
#59997=CARTESIAN_POINT ( 'NONE',  ( 107.0667039024470313, -104.2784471599420471, -19.18411693322902423 ) ) ;
#60002=VERTEX_POINT ( 'NONE', #83185 ) ;
#60010=AXIS2_PLACEMENT_3D ( 'NONE', #6097, #62381, #162 ) ;
#60019=DIRECTION ( 'NONE',  ( 0.5000000000000008882, -0.8660254037844382635, 2.684678751731760294E-14 ) ) ;
#60021=DIRECTION ( 'NONE',  ( -1.000000000000000078E-15, 1.000000000000000000, 0.000000000000000000 ) ) ;
#60026=LINE ( 'NONE', #33242, #35565 ) ;
#60027=VERTEX_POINT ( 'NONE', #11214 ) ;
#60038=EDGE_LOOP ( 'NONE', ( #26798, #47255, #61772, #58781 ) ) ;
#60044=ORIENTED_EDGE ( 'NONE', *, *, #5816, .T. ) ;
#60050=LINE ( 'NONE', #71926, #18165 ) ;
#60056=VERTEX_POINT ( 'NONE', #3960 ) ;
#60101=EDGE_LOOP ( 'NONE', ( #28907, #72726, #50625, #53252 ) ) ;
#60108=AXIS2_PLACEMENT_3D ( 'NONE', #49670, #83775, #1093 ) ;
#60113=DIRECTION ( 'NONE',  ( -1.000000000000000000, -1.734723475976808672E-15, 0.000000000000000000 ) ) ;
#60125=CARTESIAN_POINT ( 'NONE',  ( 143.8525571913658894, -140.3399344531919155, 246.6497317326439429 ) ) ;
#60131=CARTESIAN_POINT ( 'NONE',  ( 68.01586774711397254, -137.1827438074501799, 247.2088461600285996 ) ) ;
#60144=CARTESIAN_POINT ( 'NONE',  ( 97.06670390244703128, -104.2784471599409244, 17.71780685541799016 ) ) ;
#60149=ORIENTED_EDGE ( 'NONE', *, *, #53470, .F. ) ;
#60161=DIRECTION ( 'NONE',  ( -1.000000000000000000, -1.541976423090496028E-15, 0.000000000000000000 ) ) ;
#60170=VECTOR ( 'NONE', #57954, 1000.000000000000000 ) ;
#60172=DIRECTION ( 'NONE',  ( -1.000000000000000000, -1.206764157201257538E-15, 0.000000000000000000 ) ) ;
#60182=VERTEX_POINT ( 'NONE', #719 ) ;
#60190=VERTEX_POINT ( 'NONE', #54311 ) ;
#60192=PLANE ( 'NONE',  #81577 ) ;
#60198=CARTESIAN_POINT ( 'NONE',  ( 118.5667039024470313, -104.2784471599408533, 19.21780685541799016 ) ) ;
#60217=ORIENTED_EDGE ( 'NONE', *, *, #27740, .T. ) ;
#60261=FACE_OUTER_BOUND ( 'NONE', #71085, .T. ) ;
#60271=CARTESIAN_POINT ( 'NONE',  ( 112.3567964431407660, -140.4754596735087375, 246.9959941585700278 ) ) ;
#60278=ORIENTED_EDGE ( 'NONE', *, *, #47635, .T. ) ;
#60279=ORIENTED_EDGE ( 'NONE', *, *, #70412, .T. ) ;
#60283=VECTOR ( 'NONE', #12426, 1000.000000000000000 ) ;
#60301=ORIENTED_EDGE ( 'NONE', *, *, #64557, .T. ) ;
#60311=CARTESIAN_POINT ( 'NONE',  ( 67.05726156256010029, -68.28389950123548147, 246.9923701901030029 ) ) ;
#60323=EDGE_CURVE ( 'NONE', #47465, #43325, #36606, .T. ) ;
#60326=ORIENTED_EDGE ( 'NONE', *, *, #14150, .F. ) ;
#60339=DIRECTION ( 'NONE',  ( 1.000000000000000000, 0.000000000000000000, 0.000000000000000000 ) ) ;
#60378=PRODUCT ( 'Drilling Spindle Head', 'Drilling Spindle Head', '', ( #87210 ) ) ;
#60380=CARTESIAN_POINT ( 'NONE',  ( 108.0667039024470455, -121.2010968907525239, -21.78219314458149114 ) ) ;
#60382=CARTESIAN_POINT ( 'NONE',  ( 68.06670390244705970, -124.7784471599409954, 55.21780685541800437 ) ) ;
#60406=CARTESIAN_POINT ( 'NONE',  ( 108.0667039024470171, -87.35579742913141388, -11.78219314458253741 ) ) ;
#60431=EDGE_CURVE ( 'NONE', #58396, #85229, #12016, .T. ) ;
#60449=CARTESIAN_POINT ( 'NONE',  ( 70.06670417066790435, -71.37844715994097555, 55.21780685541800437 ) ) ;
#60454=CARTESIAN_POINT ( 'NONE',  ( 117.9332873271178102, -93.05227202534700837, -11.78219314458237044 ) ) ;
#60467=CIRCLE ( 'NONE', #61898, 8.999999999999994671 ) ;
#60483=VECTOR ( 'NONE', #56257, 1000.000000000000000 ) ;
#60502=CARTESIAN_POINT ( 'NONE',  ( 81.84766347661003749, -124.7784471599409670, 55.21780685541800437 ) ) ;
#60517=CARTESIAN_POINT ( 'NONE',  ( 106.5667039024470313, -108.2470741265382799, 2.217806855418114065 ) ) ;
#60535=EDGE_CURVE ( 'NONE', #1304, #80721, #52407, .T. ) ;
#60539=CARTESIAN_POINT ( 'NONE',  ( 70.56670390244700286, -67.87844715994098976, 55.21780685541800437 ) ) ;
#60540=EDGE_CURVE ( 'NONE', #14173, #31404, #45950, .T. ) ;
#60557=ADVANCED_FACE ( 'NONE', ( #46050 ), #80616, .F. ) ;
#60578=DIRECTION ( 'NONE',  ( 0.000000000000000000, 0.000000000000000000, 1.000000000000000000 ) ) ;
#60585=CARTESIAN_POINT ( 'NONE',  ( 67.56670413341505821, -124.7784471599409954, 45.21780685541799727 ) ) ;
#60610=CARTESIAN_POINT ( 'NONE',  ( 114.6444261855608460, -91.15344715994180547, -11.78219314458242550 ) ) ;
#60621=AXIS2_PLACEMENT_3D ( 'NONE', #2875, #64644, #8808 ) ;
#60627=DIRECTION ( 'NONE',  ( 0.000000000000000000, 0.000000000000000000, -1.000000000000000000 ) ) ;
#60632=CARTESIAN_POINT ( 'NONE',  ( 154.5667039024469886, -67.87844715994090450, 190.2178068554179902 ) ) ;
#60635=ORIENTED_EDGE ( 'NONE', *, *, #5940, .F. ) ;
#60640=CARTESIAN_POINT ( 'NONE',  ( 107.0667039024470313, -104.2784471599418197, -11.78219314458200984 ) ) ;
#60644=ORIENTED_EDGE ( 'NONE', *, *, #38100, .F. ) ;
#60660=EDGE_LOOP ( 'NONE', ( #72083, #64528, #7580, #21140, #82027, #9217, #70282, #47286, #7434, #26701 ) ) ;
#60675=CIRCLE ( 'NONE', #50571, 11.49999999999999645 ) ;
#60691=FACE_OUTER_BOUND ( 'NONE', #46232, .T. ) ;
#60701=DIRECTION ( 'NONE',  ( 1.000000000000000000, 0.000000000000000000, 0.000000000000000000 ) ) ;
#60715=VECTOR ( 'NONE', #79373, 1000.000000000000000 ) ;
#60721=CARTESIAN_POINT ( 'NONE',  ( 122.2221484686747459, -111.9108568887688477, -19.23816181211476817 ) ) ;
#60776=CONICAL_SURFACE ( 'NONE', #72413, 16.25000000000000000, 0.5235987755982992597 ) ;
#60791=CARTESIAN_POINT ( 'NONE',  ( 98.06670390244704549, -104.2784471599411376, 2.217806855418003043 ) ) ;
#60795=FACE_OUTER_BOUND ( 'NONE', #16218, .T. ) ;
#60818=CARTESIAN_POINT ( 'NONE',  ( 107.0667039024470313, -104.2784471599414502, 0.2178068554180012661 ) ) ;
#60823=LINE ( 'NONE', #43404, #10813 ) ;
#60830=DIRECTION ( 'NONE',  ( -3.100000000000000258E-29, 3.100000000000000044E-14, 1.000000000000000000 ) ) ;
#60831=DIRECTION ( 'NONE',  ( -3.100000000000000258E-29, 3.100000000000000044E-14, 1.000000000000000000 ) ) ;
#60836=ORIENTED_EDGE ( 'NONE', *, *, #53890, .T. ) ;
#60837=EDGE_CURVE ( 'NONE', #70844, #29186, #31446, .T. ) ;
#60844=ADVANCED_FACE ( 'NONE', ( #55997 ), #49642, .F. ) ;
#60846=DIRECTION ( 'NONE',  ( -1.000000000000000000, -1.541976423090496028E-15, 0.000000000000000000 ) ) ;
#60881=EDGE_CURVE ( 'NONE', #78112, #17073, #53194, .T. ) ;
#60901=EDGE_CURVE ( 'NONE', #31453, #60027, #87314, .T. ) ;
#60925=DIRECTION ( 'NONE',  ( -3.100000000000000258E-29, 3.100000000000000044E-14, 1.000000000000000000 ) ) ;
#60945=B_SPLINE_CURVE_WITH_KNOTS ( 'NONE', 3,
 ( #53793, #54235, #81112, #19755, #47435 ),
 .UNSPECIFIED., .F., .F.,
 ( 4, 1, 4 ),
 ( 0.000000000000000000, 0.4203864884934794266, 1.000000000000000000 ),
 .UNSPECIFIED. ) ;
#60951=EDGE_CURVE ( 'NONE', #32654, #6676, #5398, .T. ) ;
#60953=ORIENTED_EDGE ( 'NONE', *, *, #37085, .T. ) ;
#60982=LINE ( 'NONE', #33729, #30398 ) ;
#60991=DIRECTION ( 'NONE',  ( 1.000000000000000000, 0.000000000000000000, 0.000000000000000000 ) ) ;
#60993=ORIENTED_EDGE ( 'NONE', *, *, #15058, .T. ) ;
#61015=CARTESIAN_POINT ( 'NONE',  ( 46.61670390244704976, -117.2284471599409983, 55.21780685541799727 ) ) ;
#61024=VERTEX_POINT ( 'NONE', #40938 ) ;
#61038=CARTESIAN_POINT ( 'NONE',  ( 92.87912090207764493, -113.5872422955286538, -19.23816181211473975 ) ) ;
#61056=CYLINDRICAL_SURFACE ( 'NONE', #82796, 2.000000000000001776 ) ;
#61071=AXIS2_PLACEMENT_3D ( 'NONE', #62089, #89823, #1678 ) ;
#61078=VECTOR ( 'NONE', #83084, 1000.000000000000000 ) ;
#61084=DIRECTION ( 'NONE',  ( -1.000000000000000000, -1.000000000000000078E-15, 0.000000000000000000 ) ) ;
#61099=( BOUNDED_CURVE ( )  B_SPLINE_CURVE ( 2, ( #107, #50024, #78224 ),
 .UNSPECIFIED., .F., .T. ) 
 B_SPLINE_CURVE_WITH_KNOTS ( ( 3, 3 ),
 ( 0.000000000000000000, 0.5053286420056760653 ),
 .UNSPECIFIED. ) 
 CURVE ( )  GEOMETRIC_REPRESENTATION_ITEM ( )  RATIONAL_B_SPLINE_CURVE ( ( 1.000000000000000000, 1.009299002520649857, 1.000420656333769864 ) ) 
 REPRESENTATION_ITEM ( '' )  );
#61103=VERTEX_POINT ( 'NONE', #40042 ) ;
#61108=EDGE_LOOP ( 'NONE', ( #38391, #10044 ) ) ;
#61113=LINE ( 'NONE', #6168, #89362 ) ;
#61114=CARTESIAN_POINT ( 'NONE',  ( 107.0667039024470313, -104.2784471599409528, 24.21780685541800082 ) ) ;
#61118=CARTESIAN_POINT ( 'NONE',  ( 59.56670390244700997, -79.67844715994098692, 155.2178068554179902 ) ) ;
#61120=ORIENTED_EDGE ( 'NONE', *, *, #71571, .T. ) ;
#61126=B_SPLINE_SURFACE_WITH_KNOTS ( 'NONE', 3, 3, ( 
 ( #38102, #30842, #73961, #3578, #11739, #73508, #86256 ),
 ( #32611, #45337, #24038, #31274, #58968, #44902, #86706 ),
 ( #10833, #39438, #52144, #45780, #79907, #17662, #60311 ),
 ( #38539, #88048, #53484, #9960, #37663, #47575, #6706 ),
 ( #70626, #8404, #61653, #40773, #13528, #6264, #62115 ) ),
 .UNSPECIFIED., .F., .F., .F.,
 ( 4, 1, 4 ),
 ( 4, 1, 1, 1, 4 ),
 ( 0.000000000000000000, 0.5714285714285709528, 1.000000000000000000 ),
 ( -0.1863387531781160178, 0.9565458916201099449, 3.242315181216560038, 5.528084470813009688, 7.813853760409459781 ),
 .UNSPECIFIED. ) ;
#61128=DIRECTION ( 'NONE',  ( 1.000000000000000078E-15, -1.000000000000000000, 0.000000000000000000 ) ) ;
#61133=VERTEX_POINT ( 'NONE', #5548 ) ;
#61134=VECTOR ( 'NONE', #69027, 1000.000000000000227 ) ;
#61139=DIRECTION ( 'NONE',  ( 0.000000000000000000, 0.000000000000000000, -1.000000000000000000 ) ) ;
#61156=VECTOR ( 'NONE', #51968, 1000.000000000000000 ) ;
#61165=DIRECTION ( 'NONE',  ( -0.8660254037844380415, -0.5000000000000012212, 1.550000000000001284E-14 ) ) ;
#61177=CARTESIAN_POINT ( 'NONE',  ( 70.05589428573307487, -139.0036297784914723, 247.5065103411480152 ) ) ;
#61179=CARTESIAN_POINT ( 'NONE',  ( 145.3881220512730295, -139.2530407526492127, 246.1986748867973347 ) ) ;
#61183=ORIENTED_EDGE ( 'NONE', *, *, #71273, .F. ) ;
#61185=VECTOR ( 'NONE', #17998, 1000.000000000000000 ) ;
#61200=PLANE ( 'NONE',  #80090 ) ;
#61228=DIRECTION ( 'NONE',  ( -3.100000000000000258E-29, 3.100000000000000044E-14, 1.000000000000000000 ) ) ;
#61237=DIRECTION ( 'NONE',  ( 0.7071067811865487940, -0.7071067811865463515, 0.000000000000000000 ) ) ;
#61240=ORIENTED_EDGE ( 'NONE', *, *, #10978, .T. ) ;
#61242=LINE ( 'NONE', #27176, #15611 ) ;
#61250=DIRECTION ( 'NONE',  ( 1.000000000000000000, 1.000000000000000078E-15, 0.000000000000000000 ) ) ;
#61256=EDGE_LOOP ( 'NONE', ( #63906, #61964, #3021, #4872, #40027, #16319 ) ) ;
#61265=ORIENTED_EDGE ( 'NONE', *, *, #79757, .T. ) ;
#61289=DIRECTION ( 'NONE',  ( 0.4999999999999998335, 0.8660254037844387076, -2.684678751731758400E-14 ) ) ;
#61301=EDGE_CURVE ( 'NONE', #32654, #1337, #35920, .T. ) ;
#61315=VERTEX_POINT ( 'NONE', #84997 ) ;
#61350=EDGE_CURVE ( 'NONE', #65691, #25396, #76455, .T. ) ;
#61356=CARTESIAN_POINT ( 'NONE',  ( 80.75703168202301185, -80.31070608727497984, 249.3055308415380011 ) ) ;
#61361=VERTEX_POINT ( 'NONE', #22310 ) ;
#61383=EDGE_CURVE ( 'NONE', #45687, #42534, #83728, .T. ) ;
#61388=CARTESIAN_POINT ( 'NONE',  ( 143.5667039024469886, -67.87844715994090450, 222.2178068554179902 ) ) ;
#61397=ORIENTED_EDGE ( 'NONE', *, *, #49788, .T. ) ;
#61404=CARTESIAN_POINT ( 'NONE',  ( 68.97389088270736579, -137.8496454943130800, 247.5170344592769993 ) ) ;
#61406=EDGE_CURVE ( 'NONE', #13042, #2833, #58588, .T. ) ;
#61415=CARTESIAN_POINT ( 'NONE',  ( 97.06670390244701707, -98.59953881414098475, 7.717806855417813416 ) ) ;
#61420=DIRECTION ( 'NONE',  ( 0.000000000000000000, 0.000000000000000000, -1.000000000000000000 ) ) ;
#61447=VECTOR ( 'NONE', #40141, 1000.000000000000000 ) ;
#61454=EDGE_CURVE ( 'NONE', #65034, #43695, #76527, .T. ) ;
#61475=SURFACE_SIDE_STYLE ('',( #40593 ) ) ;
#61479=DIRECTION ( 'NONE',  ( 0.000000000000000000, 0.000000000000000000, 1.000000000000000000 ) ) ;
#61511=EDGE_CURVE ( 'NONE', #13876, #79449, #88142, .T. ) ;
#61514=ORIENTED_EDGE ( 'NONE', *, *, #27466, .T. ) ;
#61519=CARTESIAN_POINT ( 'NONE',  ( 107.0667039024470313, -104.2784471599412086, 7.717806855417980394 ) ) ;
#61528=ORIENTED_EDGE ( 'NONE', *, *, #32347, .F. ) ;
#61542=VERTEX_POINT ( 'NONE', #7671 ) ;
#61554=VERTEX_POINT ( 'NONE', #49431 ) ;
#61573=ORIENTED_EDGE ( 'NONE', *, *, #44463, .F. ) ;
#61574=DIRECTION ( 'NONE',  ( 1.000000000000000000, 0.000000000000000000, 0.000000000000000000 ) ) ;
#61577=CARTESIAN_POINT ( 'NONE',  ( 52.06670390244700997, -79.67844715994100113, 55.21780685541800437 ) ) ;
#61588=EDGE_CURVE ( 'NONE', #753, #51345, #14496, .T. ) ;
#61604=DIRECTION ( 'NONE',  ( -1.000000000000000000, -8.163404592832032979E-16, 0.000000000000000000 ) ) ;
#61607=AXIS2_PLACEMENT_3D ( 'NONE', #9137, #65858, #79074 ) ;
#61615=CARTESIAN_POINT ( 'NONE',  ( 97.81670390244700286, -68.87844715994096134, 222.2178068554179902 ) ) ;
#61617=CARTESIAN_POINT ( 'NONE',  ( 144.0775135191610730, -139.0036297784913870, 247.5065103411480152 ) ) ;
#61618=CARTESIAN_POINT ( 'NONE',  ( 145.3183308313961675, -139.1845296323008938, 246.4818851000068491 ) ) ;
#61640=EDGE_CURVE ( 'NONE', #78112, #33950, #46085, .T. ) ;
#61641=VECTOR ( 'NONE', #87087, 1000.000000000000000 ) ;
#61653=CARTESIAN_POINT ( 'NONE',  ( 131.8488129342790103, -69.46958951562531581, 247.5788556710219837 ) ) ;
#61661=VECTOR ( 'NONE', #16444, 1000.000000000000000 ) ;
#61684=FACE_OUTER_BOUND ( 'NONE', #47007, .T. ) ;
#61699=FACE_OUTER_BOUND ( 'NONE', #35016, .T. ) ;
#61723=ORIENTED_EDGE ( 'NONE', *, *, #4372, .F. ) ;
#61728=ADVANCED_FACE ( 'NONE', ( #44860 ), #75093, .T. ) ;
#61744=ADVANCED_FACE ( 'NONE', ( #37620 ), #71697, .T. ) ;
#61772=ORIENTED_EDGE ( 'NONE', *, *, #35992, .T. ) ;
#61773=ORIENTED_EDGE ( 'NONE', *, *, #52220, .T. ) ;
#61782=ORIENTED_EDGE ( 'NONE', *, *, #22138, .T. ) ;
#61794=DIRECTION ( 'NONE',  ( 0.000000000000000000, 0.000000000000000000, 1.000000000000000000 ) ) ;
#61812=CARTESIAN_POINT ( 'NONE',  ( 102.2800657950380696, -137.4712196896787475, 248.4142799812389910 ) ) ;
#61815=CARTESIAN_POINT ( 'NONE',  ( 107.5667039024470313, -100.3098201933451605, -19.78219314458212708 ) ) ;
#61836=LINE ( 'NONE', #28679, #35556 ) ;
#61847=VERTEX_POINT ( 'NONE', #86663 ) ;
#61853=AXIS2_PLACEMENT_3D ( 'NONE', #80114, #58736, #45992 ) ;
#61867=ORIENTED_EDGE ( 'NONE', *, *, #38525, .T. ) ;
#61870=ADVANCED_FACE ( 'NONE', ( #3983 ), #59377, .T. ) ;
#61878=EDGE_CURVE ( 'NONE', #77969, #30086, #38940, .T. ) ;
#61893=ORIENTED_EDGE ( 'NONE', *, *, #50711, .T. ) ;
#61898=AXIS2_PLACEMENT_3D ( 'NONE', #67644, #49420, #28086 ) ;
#61921=AXIS2_PLACEMENT_3D ( 'NONE', #62772, #49580, #56398 ) ;
#61931=CARTESIAN_POINT ( 'NONE',  ( 116.3167039024470029, -67.87844715994093292, 222.2178068554179902 ) ) ;
#61937=ORIENTED_EDGE ( 'NONE', *, *, #33511, .T. ) ;
#61950=ORIENTED_EDGE ( 'NONE', *, *, #75028, .T. ) ;
#61964=ORIENTED_EDGE ( 'NONE', *, *, #5802, .T. ) ;
#61966=EDGE_LOOP ( 'NONE', ( #27901, #46178, #54047 ) ) ;
#61969=DIRECTION ( 'NONE',  ( 3.100000000000000258E-29, -3.100000000000000044E-14, -1.000000000000000000 ) ) ;
#61975=EDGE_CURVE ( 'NONE', #33837, #11800, #4094, .T. ) ;
#61977=CARTESIAN_POINT ( 'NONE',  ( 67.21995684885473565, -68.02541542198279956, 246.2600046646611816 ) ) ;
#61994=LINE ( 'NONE', #13857, #77975 ) ;
#61997=VERTEX_POINT ( 'NONE', #32123 ) ;
#62006=VECTOR ( 'NONE', #69863, 1000.000000000000000 ) ;
#62014=EDGE_LOOP ( 'NONE', ( #85336, #82894, #12304, #63227, #1348 ) ) ;
#62026=ORIENTED_EDGE ( 'NONE', *, *, #83968, .F. ) ;
#62033=CARTESIAN_POINT ( 'NONE',  ( 121.2221484686747317, -94.95109689075249548, -21.78219314458229405 ) ) ;
#62039=CARTESIAN_POINT ( 'NONE',  ( 74.06670390244701707, -90.27844715994098124, 51.21780685541800437 ) ) ;
#62069=EDGE_LOOP ( 'NONE', ( #24600, #2302, #43240, #33060 ) ) ;
#62070=DIRECTION ( 'NONE',  ( -3.100000000000000258E-29, 3.100000000000000044E-14, 1.000000000000000000 ) ) ;
#62078=AXIS2_PLACEMENT_3D ( 'NONE', #14128, #21395, #12791 ) ;
#62089=CARTESIAN_POINT ( 'NONE',  ( 93.91125933621934507, -111.8737466215625744, -11.78219314458178779 ) ) ;
#62092=ADVANCED_FACE ( 'NONE', ( #23339 ), #54830, .T. ) ;
#62095=CYLINDRICAL_SURFACE ( 'NONE', #29857, 4.500000000000003553 ) ;
#62115=CARTESIAN_POINT ( 'NONE',  ( 67.05404872073289368, -69.57571276584442899, 247.4899279706389734 ) ) ;
#62120=VECTOR ( 'NONE', #58148, 999.9999999999998863 ) ;
#62137=CIRCLE ( 'NONE', #83949, 7.999999999999992895 ) ;
#62155=DIRECTION ( 'NONE',  ( -1.000000000000000000, -1.000000000000000078E-15, 0.000000000000000000 ) ) ;
#62178=CARTESIAN_POINT ( 'NONE',  ( 70.06670390441306040, -140.6784471619069734, 245.4415720117440003 ) ) ;
#62180=CARTESIAN_POINT ( 'NONE',  ( 74.19170390244705970, -127.9034471599409812, 55.21780685541800437 ) ) ;
#62195=CIRCLE ( 'NONE', #20131, 3.000000000000002665 ) ;
#62214=ORIENTED_EDGE ( 'NONE', *, *, #42428, .F. ) ;
#62249=AXIS2_PLACEMENT_3D ( 'NONE', #36740, #71270, #49443 ) ;
#62252=LINE ( 'NONE', #67730, #67229 ) ;
#62263=ORIENTED_EDGE ( 'NONE', *, *, #30979, .F. ) ;
#62265=ORIENTED_EDGE ( 'NONE', *, *, #58117, .T. ) ;
#62268=CARTESIAN_POINT ( 'NONE',  ( 72.52678588541827764, -139.0845773098406823, 247.5112265945679724 ) ) ;
#62282=DIRECTION ( 'NONE',  ( -1.000000000000000078E-15, 1.000000000000000000, 0.000000000000000000 ) ) ;
#62291=CARTESIAN_POINT ( 'NONE',  ( 137.9639241664444285, -93.39344735187280833, 249.3055338466990065 ) ) ;
#62304=CARTESIAN_POINT ( 'NONE',  ( 52.06670390244699576, -67.87844715994100397, 55.21780685541800437 ) ) ;
#62366=CARTESIAN_POINT ( 'NONE',  ( 70.11541878361150282, -140.6397552082484310, 245.9889283728621763 ) ) ;
#62380=CYLINDRICAL_SURFACE ( 'NONE', #58416, 1.999999999999995781 ) ;
#62381=DIRECTION ( 'NONE',  ( -1.000000000000000000, -1.777766061779359009E-15, 2.411074791516012434E-29 ) ) ;
#62382=AXIS2_PLACEMENT_3D ( 'NONE', #89624, #7391, #41886 ) ;
#62391=PLANE ( 'NONE',  #48090 ) ;
#62399=LINE ( 'NONE', #55555, #74078 ) ;
#62405=ORIENTED_EDGE ( 'NONE', *, *, #50205, .F. ) ;
#62416=DIRECTION ( 'NONE',  ( 3.100000000000000258E-29, -3.100000000000000044E-14, -1.000000000000000000 ) ) ;
#62423=( BOUNDED_CURVE ( )  B_SPLINE_CURVE ( 2, ( #62874, #28352, #56045 ),
 .UNSPECIFIED., .F., .T. ) 
 B_SPLINE_CURVE_WITH_KNOTS ( ( 3, 3 ),
 ( 0.01169420784674039988, 0.5170228498526580063 ),
 .UNSPECIFIED. ) 
 CURVE ( )  GEOMETRIC_REPRESENTATION_ITEM ( )  RATIONAL_B_SPLINE_CURVE ( ( 1.000420656333759872, 1.009299002520659849, 1.000000000000000000 ) ) 
 REPRESENTATION_ITEM ( '' )  );
#62425=DIRECTION ( 'NONE',  ( 1.000000000000000000, 1.000000000000000078E-15, 0.000000000000000000 ) ) ;
#62428=DIRECTION ( 'NONE',  ( 0.5000000000000016653, -0.8660254037844377084, 2.684678751731758716E-14 ) ) ;
#62432=CARTESIAN_POINT ( 'NONE',  ( 68.23039785489001474, -68.99015375674828476, 247.3122147236876458 ) ) ;
#62435=VERTEX_POINT ( 'NONE', #20969 ) ;
#62442=ADVANCED_FACE ( 'NONE', ( #82770 ), #25565, .F. ) ;
#62447=DIRECTION ( 'NONE',  ( -3.100000000000000258E-29, 3.100000000000000044E-14, 1.000000000000000000 ) ) ;
#62451=CIRCLE ( 'NONE', #23325, 4.000000000000006217 ) ;
#62459=LINE ( 'NONE', #55613, #4450 ) ;
#62476=ORIENTED_EDGE ( 'NONE', *, *, #44641, .F. ) ;
#62506=FACE_OUTER_BOUND ( 'NONE', #44583, .T. ) ;
#62519=DIRECTION ( 'NONE',  ( 1.000000000000000000, 1.000000000000000078E-15, 0.000000000000000000 ) ) ;
#62528=ADVANCED_FACE ( 'NONE', ( #43184 ), #1431, .F. ) ;
#62529=CARTESIAN_POINT ( 'NONE',  ( 145.1686704281712821, -139.0359729423161639, 246.8427441825336928 ) ) ;
#62538=CARTESIAN_POINT ( 'NONE',  ( 117.0667039024470313, -104.2784471599408960, 17.71780685541799016 ) ) ;
#62545=DIRECTION ( 'NONE',  ( 1.000000000000000000, 0.000000000000000000, 0.000000000000000000 ) ) ;
#62550=AXIS2_PLACEMENT_3D ( 'NONE', #22924, #3800, #72407 ) ;
#62580=DIRECTION ( 'NONE',  ( -1.000000000000000000, -1.734723475976808672E-15, 0.000000000000000000 ) ) ;
#62603=PLANE ( 'NONE',  #86061 ) ;
#62619=ORIENTED_EDGE ( 'NONE', *, *, #73887, .F. ) ;
#62626=CARTESIAN_POINT ( 'NONE',  ( 106.5667039024470313, -100.3098201933451747, -19.78219314458212708 ) ) ;
#62629=DIRECTION ( 'NONE',  ( 0.000000000000000000, 1.000000000000000000, 0.000000000000000000 ) ) ;
#62630=AXIS2_PLACEMENT_3D ( 'NONE', #38739, #38294, #80103 ) ;
#62643=CIRCLE ( 'NONE', #40843, 4.000000000000002665 ) ;
#62653=EDGE_CURVE ( 'NONE', #66921, #49274, #86835, .T. ) ;
#62661=LINE ( 'NONE', #76745, #88504 ) ;
#62672=DIRECTION ( 'NONE',  ( -3.100000000000000258E-29, 3.100000000000000044E-14, 1.000000000000000000 ) ) ;
#62678=VECTOR ( 'NONE', #54736, 1000.000000000000114 ) ;
#62688=DIRECTION ( 'NONE',  ( 1.000000000000000078E-15, -1.000000000000000000, 0.000000000000000000 ) ) ;
#62694=AXIS2_PLACEMENT_3D ( 'NONE', #60640, #66566, #12063 ) ;
#62698=ORIENTED_EDGE ( 'NONE', *, *, #39227, .T. ) ;
#62711=CARTESIAN_POINT ( 'NONE',  ( 99.08946256649487339, -99.09543445804985140, -19.78219314458218392 ) ) ;
#62719=DIRECTION ( 'NONE',  ( 0.9217329428042198014, 0.3878251953515564066, -1.203464411458912131E-14 ) ) ;
#62721=CARTESIAN_POINT ( 'NONE',  ( 68.70620082986425814, -127.7162791817593757, 247.5270151222840127 ) ) ;
#62723=ORIENTED_EDGE ( 'NONE', *, *, #32347, .T. ) ;
#62745=ORIENTED_EDGE ( 'NONE', *, *, #71938, .F. ) ;
#62749=CARTESIAN_POINT ( 'NONE',  ( 127.4058501689330996, -85.76982405743852667, 250.2178068554179902 ) ) ;
#62752=CARTESIAN_POINT ( 'NONE',  ( 68.21308206361896964, -138.8248129988772916, 246.0151717635989996 ) ) ;
#62772=CARTESIAN_POINT ( 'NONE',  ( 154.5667039024470171, -79.67844715994088745, 155.2178068554179902 ) ) ;
#62793=VECTOR ( 'NONE', #83150, 1000.000000000000000 ) ;
#62798=CARTESIAN_POINT ( 'NONE',  ( 93.91125933621934507, -111.8737466215629013, -21.78219314458179667 ) ) ;
#62805=EDGE_CURVE ( 'NONE', #87042, #75851, #39510, .T. ) ;
#62807=EDGE_CURVE ( 'NONE', #9127, #16335, #19067, .T. ) ;
#62811=CARTESIAN_POINT ( 'NONE',  ( 70.71519666489237466, -139.3982827360871113, 247.4032816585904868 ) ) ;
#62824=CARTESIAN_POINT ( 'NONE',  ( 68.69398407924357741, -139.3018529721033474, 245.7655250590126457 ) ) ;
#62826=CARTESIAN_POINT ( 'NONE',  ( 82.56670390244703128, -104.2784471599409670, 22.21780685541800082 ) ) ;
#62828=FACE_OUTER_BOUND ( 'NONE', #61256, .T. ) ;
#62836=CARTESIAN_POINT ( 'NONE',  ( 89.44289600121260264, -125.4749327540683197, 250.2178068554180470 ) ) ;
#62848=ORIENTED_EDGE ( 'NONE', *, *, #16873, .F. ) ;
#62851=ORIENTED_EDGE ( 'NONE', *, *, #64532, .T. ) ;
#62853=DIRECTION ( 'NONE',  ( -0.8944271909999158554, -1.475804865149861278E-14, -0.4472135954999579277 ) ) ;
#62867=CARTESIAN_POINT ( 'NONE',  ( 128.5446125969798459, -121.5356829788754709, 250.2178068554179333 ) ) ;
#62874=CARTESIAN_POINT ( 'NONE',  ( 121.2221484686747459, -113.6057974291316839, -19.26696060647573105 ) ) ;
#62875=CARTESIAN_POINT ( 'NONE',  ( 67.15160367789934526, -67.95867621982013418, 246.0731502186970090 ) ) ;
#62880=CARTESIAN_POINT ( 'NONE',  ( 143.5667039024469886, -68.87844715994090450, 222.2178068554179902 ) ) ;
#62885=CIRCLE ( 'NONE', #20814, 3.499999999999996003 ) ;
#62895=EDGE_LOOP ( 'NONE', ( #2032, #88348 ) ) ;
#62905=VECTOR ( 'NONE', #69936, 1000.000000000000000 ) ;
#62909=ORIENTED_EDGE ( 'NONE', *, *, #46780, .F. ) ;
#62921=EDGE_LOOP ( 'NONE', ( #11247, #5792, #1336, #6520 ) ) ;
#62924=ORIENTED_EDGE ( 'NONE', *, *, #20893, .T. ) ;
#62931=LINE ( 'NONE', #71120, #65950 ) ;
#62935=DIRECTION ( 'NONE',  ( 1.000000000000000000, 0.000000000000000000, 0.000000000000000000 ) ) ;
#62960=DIRECTION ( 'NONE',  ( 1.000000000000000000, 1.000000000000000078E-15, 0.000000000000000000 ) ) ;
#62961=( BOUNDED_CURVE ( )  B_SPLINE_CURVE ( 3, ( #27114, #5783, #25762, #81652 ),
 .UNSPECIFIED., .F., .T. ) 
 B_SPLINE_CURVE_WITH_KNOTS ( ( 4, 4 ),
 ( 2.671434693666587812, 3.611750613512999308 ),
 .UNSPECIFIED. ) 
 CURVE ( )  GEOMETRIC_REPRESENTATION_ITEM ( )  RATIONAL_B_SPLINE_CURVE ( ( 1.000000000000000000, 0.9276644927932375939, 0.9276644927932375939, 1.000000000000000000 ) ) 
 REPRESENTATION_ITEM ( '' )  );
#62972=VERTEX_POINT ( 'NONE', #68117 ) ;
#62986=DIRECTION ( 'NONE',  ( 0.000000000000000000, 0.000000000000000000, -1.000000000000000000 ) ) ;
#62998=ORIENTED_EDGE ( 'NONE', *, *, #25970, .T. ) ;
#63013=DIRECTION ( 'NONE',  ( 0.8660254037844392627, -0.4999999999999990008, 1.549999999999999706E-14 ) ) ;
#63026=EDGE_CURVE ( 'NONE', #10101, #59400, #54957, .T. ) ;
#63048=CARTESIAN_POINT ( 'NONE',  ( 82.00856307258283096, -104.2784471599412370, 7.717806855417980394 ) ) ;
#63062=DIRECTION ( 'NONE',  ( 0.8660254037844382635, 0.5000000000000008882, -1.550000000000000022E-14 ) ) ;
#63073=DIRECTION ( 'NONE',  ( 0.8660254037844392627, -0.4999999999999990008, 1.549999999999999706E-14 ) ) ;
#63076=DIRECTION ( 'NONE',  ( -1.000000000000000000, -1.541976423090496028E-15, 0.000000000000000000 ) ) ;
#63093=ORIENTED_EDGE ( 'NONE', *, *, #86056, .F. ) ;
#63109=EDGE_CURVE ( 'NONE', #39484, #40328, #14419, .T. ) ;
#63116=DIRECTION ( 'NONE',  ( -1.000000000000000078E-15, 1.000000000000000000, 0.000000000000000000 ) ) ;
#63120=CARTESIAN_POINT ( 'NONE',  ( 122.2221484686747459, -111.8737466215628018, -19.26696060647578435 ) ) ;
#63121=DIRECTION ( 'NONE',  ( 0.000000000000000000, 0.000000000000000000, -1.000000000000000000 ) ) ;
#63153=VECTOR ( 'NONE', #59026, 1000.000000000000000 ) ;
#63167=LINE ( 'NONE', #64523, #36324 ) ;
#63169=EDGE_CURVE ( 'NONE', #89450, #33892, #71707, .T. ) ;
#63170=CARTESIAN_POINT ( 'NONE',  ( 67.06670390244707392, -137.6758869494786950, 245.5072624240089851 ) ) ;
#63186=VECTOR ( 'NONE', #58493, 1000.000000000000000 ) ;
#63192=DIRECTION ( 'NONE',  ( 1.000000000000000078E-15, -1.000000000000000000, 0.000000000000000000 ) ) ;
#63204=CARTESIAN_POINT ( 'NONE',  ( 99.51799851144259890, -77.76606036807547184, 250.2178068554180470 ) ) ;
#63207=CARTESIAN_POINT ( 'NONE',  ( 67.03432561829117731, -137.6460688757851756, 245.8354721159570033 ) ) ;
#63212=AXIS2_PLACEMENT_3D ( 'NONE', #11311, #66722, #31301 ) ;
#63214=CARTESIAN_POINT ( 'NONE',  ( 145.3728389244185450, -136.8603515927981107, 247.4879652615099985 ) ) ;
#63216=VECTOR ( 'NONE', #4271, 1000.000000000000000 ) ;
#63227=ORIENTED_EDGE ( 'NONE', *, *, #89462, .F. ) ;
#63271=CARTESIAN_POINT ( 'NONE',  ( 70.88111044991026688, -139.0101909505960691, 247.5112285516309782 ) ) ;
#63272=CIRCLE ( 'NONE', #89415, 2.999999999999975131 ) ;
#63281=( NAMED_UNIT ( * ) SI_UNIT ( $, .STERADIAN. ) SOLID_ANGLE_UNIT ( ) );
#63284=CARTESIAN_POINT ( 'NONE',  ( 68.69238985301161904, -139.3031226333023938, 245.7154487659484232 ) ) ;
#63315=DIRECTION ( 'NONE',  ( -1.000000000000000000, -1.541976423090496028E-15, 0.000000000000000000 ) ) ;
#63319=CARTESIAN_POINT ( 'NONE',  ( 95.56670390244703128, -104.2784471599408818, 19.21780685541799016 ) ) ;
#63341=EDGE_CURVE ( 'NONE', #75352, #44089, #48886, .T. ) ;
#63374=CARTESIAN_POINT ( 'NONE',  ( 107.0667039024470313, -104.2784471599413791, 2.217806855418003043 ) ) ;
#63377=CARTESIAN_POINT ( 'NONE',  ( 90.06670420047028358, -137.6784471599409585, 55.21780685541800437 ) ) ;
#63380=ORIENTED_EDGE ( 'NONE', *, *, #45791, .T. ) ;
#63387=ORIENTED_EDGE ( 'NONE', *, *, #64532, .F. ) ;
#63411=CYLINDRICAL_SURFACE ( 'NONE', #48630, 30.99999999999998579 ) ;
#63419=ORIENTED_EDGE ( 'NONE', *, *, #79357, .F. ) ;
#63429=VERTEX_POINT ( 'NONE', #56612 ) ;
#63455=VERTEX_POINT ( 'NONE', #89820 ) ;
#63456=ORIENTED_EDGE ( 'NONE', *, *, #84152, .F. ) ;
#63457=EDGE_CURVE ( 'NONE', #65259, #61997, #34831, .T. ) ;
#63466=CARTESIAN_POINT ( 'NONE',  ( 107.5667039024470313, -109.0284471599420613, -19.78219314458187839 ) ) ;
#63474=DIRECTION ( 'NONE',  ( 1.000000000000000000, 1.000000000000000078E-15, 0.000000000000000000 ) ) ;
#63478=VERTEX_POINT ( 'NONE', #10261 ) ;
#63480=AXIS2_PLACEMENT_3D ( 'NONE', #25715, #14677, #84173 ) ;
#63485=VECTOR ( 'NONE', #3641, 1000.000000000000000 ) ;
#63501=DIRECTION ( 'NONE',  ( 0.000000000000000000, 0.000000000000000000, 1.000000000000000000 ) ) ;
#63520=ORIENTED_EDGE ( 'NONE', *, *, #27758, .T. ) ;
#63534=EDGE_LOOP ( 'NONE', ( #34302, #66480, #56033, #33756 ) ) ;
#63547=EDGE_LOOP ( 'NONE', ( #14675, #42759, #29258, #47260, #1585, #49550 ) ) ;
#63569=EDGE_CURVE ( 'NONE', #3381, #74492, #64614, .T. ) ;
#63577=EDGE_CURVE ( 'NONE', #45437, #52825, #86963, .T. ) ;
#63618=VERTEX_POINT ( 'NONE', #84184 ) ;
#63622=CARTESIAN_POINT ( 'NONE',  ( 67.06674209438934042, -104.4391121967051816, 246.0899098363300084 ) ) ;
#63624=CARTESIAN_POINT ( 'NONE',  ( 110.2536356736639220, -106.6957733451320394, 2.217806855418086087 ) ) ;
#63646=CARTESIAN_POINT ( 'NONE',  ( 108.0667039024470171, -87.35579742913172652, -21.78219314458254630 ) ) ;
#63654=VERTEX_POINT ( 'NONE', #56893 ) ;
#63658=CARTESIAN_POINT ( 'NONE',  ( 110.8821949118856622, -76.97768462775962917, 250.2178068554180470 ) ) ;
#63660=EDGE_CURVE ( 'NONE', #85940, #22487, #84632, .T. ) ;
#63675=CARTESIAN_POINT ( 'NONE',  ( 107.0667039024470313, -104.2784471599420755, -19.78219314458201694 ) ) ;
#63685=LINE ( 'NONE', #15994, #12864 ) ;
#63686=EDGE_CURVE ( 'NONE', #11403, #26317, #71721, .T. ) ;
#63696=AXIS2_PLACEMENT_3D ( 'NONE', #50499, #9186, #8746 ) ;
#63701=VECTOR ( 'NONE', #22139, 1000.000000000000000 ) ;
#63711=ORIENTED_EDGE ( 'NONE', *, *, #9191, .F. ) ;
#63715=VECTOR ( 'NONE', #25844, 1000.000000000000000 ) ;
#63722=ORIENTED_EDGE ( 'NONE', *, *, #86849, .F. ) ;
#63725=CARTESIAN_POINT ( 'NONE',  ( 70.81267823946878082, -139.1710219483943263, 247.4769279846591701 ) ) ;
#63737=PLANE ( 'NONE',  #79645 ) ;
#63751=DIRECTION ( 'NONE',  ( 1.000000000000000000, 1.000000000000000078E-15, 0.000000000000000000 ) ) ;
#63764=ADVANCED_FACE ( 'NONE', ( #33987 ), #74893, .T. ) ;
#63768=ORIENTED_EDGE ( 'NONE', *, *, #78733, .T. ) ;
#63783=CARTESIAN_POINT ( 'NONE',  ( 131.3470363009685968, -117.3006669637343293, 250.2178068554179902 ) ) ;
#63785=CYLINDRICAL_SURFACE ( 'NONE', #18693, 3.000000000000002665 ) ;
#63789=FACE_OUTER_BOUND ( 'NONE', #40825, .T. ) ;
#63806=ORIENTED_EDGE ( 'NONE', *, *, #42027, .F. ) ;
#63810=LINE ( 'NONE', #22041, #40408 ) ;
#63836=DIRECTION ( 'NONE',  ( -3.100000000000000258E-29, 3.100000000000000044E-14, 1.000000000000000000 ) ) ;
#63852=FACE_OUTER_BOUND ( 'NONE', #70498, .T. ) ;
#63854=CARTESIAN_POINT ( 'NONE',  ( 91.91125933621933086, -104.2784471599418339, -11.78219314458200984 ) ) ;
#63855=AXIS2_PLACEMENT_3D ( 'NONE', #3843, #51963, #10213 ) ;
#63861=CARTESIAN_POINT ( 'NONE',  ( 145.6753386997136488, -136.9877269832281002, 247.4404324032252021 ) ) ;
#63863=EDGE_LOOP ( 'NONE', ( #42343, #4049, #47649, #25509 ) ) ;
#63875=DIRECTION ( 'NONE',  ( 0.000000000000000000, 0.000000000000000000, 1.000000000000000000 ) ) ;
#63894=ORIENTED_EDGE ( 'NONE', *, *, #35992, .F. ) ;
#63897=CARTESIAN_POINT ( 'NONE',  ( 92.81551872686561921, -95.01002112898675023, -19.18411693322930134 ) ) ;
#63906=ORIENTED_EDGE ( 'NONE', *, *, #20963, .F. ) ;
#63907=DIRECTION ( 'NONE',  ( 0.000000000000000000, 0.000000000000000000, -1.000000000000000000 ) ) ;
#63919=ORIENTED_EDGE ( 'NONE', *, *, #5030, .T. ) ;
#63963=EDGE_CURVE ( 'NONE', #71994, #67598, #43931, .T. ) ;
#63978=ORIENTED_EDGE ( 'NONE', *, *, #58690, .T. ) ;
#63982=CARTESIAN_POINT ( 'NONE',  ( 91.91125933621933086, -96.68314769832139177, -21.78219314458224076 ) ) ;
#63985=EDGE_CURVE ( 'NONE', #47787, #62972, #17328, .T. ) ;
#63987=AXIS2_PLACEMENT_3D ( 'NONE', #32555, #33014, #81644 ) ;
#63990=LINE ( 'NONE', #30800, #63186 ) ;
#64031=CARTESIAN_POINT ( 'NONE',  ( 68.91040501423763942, -69.55594750570173801, 247.4992607834631997 ) ) ;
#64057=ORIENTED_EDGE ( 'NONE', *, *, #2013, .F. ) ;
#64061=CARTESIAN_POINT ( 'NONE',  ( 107.0667039024470313, -104.2784471599420897, -20.48315503890502143 ) ) ;
#64083=DIRECTION ( 'NONE',  ( 0.8660254037844392627, -0.4999999999999990008, 1.549999999999999706E-14 ) ) ;
#64102=CARTESIAN_POINT ( 'NONE',  ( 86.72755763596094880, -122.7870702624433221, 249.2178068554179902 ) ) ;
#64121=DIRECTION ( 'NONE',  ( 0.000000000000000000, 0.000000000000000000, 1.000000000000000000 ) ) ;
#64150=DIRECTION ( 'NONE',  ( 0.5000000000000015543, -0.8660254037844377084, 2.688821387764056676E-14 ) ) ;
#64153=AXIS2_PLACEMENT_3D ( 'NONE', #5647, #61479, #54644 ) ;
#64177=DIRECTION ( 'NONE',  ( 1.000000000000000078E-15, -1.000000000000000000, 0.000000000000000000 ) ) ;
#64179=CARTESIAN_POINT ( 'NONE',  ( 70.64051057348294194, -139.5687525891779899, 247.3260285211522103 ) ) ;
#64196=VECTOR ( 'NONE', #41094, 1000.000000000000000 ) ;
#64209=ORIENTED_EDGE ( 'NONE', *, *, #83917, .F. ) ;
#64228=CARTESIAN_POINT ( 'NONE',  ( 132.1035770464692405, -115.7792181415380099, 250.2178068554179902 ) ) ;
#64230=DIRECTION ( 'NONE',  ( -0.000000000000000000, -0.000000000000000000, -1.000000000000000000 ) ) ;
#64233=CARTESIAN_POINT ( 'NONE',  ( 106.5667039024470455, -113.7784471599420613, -19.78219314458171141 ) ) ;
#64249=EDGE_CURVE ( 'NONE', #34414, #35902, #68864, .T. ) ;
#64260=PLANE ( 'NONE',  #31834 ) ;
#64276=ADVANCED_FACE ( 'NONE', ( #41140, #34332 ), #27523, .F. ) ;
#64285=CARTESIAN_POINT ( 'NONE',  ( 76.16940679758155852, -115.1634909102945841, 249.3055308415380011 ) ) ;
#64303=DIRECTION ( 'NONE',  ( -1.000000000000000078E-15, 1.000000000000000000, -3.100000000000000044E-14 ) ) ;
#64308=CARTESIAN_POINT ( 'NONE',  ( 145.3728389244185450, -136.8603515927981107, 247.4879652615099985 ) ) ;
#64310=EDGE_LOOP ( 'NONE', ( #33640, #69179, #17665, #28920, #17196, #71429 ) ) ;
#64316=EDGE_CURVE ( 'NONE', #47689, #5461, #60675, .T. ) ;
#64360=VERTEX_POINT ( 'NONE', #41582 ) ;
#64384=DIRECTION ( 'NONE',  ( -3.100000000000000258E-29, 3.100000000000000044E-14, 1.000000000000000000 ) ) ;
#64398=DIRECTION ( 'NONE',  ( 1.000000000000000078E-15, -1.000000000000000000, 0.000000000000000000 ) ) ;
#64459=CARTESIAN_POINT ( 'NONE',  ( 59.56670390244700997, -79.67844715994098692, 190.2178068554179902 ) ) ;
#64482=AXIS2_PLACEMENT_3D ( 'NONE', #14810, #15703, #8438 ) ;
#64489=VECTOR ( 'NONE', #51451, 1000.000000000000000 ) ;
#64494=CARTESIAN_POINT ( 'NONE',  ( 144.1872586526515647, -138.0587248278176844, 247.6570847665630026 ) ) ;
#64497=FACE_BOUND ( 'NONE', #45400, .T. ) ;
#64507=LINE ( 'NONE', #22736, #59356 ) ;
#64516=ORIENTED_EDGE ( 'NONE', *, *, #15058, .F. ) ;
#64523=CARTESIAN_POINT ( 'NONE',  ( 99.08946256649485917, -109.4614598618343138, -19.78219314458184996 ) ) ;
#64525=EDGE_CURVE ( 'NONE', #34621, #31568, #52835, .T. ) ;
#64528=ORIENTED_EDGE ( 'NONE', *, *, #52590, .F. ) ;
#64530=CIRCLE ( 'NONE', #4993, 7.999999999999992895 ) ;
#64532=EDGE_CURVE ( 'NONE', #55038, #36478, #40585, .T. ) ;
#64533=CARTESIAN_POINT ( 'NONE',  ( 52.06670390244700286, -77.67844715994100113, 55.21780685541800437 ) ) ;
#64556=CARTESIAN_POINT ( 'NONE',  ( 143.5667039024469886, -67.87844715994090450, 96.96780685541800437 ) ) ;
#64557=EDGE_CURVE ( 'NONE', #65511, #22487, #23425, .T. ) ;
#64558=DIRECTION ( 'NONE',  ( -1.000000000000000078E-15, 1.000000000000000000, 0.000000000000000000 ) ) ;
#64589=ORIENTED_EDGE ( 'NONE', *, *, #79850, .T. ) ;
#64606=DIRECTION ( 'NONE',  ( 1.000000000000000078E-15, -1.000000000000000000, 0.000000000000000000 ) ) ;
#64614=LINE ( 'NONE', #7855, #42007 ) ;
#64617=CARTESIAN_POINT ( 'NONE',  ( 63.06670390244699576, -67.87844715994098976, 85.21780685541799016 ) ) ;
#64624=CARTESIAN_POINT ( 'NONE',  ( 68.91268721346291670, -139.0876414149588527, 246.7345552620604678 ) ) ;
#64630=DIRECTION ( 'NONE',  ( -1.000000000000000078E-15, 1.000000000000000000, 0.000000000000000000 ) ) ;
#64644=DIRECTION ( 'NONE',  ( -3.100000000000000258E-29, 3.100000000000000044E-14, 1.000000000000000000 ) ) ;
#64649=ORIENTED_EDGE ( 'NONE', *, *, #63341, .F. ) ;
#64672=LINE ( 'NONE', #9265, #11612 ) ;
#64691=AXIS2_PLACEMENT_3D ( 'NONE', #32685, #81755, #60831 ) ;
#64714=ORIENTED_EDGE ( 'NONE', *, *, #4873, .F. ) ;
#64722=CARTESIAN_POINT ( 'NONE',  ( 86.74776510736894863, -122.7922775461496627, 250.2190963482990185 ) ) ;
#64726=CIRCLE ( 'NONE', #37172, 17.00000000000000000 ) ;
#64727=AXIS2_PLACEMENT_3D ( 'NONE', #74728, #26570, #59733 ) ;
#64739=CARTESIAN_POINT ( 'NONE',  ( 147.0667039024469886, -67.87844716047348470, 245.4920193514540188 ) ) ;
#64741=DIRECTION ( 'NONE',  ( 1.000000000000000000, 0.000000000000000000, 0.000000000000000000 ) ) ;
#64742=DIRECTION ( 'NONE',  ( 0.07779791923983175872, 0.07779791925944627706, 0.9939290555773350189 ) ) ;
#64760=AXIS2_PLACEMENT_3D ( 'NONE', #51560, #66085, #65647 ) ;
#64761=ADVANCED_FACE ( 'NONE', ( #71010 ), #63737, .F. ) ;
#64779=ADVANCED_FACE ( 'NONE', ( #85983 ), #86865, .T. ) ;
#64794=CARTESIAN_POINT ( 'NONE',  ( 86.72755763596092038, -85.76982405743865456, 250.2178068554179902 ) ) ;
#64818=ORIENTED_EDGE ( 'NONE', *, *, #86409, .F. ) ;
#64828=ORIENTED_EDGE ( 'NONE', *, *, #79349, .T. ) ;
#64849=CARTESIAN_POINT ( 'NONE',  ( 107.5667039024470455, -113.2645475377471058, 2.217806855418280598 ) ) ;
#64852=CARTESIAN_POINT ( 'NONE',  ( 140.0667039024470455, -118.2784471599408960, 51.21780685541800437 ) ) ;
#64854=VERTEX_POINT ( 'NONE', #85092 ) ;
#64855=AXIS2_PLACEMENT_3D ( 'NONE', #83871, #77049, #14829 ) ;
#64856=CARTESIAN_POINT ( 'NONE',  ( 162.0667039024470171, -77.67844715994088745, 222.2178068554179902 ) ) ;
#64867=AXIS2_PLACEMENT_3D ( 'NONE', #85157, #15205, #8394 ) ;
#64877=DIRECTION ( 'NONE',  ( -0.7071067811865477948, 0.7071067811865473507, 0.000000000000000000 ) ) ;
#64878=EDGE_CURVE ( 'NONE', #701, #1745, #21615, .T. ) ;
#64885=EDGE_LOOP ( 'NONE', ( #55636, #54609 ) ) ;
#64907=ORIENTED_EDGE ( 'NONE', *, *, #65488, .T. ) ;
#64914=DIRECTION ( 'NONE',  ( -0.000000000000000000, -0.000000000000000000, 1.000000000000000000 ) ) ;
#64917=CARTESIAN_POINT ( 'NONE',  ( 68.89066010437798582, -69.53878131779040928, 247.4962434065126331 ) ) ;
#64928=VERTEX_POINT ( 'NONE', #68210 ) ;
#64933=CARTESIAN_POINT ( 'NONE',  ( 145.0437226634070669, -139.7014121172837804, 246.0198185477100026 ) ) ;
#64960=CARTESIAN_POINT ( 'NONE',  ( 137.0667039024470739, -118.2784471599408960, 222.2178068554179902 ) ) ;
#64966=DIRECTION ( 'NONE',  ( -1.000000000000000000, -8.953411488912552682E-16, 0.000000000000000000 ) ) ;
#64988=ORIENTED_EDGE ( 'NONE', *, *, #7998, .T. ) ;
#65000=VECTOR ( 'NONE', #39677, 1000.000000000000000 ) ;
#65001=PLANE ( 'NONE',  #45691 ) ;
#65015=CARTESIAN_POINT ( 'NONE',  ( 98.58946256649485917, -108.5954344580498514, -19.78219314458187839 ) ) ;
#65034=VERTEX_POINT ( 'NONE', #81415 ) ;
#65037=DIRECTION ( 'NONE',  ( -1.000000000000000078E-15, 1.000000000000000000, 0.000000000000000000 ) ) ;
#65040=FACE_BOUND ( 'NONE', #9872, .T. ) ;
#65053=DIRECTION ( 'NONE',  ( -1.000000000000000000, -8.163404592832032979E-16, 0.000000000000000000 ) ) ;
#65057=AXIS2_PLACEMENT_3D ( 'NONE', #6809, #69044, #76304 ) ;
#65063=ORIENTED_EDGE ( 'NONE', *, *, #79757, .F. ) ;
#65074=CARTESIAN_POINT ( 'NONE',  ( 69.76189330943638822, -138.2438803413000130, 247.6262417895221120 ) ) ;
#65079=DIRECTION ( 'NONE',  ( -0.7071067811865503483, -0.7071067811865445751, 0.000000000000000000 ) ) ;
#65104=CARTESIAN_POINT ( 'NONE',  ( 106.5667039024470313, -108.2470741265389620, -19.78219314458190681 ) ) ;
#65126=CARTESIAN_POINT ( 'NONE',  ( 89.65393875053220540, -82.56959722164945958, 250.2201230397200220 ) ) ;
#65133=ADVANCED_FACE ( 'NONE', ( #52736 ), #12806, .F. ) ;
#65145=ORIENTED_EDGE ( 'NONE', *, *, #89908, .T. ) ;
#65148=DIRECTION ( 'NONE',  ( -0.7967329428042217998, 0.6043315462976631691, -1.875669758399923617E-14 ) ) ;
#65162=CARTESIAN_POINT ( 'NONE',  ( 84.13799348605135719, -119.9310939662431537, 250.2190963482990185 ) ) ;
#65170=VECTOR ( 'NONE', #4447, 1000.000000000000000 ) ;
#65176=EDGE_CURVE ( 'NONE', #36821, #11860, #69551, .T. ) ;
#65211=ADVANCED_FACE ( 'NONE', ( #57 ), #503, .T. ) ;
#65219=CARTESIAN_POINT ( 'NONE',  ( 147.0667039024470171, -79.67844715994090166, 222.2178068554179902 ) ) ;
#65223=CONICAL_SURFACE ( 'NONE', #46317, 16.25000000000000000, 0.5235987755982992597 ) ;
#65248=VECTOR ( 'NONE', #35721, 1000.000000000000000 ) ;
#65249=CARTESIAN_POINT ( 'NONE',  ( 107.0667039024470313, -104.2784471599409528, 45.21780685541799727 ) ) ;
#65258=ORIENTED_EDGE ( 'NONE', *, *, #119, .T. ) ;
#65259=VERTEX_POINT ( 'NONE', #42271 ) ;
#65273=VERTEX_POINT ( 'NONE', #49531 ) ;
#65311=DIRECTION ( 'NONE',  ( -1.000000000000000000, 0.000000000000000000, 0.000000000000000000 ) ) ;
#65344=( BOUNDED_CURVE ( )  B_SPLINE_CURVE ( 2, ( #37474, #42925, #8894 ),
 .UNSPECIFIED., .F., .F. ) 
 B_SPLINE_CURVE_WITH_KNOTS ( ( 3, 3 ),
 ( 0.01169420784673960018, 0.5170228498526590055 ),
 .UNSPECIFIED. ) 
 CURVE ( )  GEOMETRIC_REPRESENTATION_ITEM ( )  RATIONAL_B_SPLINE_CURVE ( ( 1.000420656333759872, 1.009299002520659849, 1.000000000000000000 ) ) 
 REPRESENTATION_ITEM ( '' )  );
#65359=CARTESIAN_POINT ( 'NONE',  ( 94.87702571208245672, -114.7407331754002229, -21.02845593540777003 ) ) ;
#65360=DIRECTION ( 'NONE',  ( 1.000000000000000078E-15, -1.000000000000000000, 0.000000000000000000 ) ) ;
#65391=DIRECTION ( 'NONE',  ( 3.100000000000000258E-29, -3.100000000000000044E-14, -1.000000000000000000 ) ) ;
#65414=LINE ( 'NONE', #31774, #68288 ) ;
#65444=AXIS2_PLACEMENT_3D ( 'NONE', #50303, #7644, #36245 ) ;
#65452=LINE ( 'NONE', #79547, #69078 ) ;
#65468=CARTESIAN_POINT ( 'NONE',  ( 75.91207007020635444, -69.50612193463149424, 247.5400045958994042 ) ) ;
#65472=VECTOR ( 'NONE', #87501, 999.9999999999998863 ) ;
#65488=EDGE_CURVE ( 'NONE', #71019, #75012, #47522, .T. ) ;
#65500=AXIS2_PLACEMENT_3D ( 'NONE', #63377, #8883, #49736 ) ;
#65511=VERTEX_POINT ( 'NONE', #89342 ) ;
#65516=DIRECTION ( 'NONE',  ( 0.000000000000000000, 0.000000000000000000, 1.000000000000000000 ) ) ;
#65529=CIRCLE ( 'NONE', #9017, 11.49999999999999645 ) ;
#65536=ORIENTED_EDGE ( 'NONE', *, *, #134, .T. ) ;
#65538=VERTEX_POINT ( 'NONE', #88893 ) ;
#65540=DIRECTION ( 'NONE',  ( 0.000000000000000000, 0.000000000000000000, 1.000000000000000000 ) ) ;
#65546=FACE_OUTER_BOUND ( 'NONE', #70744, .T. ) ;
#65549=CARTESIAN_POINT ( 'NONE',  ( 145.9684219307273452, -136.2709667195323959, 247.3967439480269945 ) ) ;
#65553=ORIENTED_EDGE ( 'NONE', *, *, #72788, .T. ) ;
#65574=CARTESIAN_POINT ( 'NONE',  ( 127.5395909587422949, -72.61999453823881367, 248.4067532124560103 ) ) ;
#65575=CARTESIAN_POINT ( 'NONE',  ( 146.4947614284610609, -68.42932138493740979, 246.8950229379430539 ) ) ;
#65576=DIRECTION ( 'NONE',  ( 3.100000000000000258E-29, -3.100000000000000044E-14, -1.000000000000000000 ) ) ;
#65590=VERTEX_POINT ( 'NONE', #26645 ) ;
#65597=CIRCLE ( 'NONE', #69952, 32.50000000000001421 ) ;
#65606=DIRECTION ( 'NONE',  ( 3.100000000000000258E-29, -3.100000000000000044E-14, -1.000000000000000000 ) ) ;
#65619=CARTESIAN_POINT ( 'NONE',  ( 143.6448735140314454, -139.9068108329578308, 247.1123908456728486 ) ) ;
#65632=CYLINDRICAL_SURFACE ( 'NONE', #53847, 7.999999999999992895 ) ;
#65647=DIRECTION ( 'NONE',  ( 1.000000000000000000, 0.000000000000000000, 0.000000000000000000 ) ) ;
#65648=ORIENTED_EDGE ( 'NONE', *, *, #18600, .T. ) ;
#65681=FACE_OUTER_BOUND ( 'NONE', #47402, .T. ) ;
#65691=VERTEX_POINT ( 'NONE', #70681 ) ;
#65696=AXIS2_PLACEMENT_3D ( 'NONE', #59713, #3879, #5678 ) ;
#65742=ADVANCED_FACE ( 'NONE', ( #84330 ), #50668, .T. ) ;
#65751=DIRECTION ( 'NONE',  ( -3.100000000000000258E-29, 3.100000000000000044E-14, 1.000000000000000000 ) ) ;
#65754=EDGE_LOOP ( 'NONE', ( #67481, #22053, #53898, #24472 ) ) ;
#65775=VECTOR ( 'NONE', #36100, 1000.000000000000000 ) ;
#65800=AXIS2_PLACEMENT_3D ( 'NONE', #4051, #52608, #30871 ) ;
#65811=EDGE_CURVE ( 'NONE', #82359, #68139, #46060, .T. ) ;
#65842=DIRECTION ( 'NONE',  ( 0.8660254037844380415, 0.5000000000000012212, -1.550000000000001284E-14 ) ) ;
#65844=CARTESIAN_POINT ( 'NONE',  ( 56.06670390244699576, -67.87844715994098976, 120.2178068554179902 ) ) ;
#65858=DIRECTION ( 'NONE',  ( -3.100000000000000258E-29, 3.100000000000000044E-14, 1.000000000000000000 ) ) ;
#65864=EDGE_CURVE ( 'NONE', #41538, #76165, #32005, .T. ) ;
#65875=VERTEX_POINT ( 'NONE', #10667 ) ;
#65880=ADVANCED_FACE ( 'NONE', ( #86992 ), #45608, .T. ) ;
#65890=AXIS2_PLACEMENT_3D ( 'NONE', #86974, #52836, #18359 ) ;
#65906=DIRECTION ( 'NONE',  ( 0.000000000000000000, 0.000000000000000000, -1.000000000000000000 ) ) ;
#65937=CARTESIAN_POINT ( 'NONE',  ( 147.0667039024469886, -67.87844715994090450, 222.2178068554179902 ) ) ;
#65945=EDGE_LOOP ( 'NONE', ( #60149, #75115, #82447, #79569, #70540 ) ) ;
#65947=CIRCLE ( 'NONE', #61607, 15.50000000000000000 ) ;
#65950=VECTOR ( 'NONE', #70209, 1000.000000000000000 ) ;
#65952=CARTESIAN_POINT ( 'NONE',  ( 68.74877429598565470, -139.2496317701004784, 246.2158363995229706 ) ) ;
#65965=ORIENTED_EDGE ( 'NONE', *, *, #20893, .F. ) ;
#65979=CARTESIAN_POINT ( 'NONE',  ( 119.2563820928116343, -93.81616114448401333, -21.02845593540860492 ) ) ;
#65993=PLANE ( 'NONE',  #62630 ) ;
#66000=ORIENTED_EDGE ( 'NONE', *, *, #49367, .F. ) ;
#66002=PLANE ( 'NONE',  #61853 ) ;
#66009=AXIS2_PLACEMENT_3D ( 'NONE', #27571, #5794, #47989 ) ;
#66012=LINE ( 'NONE', #74188, #13954 ) ;
#66015=EDGE_LOOP ( 'NONE', ( #73843, #11760, #14627, #13169 ) ) ;
#66049=CARTESIAN_POINT ( 'NONE',  ( 131.5667039024470455, -104.2784471599409244, 23.21780685541800082 ) ) ;
#66053=CARTESIAN_POINT ( 'NONE',  ( 143.5298718395760602, -139.6521136699046792, 247.2811342184976695 ) ) ;
#66059=CARTESIAN_POINT ( 'NONE',  ( 85.06670390244700286, -71.37844715994096134, 222.2178068554179902 ) ) ;
#66065=ORIENTED_EDGE ( 'NONE', *, *, #16917, .T. ) ;
#66072=DIRECTION ( 'NONE',  ( 1.000000000000000000, 1.000000000000000078E-15, 0.000000000000000000 ) ) ;
#66080=ORIENTED_EDGE ( 'NONE', *, *, #3551, .T. ) ;
#66085=DIRECTION ( 'NONE',  ( 0.000000000000000000, 0.000000000000000000, 1.000000000000000000 ) ) ;
#66091=AXIS2_PLACEMENT_3D ( 'NONE', #58283, #16514, #37851 ) ;
#66095=VECTOR ( 'NONE', #22221, 999.9999999999998863 ) ;
#66124=ORIENTED_EDGE ( 'NONE', *, *, #14142, .T. ) ;
#66130=DIRECTION ( 'NONE',  ( 0.000000000000000000, 0.000000000000000000, 1.000000000000000000 ) ) ;
#66143=CARTESIAN_POINT ( 'NONE',  ( 91.91125933621951560, -96.57698625956682292, -11.78219314458225853 ) ) ;
#66152=CARTESIAN_POINT ( 'NONE',  ( 91.91229609755362162, -96.60849280716382737, -19.21046202161324956 ) ) ;
#66157=FACE_OUTER_BOUND ( 'NONE', #79222, .T. ) ;
#66162=CARTESIAN_POINT ( 'NONE',  ( 99.08946256649487339, -99.09543445804985140, -19.78219314458218392 ) ) ;
#66182=LINE ( 'NONE', #59370, #26234 ) ;
#66193=CARTESIAN_POINT ( 'NONE',  ( 68.58297366894557001, -139.1947169264394688, 246.0943807925750093 ) ) ;
#66194=CIRCLE ( 'NONE', #89438, 29.49999999999998579 ) ;
#66208=EDGE_CURVE ( 'NONE', #10101, #44089, #15157, .T. ) ;
#66223=CARTESIAN_POINT ( 'NONE',  ( 143.5667039024469886, -68.87844715994090450, 222.2178068554179902 ) ) ;
#66235=CIRCLE ( 'NONE', #75010, 17.00000000000000000 ) ;
#66238=DIRECTION ( 'NONE',  ( -3.100000000000000258E-29, 3.100000000000000044E-14, 1.000000000000000000 ) ) ;
#66241=ORIENTED_EDGE ( 'NONE', *, *, #20140, .T. ) ;
#66243=ADVANCED_FACE ( 'NONE', ( #42833 ), #27877, .T. ) ;
#66258=AXIS2_PLACEMENT_3D ( 'NONE', #52245, #16430, #44106 ) ;
#66262=LINE ( 'NONE', #79488, #41408 ) ;
#66265=CARTESIAN_POINT ( 'NONE',  ( 121.2862831202667167, -94.98932219798427923, -19.21046202161327798 ) ) ;
#66288=AXIS2_PLACEMENT_3D ( 'NONE', #79033, #53051, #23627 ) ;
#66300=DIRECTION ( 'NONE',  ( 0.000000000000000000, 0.000000000000000000, 1.000000000000000000 ) ) ;
#66308=EDGE_LOOP ( 'NONE', ( #62026, #24607, #68485, #62476, #69834, #1504, #19397 ) ) ;
#66343=CARTESIAN_POINT ( 'NONE',  ( 70.06670417066791856, -83.77844715994098124, 55.21780685541800437 ) ) ;
#66381=EDGE_LOOP ( 'NONE', ( #81197, #46806, #68033, #85579 ) ) ;
#66384=CARTESIAN_POINT ( 'NONE',  ( 70.06670390244705970, -124.7784471599409812, 55.21780685541800437 ) ) ;
#66390=DIRECTION ( 'NONE',  ( 1.000000000000000078E-15, -1.000000000000000000, 0.000000000000000000 ) ) ;
#66392=AXIS2_PLACEMENT_3D ( 'NONE', #17836, #86887, #51446 ) ;
#66397=CARTESIAN_POINT ( 'NONE',  ( 68.96108109926477425, -139.0395986478499708, 246.8356254435167614 ) ) ;
#66409=AXIS2_PLACEMENT_3D ( 'NONE', #89379, #88929, #81678 ) ;
#66416=VERTEX_POINT ( 'NONE', #45499 ) ;
#66421=ORIENTED_EDGE ( 'NONE', *, *, #20873, .F. ) ;
#66426=DIRECTION ( 'NONE',  ( 1.000000000000000000, 1.000000000000000078E-15, 0.000000000000000000 ) ) ;
#66480=ORIENTED_EDGE ( 'NONE', *, *, #28038, .T. ) ;
#66494=EDGE_CURVE ( 'NONE', #86558, #50049, #40049, .T. ) ;
#66498=EDGE_CURVE ( 'NONE', #22506, #54510, #36315, .T. ) ;
#66506=CARTESIAN_POINT ( 'NONE',  ( 143.9181536748402266, -140.4668907707514052, 246.4376387225517533 ) ) ;
#66514=CARTESIAN_POINT ( 'NONE',  ( 67.85198242736144891, -137.2567436070751796, 247.0961534730330982 ) ) ;
#66530=CARTESIAN_POINT ( 'NONE',  ( 70.06670390244703128, -96.32844715994099261, 55.21780685541800437 ) ) ;
#66534=EDGE_LOOP ( 'NONE', ( #17640, #66124, #14806, #18825 ) ) ;
#66555=CARTESIAN_POINT ( 'NONE',  ( 107.0667039024470313, -104.2784471599413791, 2.217806855418003043 ) ) ;
#66556=VECTOR ( 'NONE', #45361, 1000.000000000000000 ) ;
#66566=DIRECTION ( 'NONE',  ( -3.100000000000000258E-29, 3.100000000000000044E-14, 1.000000000000000000 ) ) ;
#66570=DIRECTION ( 'NONE',  ( 0.8660254037844380415, 0.5000000000000012212, -1.550000000000001284E-14 ) ) ;
#66574=ORIENTED_EDGE ( 'NONE', *, *, #70347, .F. ) ;
#66579=CARTESIAN_POINT ( 'NONE',  ( 122.2221484686747317, -96.68314769832130651, -19.26696060647622843 ) ) ;
#66595=LINE ( 'NONE', #52926, #2559 ) ;
#66607=ORIENTED_EDGE ( 'NONE', *, *, #61878, .F. ) ;
#66621=CARTESIAN_POINT ( 'NONE',  ( 107.0667039024470313, -104.2784471599409528, 22.21780685541800082 ) ) ;
#66623=ORIENTED_EDGE ( 'NONE', *, *, #53536, .F. ) ;
#66630=VERTEX_POINT ( 'NONE', #84102 ) ;
#66648=CARTESIAN_POINT ( 'NONE',  ( 112.3595036205099689, -139.4350393735792579, 247.7272646988739950 ) ) ;
#66651=CARTESIAN_POINT ( 'NONE',  ( 69.08968514148706674, -139.7014121172838657, 246.0198185477100026 ) ) ;
#66679=VECTOR ( 'NONE', #35224, 1000.000000000000000 ) ;
#66682=CARTESIAN_POINT ( 'NONE',  ( 67.06670390244701707, -79.67844715994098692, 180.4678068554179902 ) ) ;
#66691=CARTESIAN_POINT ( 'NONE',  ( 132.2857443282839824, -83.77844715994092439, 55.21780685541800437 ) ) ;
#66692=CARTESIAN_POINT ( 'NONE',  ( 107.0667039024470313, -104.2784471599409528, 24.21780685541800082 ) ) ;
#66722=DIRECTION ( 'NONE',  ( -3.100000000000000258E-29, 3.100000000000000044E-14, 1.000000000000000000 ) ) ;
#66764=DIRECTION ( 'NONE',  ( 1.000000000000000000, 0.000000000000000000, 0.000000000000000000 ) ) ;
#66781=DIRECTION ( 'NONE',  ( 1.000000000000000078E-15, -1.000000000000000000, 0.000000000000000000 ) ) ;
#66833=DIRECTION ( 'NONE',  ( 0.000000000000000000, -1.000000000000000000, 0.000000000000000000 ) ) ;
#66839=ORIENTED_EDGE ( 'NONE', *, *, #43620, .T. ) ;
#66842=FACE_OUTER_BOUND ( 'NONE', #10348, .T. ) ;
#66850=ORIENTED_EDGE ( 'NONE', *, *, #23571, .F. ) ;
#66855=FACE_OUTER_BOUND ( 'NONE', #13156, .T. ) ;
#66860=CIRCLE ( 'NONE', #84400, 3.500000000000003109 ) ;
#66868=DIRECTION ( 'NONE',  ( -0.9217329428042198014, -0.3878251953515564066, 1.203464411458912131E-14 ) ) ;
#66901=B_SPLINE_SURFACE_WITH_KNOTS ( 'NONE', 3, 3, ( 
 ( #39581, #62721, #42705, #70444, #6863 ),
 ( #15031, #41809, #69546, #498, #14132 ),
 ( #15491, #83629, #35910, #49973, #1857 ),
 ( #8219, #69097, #63622, #49525, #20943 ),
 ( #63170, #1409, #70902, #41364, #69994 ) ),
 .UNSPECIFIED., .F., .F., .F.,
 ( 4, 1, 4 ),
 ( 4, 1, 4 ),
 ( 0.000000000000000000, 0.5714285714285709528, 1.000000000000000000 ),
 ( 0.1438910682813560049, 3.135239217345689777, 7.123703416098150498 ),
 .UNSPECIFIED. ) ;
#66903=ORIENTED_EDGE ( 'NONE', *, *, #76441, .T. ) ;
#66906=AXIS2_PLACEMENT_3D ( 'NONE', #51466, #77866, #23799 ) ;
#66921=VERTEX_POINT ( 'NONE', #40834 ) ;
#66927=AXIS2_PLACEMENT_3D ( 'NONE', #24302, #9330, #51531 ) ;
#66964=LINE ( 'NONE', #74675, #85891 ) ;
#66968=DIRECTION ( 'NONE',  ( 1.000000000000000000, 1.000000000000000078E-15, -0.000000000000000000 ) ) ;
#66969=DIRECTION ( 'NONE',  ( 1.000000000000000000, 1.000000000000000078E-15, 0.000000000000000000 ) ) ;
#66980=DIRECTION ( 'NONE',  ( -3.100000000000000258E-29, 3.100000000000000044E-14, 1.000000000000000000 ) ) ;
#66982=DIRECTION ( 'NONE',  ( 1.000000000000000000, 0.000000000000000000, 0.000000000000000000 ) ) ;
#66995=CARTESIAN_POINT ( 'NONE',  ( 68.06670390244704549, -114.5284471599409812, 55.21780685541800437 ) ) ;
#66998=ADVANCED_FACE ( 'NONE', ( #75377 ), #11808, .F. ) ;
#67003=DIRECTION ( 'NONE',  ( -1.000000000000000000, -1.734723475976808672E-15, 0.000000000000000000 ) ) ;
#67011=CARTESIAN_POINT ( 'NONE',  ( 67.06803888862225449, -67.87902570666702218, 245.5599109093815002 ) ) ;
#67027=CARTESIAN_POINT ( 'NONE',  ( 84.19170390244700286, -68.87844715994097555, 138.7178068554180186 ) ) ;
#67043=VERTEX_POINT ( 'NONE', #7232 ) ;
#67053=VERTEX_POINT ( 'NONE', #62178 ) ;
#67056=ORIENTED_EDGE ( 'NONE', *, *, #70705, .T. ) ;
#67070=CARTESIAN_POINT ( 'NONE',  ( 98.58946256649487339, -99.96145986183361742, 2.217806855417864043 ) ) ;
#67099=CARTESIAN_POINT ( 'NONE',  ( 112.3589615562450774, -139.8532878908926307, 247.5529029630430102 ) ) ;
#67102=CARTESIAN_POINT ( 'NONE',  ( 98.06670390244704549, -104.2784471599414076, 2.217806855418003043 ) ) ;
#67104=VERTEX_POINT ( 'NONE', #70803 ) ;
#67112=ADVANCED_FACE ( 'NONE', ( #83100 ), #8122, .T. ) ;
#67139=CARTESIAN_POINT ( 'NONE',  ( 81.84766347661002328, -83.77844715994098124, 222.2178068554179902 ) ) ;
#67159=LINE ( 'NONE', #17681, #66556 ) ;
#67168=CARTESIAN_POINT ( 'NONE',  ( 107.0667039024469886, -67.87844715994094713, 173.2178068554179902 ) ) ;
#67177=DIRECTION ( 'NONE',  ( -3.100000000000000258E-29, 3.100000000000000044E-14, 1.000000000000000000 ) ) ;
#67178=EDGE_LOOP ( 'NONE', ( #14526, #46281, #11245, #20036 ) ) ;
#67188=LINE ( 'NONE', #4971, #22774 ) ;
#67194=CIRCLE ( 'NONE', #59917, 2.000000000000001776 ) ;
#67220=ORIENTED_EDGE ( 'NONE', *, *, #26154, .T. ) ;
#67229=VECTOR ( 'NONE', #34991, 1000.000000000000000 ) ;
#67247=DIRECTION ( 'NONE',  ( 1.000000000000000000, 0.000000000000000000, 0.000000000000000000 ) ) ;
#67274=LINE ( 'NONE', #80477, #2215 ) ;
#67283=CARTESIAN_POINT ( 'NONE',  ( 147.0667039024469886, -67.87844715994090450, 222.2178068554179902 ) ) ;
#67285=DIRECTION ( 'NONE',  ( 3.100000000000000258E-29, -3.100000000000000044E-14, -1.000000000000000000 ) ) ;
#67286=CARTESIAN_POINT ( 'NONE',  ( 123.5302891131021710, -139.7352204321790339, 247.5112265945679724 ) ) ;
#67289=CARTESIAN_POINT ( 'NONE',  ( 116.3167039024470029, -68.87844715994093292, 222.2178068554179902 ) ) ;
#67300=CARTESIAN_POINT ( 'NONE',  ( 147.0664286958740945, -101.1139857980062118, 246.2087142436340059 ) ) ;
#67310=AXIS2_PLACEMENT_3D ( 'NONE', #53037, #5382, #33081 ) ;
#67312=EDGE_LOOP ( 'NONE', ( #9856, #75370, #87374, #56803 ) ) ;
#67315=ORIENTED_EDGE ( 'NONE', *, *, #78534, .F. ) ;
#67344=CYLINDRICAL_SURFACE ( 'NONE', #8468, 7.999999999999992895 ) ;
#67350=FACE_OUTER_BOUND ( 'NONE', #8777, .T. ) ;
#67362=VERTEX_POINT ( 'NONE', #2209 ) ;
#67385=ORIENTED_EDGE ( 'NONE', *, *, #53750, .F. ) ;
#67406=CARTESIAN_POINT ( 'NONE',  ( 107.0667039024470313, -104.2784471599420755, -19.78219314458201694 ) ) ;
#67435=FACE_OUTER_BOUND ( 'NONE', #71692, .T. ) ;
#67440=ORIENTED_EDGE ( 'NONE', *, *, #63686, .F. ) ;
#67448=CARTESIAN_POINT ( 'NONE',  ( 74.06670390244701707, -90.27844715994098124, 51.21780685541800437 ) ) ;
#67481=ORIENTED_EDGE ( 'NONE', *, *, #11813, .F. ) ;
#67508=CARTESIAN_POINT ( 'NONE',  ( 124.0667039024470313, -101.5893827172045860, -9.937637710810113489 ) ) ;
#67509=EDGE_CURVE ( 'NONE', #38678, #89615, #38897, .T. ) ;
#67510=CARTESIAN_POINT ( 'NONE',  ( 107.0667039024470313, -104.2784471599409528, 23.21780685541800082 ) ) ;
#67540=ADVANCED_FACE ( 'NONE', ( #87112 ), #81654, .F. ) ;
#67598=VERTEX_POINT ( 'NONE', #75718 ) ;
#67603=FACE_OUTER_BOUND ( 'NONE', #80798, .T. ) ;
#67621=LINE ( 'NONE', #45369, #63715 ) ;
#67644=CARTESIAN_POINT ( 'NONE',  ( 107.0667039024470313, -104.2784471599413934, 2.217806855418003043 ) ) ;
#67650=AXIS2_PLACEMENT_3D ( 'NONE', #77639, #52022, #37972 ) ;
#67652=VECTOR ( 'NONE', #35844, 1000.000000000000114 ) ;
#67678=FACE_OUTER_BOUND ( 'NONE', #20889, .T. ) ;
#67707=AXIS2_PLACEMENT_3D ( 'NONE', #73784, #66968, #53307 ) ;
#67711=ORIENTED_EDGE ( 'NONE', *, *, #36164, .F. ) ;
#67726=CIRCLE ( 'NONE', #28560, 4.500000000000003553 ) ;
#67727=CARTESIAN_POINT ( 'NONE',  ( 107.9747653995834327, -87.30271670975442078, -11.78219314458253741 ) ) ;
#67730=CARTESIAN_POINT ( 'NONE',  ( 107.5667039024470171, -94.77844715994206126, -19.78219314458232247 ) ) ;
#67738=CARTESIAN_POINT ( 'NONE',  ( 86.74776500631861609, -85.76461670310806085, 250.2190963482990185 ) ) ;
#67740=EDGE_CURVE ( 'NONE', #56065, #59400, #20149, .T. ) ;
#67755=FACE_OUTER_BOUND ( 'NONE', #85022, .T. ) ;
#67756=DIRECTION ( 'NONE',  ( -3.100000000000000258E-29, 3.100000000000000044E-14, 1.000000000000000000 ) ) ;
#67807=DIRECTION ( 'NONE',  ( 0.8660254037844389297, -0.4999999999999993894, 1.550000000000000968E-14 ) ) ;
#67834=LINE ( 'NONE', #61015, #74829 ) ;
#67841=LINE ( 'NONE', #12433, #59403 ) ;
#67844=ORIENTED_EDGE ( 'NONE', *, *, #69690, .F. ) ;
#67846=ORIENTED_EDGE ( 'NONE', *, *, #29814, .T. ) ;
#67855=FILL_AREA_STYLE_COLOUR ( '', #21776 ) ;
#67866=PLANE ( 'NONE',  #76804 ) ;
#67873=CARTESIAN_POINT ( 'NONE',  ( 74.06670390244701707, -90.27844715994098124, 51.21780685541800437 ) ) ;
#67879=VECTOR ( 'NONE', #49945, 1000.000000000000000 ) ;
#67885=VERTEX_POINT ( 'NONE', #2737 ) ;
#67920=LINE ( 'NONE', #24800, #76461 ) ;
#67950=CARTESIAN_POINT ( 'NONE',  ( 106.0667039024470171, -87.35579742913164125, -19.26696060647653397 ) ) ;
#67951=ORIENTED_EDGE ( 'NONE', *, *, #80428, .T. ) ;
#67965=CARTESIAN_POINT ( 'NONE',  ( 122.2221484686745185, -96.57698625956679450, -11.78219314458225853 ) ) ;
#67969=DIRECTION ( 'NONE',  ( 1.000000000000000078E-15, -1.000000000000000000, 0.000000000000000000 ) ) ;
#67983=CARTESIAN_POINT ( 'NONE',  ( 144.0667039024470739, -137.6784471599409017, 222.2178068554179902 ) ) ;
#67997=ORIENTED_EDGE ( 'NONE', *, *, #72995, .T. ) ;
#68021=DIRECTION ( 'NONE',  ( -1.000000000000000078E-15, 1.000000000000000000, -3.100000000000000044E-14 ) ) ;
#68030=VECTOR ( 'NONE', #76318, 1000.000000000000000 ) ;
#68033=ORIENTED_EDGE ( 'NONE', *, *, #74615, .T. ) ;
#68046=PLANE ( 'NONE',  #4805 ) ;
#68055=CARTESIAN_POINT ( 'NONE',  ( 115.5439452383992176, -108.5954344580498372, -19.78219314458187839 ) ) ;
#68064=ORIENTED_EDGE ( 'NONE', *, *, #62, .T. ) ;
#68069=CARTESIAN_POINT ( 'NONE',  ( 107.0667039024470313, -104.2784471599409528, 23.21780685541800082 ) ) ;
#68085=DIRECTION ( 'NONE',  ( -0.7396053187813123042, -0.6730408400909958511, 0.000000000000000000 ) ) ;
#68111=CIRCLE ( 'NONE', #49292, 3.499999999999996003 ) ;
#68117=CARTESIAN_POINT ( 'NONE',  ( 95.56670390244703128, -104.2784471599414644, 0.2178068554180012661 ) ) ;
#68129=EDGE_LOOP ( 'NONE', ( #56988, #56972 ) ) ;
#68135=EDGE_CURVE ( 'NONE', #74274, #82155, #14230, .T. ) ;
#68139=VERTEX_POINT ( 'NONE', #79492 ) ;
#68152=DIRECTION ( 'NONE',  ( 0.000000000000000000, 0.000000000000000000, 1.000000000000000000 ) ) ;
#68182=ORIENTED_EDGE ( 'NONE', *, *, #32048, .T. ) ;
#68187=FACE_OUTER_BOUND ( 'NONE', #66308, .T. ) ;
#68199=VERTEX_POINT ( 'NONE', #52007 ) ;
#68210=CARTESIAN_POINT ( 'NONE',  ( 71.06670390244705970, -118.2784471599409812, 51.21780685541800437 ) ) ;
#68218=CARTESIAN_POINT ( 'NONE',  ( 147.0663630288289880, -77.84642232681920859, 246.0747600069850023 ) ) ;
#68260=FACE_OUTER_BOUND ( 'NONE', #63863, .T. ) ;
#68264=ORIENTED_EDGE ( 'NONE', *, *, #63569, .T. ) ;
#68272=DIRECTION ( 'NONE',  ( 3.100000000000000258E-29, -3.100000000000000044E-14, -1.000000000000000000 ) ) ;
#68283=CARTESIAN_POINT ( 'NONE',  ( 59.56670390244700997, -79.67844715994098692, 120.2178068554179902 ) ) ;
#68288=VECTOR ( 'NONE', #30891, 1000.000000000000000 ) ;
#68334=CYLINDRICAL_SURFACE ( 'NONE', #76112, 3.499999999999996003 ) ;
#68355=PLANE ( 'NONE',  #23955 ) ;
#68362=FACE_OUTER_BOUND ( 'NONE', #85281, .T. ) ;
#68372=EDGE_CURVE ( 'NONE', #28990, #41770, #80654, .T. ) ;
#68378=ORIENTED_EDGE ( 'NONE', *, *, #58519, .F. ) ;
#68393=ORIENTED_EDGE ( 'NONE', *, *, #77579, .F. ) ;
#68416=AXIS2_PLACEMENT_3D ( 'NONE', #3965, #11219, #38924 ) ;
#68424=CARTESIAN_POINT ( 'NONE',  ( 116.3167039024470029, -67.87844715994093292, 55.21780685541800437 ) ) ;
#68428=ORIENTED_EDGE ( 'NONE', *, *, #17855, .T. ) ;
#68443=DIRECTION ( 'NONE',  ( 1.000000000000000000, 1.000000000000000078E-15, 0.000000000000000000 ) ) ;
#68454=CARTESIAN_POINT ( 'NONE',  ( 87.68258360185966183, -140.6784122025596560, 246.0580355273719988 ) ) ;
#68458=CIRCLE ( 'NONE', #82997, 2.000000000000007550 ) ;
#68477=CARTESIAN_POINT ( 'NONE',  ( 132.1248447323112316, -104.2784471599408818, 17.71780685541799016 ) ) ;
#68485=ORIENTED_EDGE ( 'NONE', *, *, #5605, .T. ) ;
#68486=EDGE_CURVE ( 'NONE', #60056, #75262, #40346, .T. ) ;
#68502=CARTESIAN_POINT ( 'NONE',  ( 110.2536356736639220, -106.6957733451320394, 2.217806855418086087 ) ) ;
#68507=ORIENTED_EDGE ( 'NONE', *, *, #69862, .T. ) ;
#68523=DIRECTION ( 'NONE',  ( 1.000000000000000000, 0.000000000000000000, 0.000000000000000000 ) ) ;
#68525=LINE ( 'NONE', #21267, #2777 ) ;
#68548=EDGE_CURVE ( 'NONE', #40328, #65691, #46164, .T. ) ;
#68560=EDGE_CURVE ( 'NONE', #17136, #15221, #25895, .T. ) ;
#68567=EDGE_CURVE ( 'NONE', #67053, #67104, #47409, .T. ) ;
#68594=CARTESIAN_POINT ( 'NONE',  ( 144.5667039024470455, -118.2784471599408960, 45.21780685541799727 ) ) ;
#68597=VERTEX_POINT ( 'NONE', #83330 ) ;
#68629=CARTESIAN_POINT ( 'NONE',  ( 121.3140869715381314, -95.00417761012944595, -11.78219314458228695 ) ) ;
#68639=ORIENTED_EDGE ( 'NONE', *, *, #25390, .F. ) ;
#68648=CARTESIAN_POINT ( 'NONE',  ( 119.2077814229834729, -133.9288653316829141, 249.3173333679100097 ) ) ;
#68654=ADVANCED_FACE ( 'NONE', ( #645 ), #63785, .F. ) ;
#68656=DIRECTION ( 'NONE',  ( 0.8660254037844380415, 0.5000000000000012212, -1.550000000000001284E-14 ) ) ;
#68661=ADVANCED_FACE ( 'NONE', ( #56499 ), #21105, .T. ) ;
#68692=DIRECTION ( 'NONE',  ( 0.000000000000000000, 0.000000000000000000, -1.000000000000000000 ) ) ;
#68699=AXIS2_PLACEMENT_3D ( 'NONE', #52761, #11476, #17838 ) ;
#68700=FACE_OUTER_BOUND ( 'NONE', #17015, .T. ) ;
#68728=ORIENTED_EDGE ( 'NONE', *, *, #10140, .F. ) ;
#68750=ORIENTED_EDGE ( 'NONE', *, *, #53013, .T. ) ;
#68757=DIRECTION ( 'NONE',  ( 0.000000000000000000, 0.000000000000000000, 1.000000000000000000 ) ) ;
#68763=LINE ( 'NONE', #74676, #17832 ) ;
#68766=EDGE_CURVE ( 'NONE', #45547, #75555, #24233, .T. ) ;
#68798=ORIENTED_EDGE ( 'NONE', *, *, #31826, .T. ) ;
#68805=DIRECTION ( 'NONE',  ( -1.000000000000000078E-15, 1.000000000000000000, 0.000000000000000000 ) ) ;
#68809=CARTESIAN_POINT ( 'NONE',  ( 67.99030470749720223, -68.76354271653610795, 247.1802073626070353 ) ) ;
#68825=VERTEX_POINT ( 'NONE', #4227 ) ;
#68830=CARTESIAN_POINT ( 'NONE',  ( 52.56670390244699576, -68.37844715994100397, 55.21780685541800437 ) ) ;
#68836=DIRECTION ( 'NONE',  ( 1.777766061779359009E-15, -1.000000000000000000, 3.100000000000000044E-14 ) ) ;
#68864=LINE ( 'NONE', #67070, #31701 ) ;
#68873=LINE ( 'NONE', #48848, #2218 ) ;
#68909=ORIENTED_EDGE ( 'NONE', *, *, #10429, .T. ) ;
#68927=FACE_OUTER_BOUND ( 'NONE', #19935, .T. ) ;
#68968=CYLINDRICAL_SURFACE ( 'NONE', #33025, 2.999999999999975131 ) ;
#68979=LINE ( 'NONE', #21736, #87477 ) ;
#68981=CYLINDRICAL_SURFACE ( 'NONE', #22451, 4.000000000000002665 ) ;
#68999=VERTEX_POINT ( 'NONE', #5120 ) ;
#69008=ORIENTED_EDGE ( 'NONE', *, *, #18600, .F. ) ;
#69009=VECTOR ( 'NONE', #83114, 999.9999999999998863 ) ;
#69027=DIRECTION ( 'NONE',  ( -0.5000000000000069944, 0.8660254037844344888, -2.684678751731748934E-14 ) ) ;
#69031=AXIS2_PLACEMENT_3D ( 'NONE', #75921, #47747, #6874 ) ;
#69033=DIRECTION ( 'NONE',  ( -3.100000000000000258E-29, 3.100000000000000044E-14, 1.000000000000000000 ) ) ;
#69044=DIRECTION ( 'NONE',  ( -3.100000000000000258E-29, 3.100000000000000044E-14, 1.000000000000000000 ) ) ;
#69049=FACE_OUTER_BOUND ( 'NONE', #20974, .T. ) ;
#69065=EDGE_CURVE ( 'NONE', #60002, #45648, #56415, .T. ) ;
#69069=EDGE_CURVE ( 'NONE', #68999, #14487, #24477, .T. ) ;
#69078=VECTOR ( 'NONE', #85024, 1000.000000000000000 ) ;
#69090=CARTESIAN_POINT ( 'NONE',  ( 107.5667039024470455, -112.2628068712777036, -19.78219314458176825 ) ) ;
#69091=EDGE_CURVE ( 'NONE', #37650, #75315, #62195, .T. ) ;
#69097=CARTESIAN_POINT ( 'NONE',  ( 67.06680637612726059, -127.7071673695392917, 245.9559769091540034 ) ) ;
#69105=CARTESIAN_POINT ( 'NONE',  ( 68.77377604071689632, -69.45229246467815187, 247.4784000562319761 ) ) ;
#69121=ORIENTED_EDGE ( 'NONE', *, *, #70705, .F. ) ;
#69123=DIRECTION ( 'NONE',  ( -1.000000000000000000, -1.734723475976808672E-15, 0.000000000000000000 ) ) ;
#69134=VERTEX_POINT ( 'NONE', #24457 ) ;
#69151=ORIENTED_EDGE ( 'NONE', *, *, #25886, .T. ) ;
#69163=ORIENTED_EDGE ( 'NONE', *, *, #78959, .T. ) ;
#69175=ORIENTED_EDGE ( 'NONE', *, *, #41903, .T. ) ;
#69179=ORIENTED_EDGE ( 'NONE', *, *, #56380, .T. ) ;
#69199=CIRCLE ( 'NONE', #61921, 3.500000000000003109 ) ;
#69214=DIRECTION ( 'NONE',  ( -3.100000000000000258E-29, 3.100000000000000044E-14, 1.000000000000000000 ) ) ;
#69230=CARTESIAN_POINT ( 'NONE',  ( 116.0667039024470313, -104.2784471599413791, 2.217806855418003043 ) ) ;
#69232=B_SPLINE_CURVE_WITH_KNOTS ( 'NONE', 3,
 ( #5649, #61038, #19710, #88769 ),
 .UNSPECIFIED., .F., .F.,
 ( 4, 4 ),
 ( -0.6035999334370369951, -0.5903216970416030884 ),
 .UNSPECIFIED. ) ;
#69246=AXIS2_PLACEMENT_3D ( 'NONE', #81082, #80183, #17497 ) ;
#69249=CYLINDRICAL_SURFACE ( 'NONE', #15332, 3.000000864267367895 ) ;
#69293=EDGE_LOOP ( 'NONE', ( #55171, #19243 ) ) ;
#69345=ORIENTED_EDGE ( 'NONE', *, *, #53019, .T. ) ;
#69351=CARTESIAN_POINT ( 'NONE',  ( 145.2008403534674699, -139.0679250929170792, 246.7780077290963163 ) ) ;
#69390=EDGE_CURVE ( 'NONE', #46470, #6854, #43884, .T. ) ;
#69393=DIRECTION ( 'NONE',  ( 1.000000000000000000, 5.440892098500631367E-15, -1.376676550535195643E-28 ) ) ;
#69400=ADVANCED_FACE ( 'NONE', ( #83911 ), #56622, .T. ) ;
#69432=DIRECTION ( 'NONE',  ( -1.150535366796005147E-15, 1.000000000000000000, -3.100000000000000044E-14 ) ) ;
#69442=CIRCLE ( 'NONE', #34606, 17.00000000000000000 ) ;
#69445=VERTEX_POINT ( 'NONE', #36650 ) ;
#69463=EDGE_CURVE ( 'NONE', #64854, #29557, #22577, .T. ) ;
#69482=CARTESIAN_POINT ( 'NONE',  ( 107.0667039024470313, -104.2784471599420755, -19.78219314458201694 ) ) ;
#69495=DIRECTION ( 'NONE',  ( 1.000000000000000078E-15, -1.000000000000000000, 0.000000000000000000 ) ) ;
#69508=ORIENTED_EDGE ( 'NONE', *, *, #78534, .T. ) ;
#69511=EDGE_CURVE ( 'NONE', #2874, #79206, #12736, .T. ) ;
#69546=CARTESIAN_POINT ( 'NONE',  ( 68.02453369492833701, -104.4395081749008796, 247.5031975998799965 ) ) ;
#69550=( LENGTH_UNIT ( ) NAMED_UNIT ( * ) SI_UNIT ( .MILLI., .METRE. ) );
#69551=LINE ( 'NONE', #42711, #34751 ) ;
#69558=DIRECTION ( 'NONE',  ( -3.100000000000000258E-29, 3.100000000000000044E-14, 1.000000000000000000 ) ) ;
#69561=ORIENTED_EDGE ( 'NONE', *, *, #80991, .T. ) ;
#69581=CARTESIAN_POINT ( 'NONE',  ( 68.37671137566576363, -137.2574698224148904, 247.4285129581799936 ) ) ;
#69591=CARTESIAN_POINT ( 'NONE',  ( 147.0667039024457665, -137.6758868153238780, 245.5072646551060132 ) ) ;
#69652=CARTESIAN_POINT ( 'NONE',  ( 117.0667039024470313, -104.2784471599412086, 7.717806855417980394 ) ) ;
#69654=CARTESIAN_POINT ( 'NONE',  ( 68.69272960418753371, -139.3028697034590664, 245.7287393302975147 ) ) ;
#69656=CARTESIAN_POINT ( 'NONE',  ( 143.0667039024470171, -118.2784471599408960, 51.21780685541800437 ) ) ;
#69664=CARTESIAN_POINT ( 'NONE',  ( 88.01156830653452801, -124.1980709993373750, 250.2178068554179333 ) ) ;
#69672=DIRECTION ( 'NONE',  ( 1.000000000000000000, 3.555032108465730541E-16, 0.000000000000000000 ) ) ;
#69687=LINE ( 'NONE', #36516, #77714 ) ;
#69690=EDGE_CURVE ( 'NONE', #36508, #19483, #8399, .T. ) ;
#69700=CARTESIAN_POINT ( 'NONE',  ( 127.4058501689331280, -122.7870702624433221, 250.2178068554179902 ) ) ;
#69705=DIRECTION ( 'NONE',  ( -1.000000000000000000, -1.000000000000000078E-15, 0.000000000000000000 ) ) ;
#69717=CARTESIAN_POINT ( 'NONE',  ( 145.8234706062852979, -69.06773314681258569, 247.3490213069128458 ) ) ;
#69721=DIRECTION ( 'NONE',  ( 3.100000000000000258E-29, -3.100000000000000044E-14, -1.000000000000000000 ) ) ;
#69726=AXIS2_PLACEMENT_3D ( 'NONE', #23187, #55852, #2273 ) ;
#69738=ORIENTED_EDGE ( 'NONE', *, *, #24101, .T. ) ;
#69752=ORIENTED_EDGE ( 'NONE', *, *, #58987, .T. ) ;
#69775=VECTOR ( 'NONE', #29381, 1000.000000000000000 ) ;
#69784=DIRECTION ( 'NONE',  ( 1.000000000000000000, 1.000000000000000078E-15, 0.000000000000000000 ) ) ;
#69795=VECTOR ( 'NONE', #64384, 1000.000000000000000 ) ;
#69797=VERTEX_POINT ( 'NONE', #83797 ) ;
#69801=DIRECTION ( 'NONE',  ( -1.150535366796005147E-15, 1.000000000000000000, -3.100000000000000044E-14 ) ) ;
#69816=EDGE_CURVE ( 'NONE', #87073, #1742, #14761, .T. ) ;
#69824=DIRECTION ( 'NONE',  ( 1.000000000000000078E-15, -1.000000000000000000, 0.000000000000000000 ) ) ;
#69834=ORIENTED_EDGE ( 'NONE', *, *, #49569, .T. ) ;
#69835=VECTOR ( 'NONE', #78880, 999.9999999999998863 ) ;
#69844=CYLINDRICAL_SURFACE ( 'NONE', #55577, 2.999999999999988898 ) ;
#69862=EDGE_CURVE ( 'NONE', #53716, #20346, #87320, .T. ) ;
#69863=DIRECTION ( 'NONE',  ( 1.000000000000000078E-15, -1.000000000000000000, 3.100000000000000044E-14 ) ) ;
#69866=CARTESIAN_POINT ( 'NONE',  ( 127.4058501689331280, -85.76982405743856930, 249.2178068554179902 ) ) ;
#69870=DIRECTION ( 'NONE',  ( -0.8660254037844392627, 0.4999999999999990008, -1.549999999999999706E-14 ) ) ;
#69876=AXIS2_PLACEMENT_3D ( 'NONE', #55664, #71587, #9347 ) ;
#69880=DIRECTION ( 'NONE',  ( 0.000000000000000000, 0.000000000000000000, -1.000000000000000000 ) ) ;
#69919=DIRECTION ( 'NONE',  ( -1.000000000000000078E-15, 1.000000000000000000, 0.000000000000000000 ) ) ;
#69932=CYLINDRICAL_SURFACE ( 'NONE', #17163, 3.999999999999998224 ) ;
#69936=DIRECTION ( 'NONE',  ( 0.000000000000000000, 0.000000000000000000, 1.000000000000000000 ) ) ;
#69941=DIRECTION ( 'NONE',  ( 0.000000000000000000, 0.000000000000000000, 1.000000000000000000 ) ) ;
#69952=AXIS2_PLACEMENT_3D ( 'NONE', #4365, #30725, #81133 ) ;
#69957=ORIENTED_EDGE ( 'NONE', *, *, #28661, .T. ) ;
#69959=ORIENTED_EDGE ( 'NONE', *, *, #49290, .T. ) ;
#69977=FACE_OUTER_BOUND ( 'NONE', #52917, .T. ) ;
#69980=CARTESIAN_POINT ( 'NONE',  ( 122.2221484686747459, -111.8737466215628018, -19.26696060647578435 ) ) ;
#69984=VERTEX_POINT ( 'NONE', #54143 ) ;
#69989=PRODUCT_DEFINITION ( 'UNKNOWN', '', #21763, #70549 ) ;
#69994=CARTESIAN_POINT ( 'NONE',  ( 67.06670390244700286, -67.87844715994098976, 245.4920193514479934 ) ) ;
#69995=CARTESIAN_POINT ( 'NONE',  ( 107.0667039024470313, -119.4690460831833150, -11.78219314458153733 ) ) ;
#69998=SHAPE_REPRESENTATION_RELATIONSHIP ( 'NONE' , 'NONE' ,  #14421, #3408 ) ;
#70004=ADVANCED_FACE ( 'NONE', ( #81903 ), #67344, .F. ) ;
#70005=AXIS2_PLACEMENT_3D ( 'NONE', #32573, #80307, #73463 ) ;
#70018=DIRECTION ( 'NONE',  ( -1.000000000000000078E-15, 1.000000000000000000, 0.000000000000000000 ) ) ;
#70022=ORIENTED_EDGE ( 'NONE', *, *, #79471, .F. ) ;
#70030=CARTESIAN_POINT ( 'NONE',  ( 67.62344788955067543, -138.2352025272443825, 245.9283337036430055 ) ) ;
#70073=ORIENTED_EDGE ( 'NONE', *, *, #76473, .F. ) ;
#70076=FACE_OUTER_BOUND ( 'NONE', #6778, .T. ) ;
#70105=ADVANCED_FACE ( 'NONE', ( #87258 ), #72292, .T. ) ;
#70127=DIRECTION ( 'NONE',  ( -3.100000000000000258E-29, 3.100000000000000044E-14, 1.000000000000000000 ) ) ;
#70143=CARTESIAN_POINT ( 'NONE',  ( 70.06968321367156705, -140.6784088069870222, 245.5331728854790185 ) ) ;
#70150=ORIENTED_EDGE ( 'NONE', *, *, #23655, .F. ) ;
#70181=EDGE_LOOP ( 'NONE', ( #47076, #13304 ) ) ;
#70193=FACE_OUTER_BOUND ( 'NONE', #39400, .T. ) ;
#70201=ADVANCED_FACE ( 'NONE', ( #9608 ), #51812, .F. ) ;
#70207=EDGE_CURVE ( 'NONE', #63654, #86303, #23003, .T. ) ;
#70209=DIRECTION ( 'NONE',  ( 0.000000000000000000, 0.000000000000000000, -1.000000000000000000 ) ) ;
#70210=DIRECTION ( 'NONE',  ( -1.000000000000000078E-15, 1.000000000000000000, 0.000000000000000000 ) ) ;
#70233=DIRECTION ( 'NONE',  ( 1.000000000000000000, 0.000000000000000000, 0.000000000000000000 ) ) ;
#70237=EDGE_CURVE ( 'NONE', #13431, #71967, #14224, .T. ) ;
#70250=EDGE_LOOP ( 'NONE', ( #2060, #7267, #41887, #55172, #53842, #57841, #55020, #23806 ) ) ;
#70259=DIRECTION ( 'NONE',  ( 3.100000000000000258E-29, -3.100000000000000044E-14, -1.000000000000000000 ) ) ;
#70266=CARTESIAN_POINT ( 'NONE',  ( 52.06670390244699576, -67.87844715994100397, 55.21780685541800437 ) ) ;
#70281=DIRECTION ( 'NONE',  ( -1.150535366796005147E-15, 1.000000000000000000, -3.100000000000000044E-14 ) ) ;
#70282=ORIENTED_EDGE ( 'NONE', *, *, #1503, .T. ) ;
#70287=EDGE_CURVE ( 'NONE', #4284, #29468, #59964, .T. ) ;
#70293=DIRECTION ( 'NONE',  ( 3.100000000000000258E-29, -3.100000000000000044E-14, -1.000000000000000000 ) ) ;
#70301=ORIENTED_EDGE ( 'NONE', *, *, #39839, .F. ) ;
#70319=CARTESIAN_POINT ( 'NONE',  ( 107.0667039024470313, -104.2784471599413934, 2.217806855418003043 ) ) ;
#70321=LINE ( 'NONE', #41695, #36720 ) ;
#70343=DIRECTION ( 'NONE',  ( -1.000000000000000000, -1.206764157201257538E-15, 0.000000000000000000 ) ) ;
#70347=EDGE_CURVE ( 'NONE', #26346, #57531, #8520, .T. ) ;
#70379=AXIS2_PLACEMENT_3D ( 'NONE', #19602, #80500, #25072 ) ;
#70394=AXIS2_PLACEMENT_3D ( 'NONE', #82774, #48202, #35479 ) ;
#70398=EDGE_LOOP ( 'NONE', ( #39745, #53722, #786, #68728 ) ) ;
#70403=( BOUNDED_CURVE ( )  B_SPLINE_CURVE ( 2, ( #37662, #65359, #3142 ),
 .UNSPECIFIED., .F., .T. ) 
 B_SPLINE_CURVE_WITH_KNOTS ( ( 3, 3 ),
 ( 0.000000000000000000, 0.5053286420056780637 ),
 .UNSPECIFIED. ) 
 CURVE ( )  GEOMETRIC_REPRESENTATION_ITEM ( )  RATIONAL_B_SPLINE_CURVE ( ( 1.000000000000000000, 1.009299002520649857, 1.000420656333769864 ) ) 
 REPRESENTATION_ITEM ( '' )  );
#70404=B_SPLINE_CURVE_WITH_KNOTS ( 'NONE', 3,
 ( #52158, #45355, #10413, #73075, #31289, #38553, #52599 ),
 .UNSPECIFIED., .F., .F.,
 ( 4, 1, 1, 1, 4 ),
 ( -0.1863381261298940050, 0.9565458916201099449, 3.242315181216560038, 5.528084470813009688, 7.813853433339420285 ),
 .UNSPECIFIED. ) ;
#70410=VERTEX_POINT ( 'NONE', #27255 ) ;
#70412=EDGE_CURVE ( 'NONE', #57634, #36122, #24469, .T. ) ;
#70415=CARTESIAN_POINT ( 'NONE',  ( 143.0536128999585515, -139.9914422477621088, 247.3423811826519909 ) ) ;
#70420=CARTESIAN_POINT ( 'NONE',  ( 106.1318921495875145, -121.2375349704976486, -19.21044887263748180 ) ) ;
#70444=CARTESIAN_POINT ( 'NONE',  ( 68.70813896271630483, -81.16137653295078280, 247.5270838628449894 ) ) ;
#70445=DIRECTION ( 'NONE',  ( 1.000000000000000000, 0.000000000000000000, 0.000000000000000000 ) ) ;
#70451=( LENGTH_UNIT ( ) NAMED_UNIT ( * ) SI_UNIT ( .MILLI., .METRE. ) );
#70467=CARTESIAN_POINT ( 'NONE',  ( 107.0667039024470313, -104.2784471599409528, 23.21780685541800082 ) ) ;
#70478=CARTESIAN_POINT ( 'NONE',  ( 103.3797721312301405, -102.7271463785351671, 2.217806855417947531 ) ) ;
#70484=ORIENTED_EDGE ( 'NONE', *, *, #83522, .T. ) ;
#70487=EDGE_CURVE ( 'NONE', #65273, #77074, #5, .T. ) ;
#70498=EDGE_LOOP ( 'NONE', ( #82055, #73181 ) ) ;
#70506=CYLINDRICAL_SURFACE ( 'NONE', #83281, 2.000000000000007550 ) ;
#70516=PLANE ( 'NONE',  #63696 ) ;
#70538=LINE ( 'NONE', #8307, #31051 ) ;
#70539=CARTESIAN_POINT ( 'NONE',  ( 115.5439452383992176, -108.5954344580498372, -19.78219314458187839 ) ) ;
#70540=ORIENTED_EDGE ( 'NONE', *, *, #52612, .T. ) ;
#70549=PRODUCT_DEFINITION_CONTEXT ( 'detailed design', #85250, 'design' ) ;
#70575=AXIS2_PLACEMENT_3D ( 'NONE', #56267, #6794, #8147 ) ;
#70597=CARTESIAN_POINT ( 'NONE',  ( 133.3245970085671104, -95.93364041391147623, 250.2178068554180470 ) ) ;
#70604=CARTESIAN_POINT ( 'NONE',  ( 67.34197081037864052, -68.14385895291664497, 246.5134725747785751 ) ) ;
#70610=DIRECTION ( 'NONE',  ( -0.7071067811865536790, 0.7071067811865414665, 0.000000000000000000 ) ) ;
#70612=LINE ( 'NONE', #42878, #9089 ) ;
#70614=AXIS2_PLACEMENT_3D ( 'NONE', #87593, #88047, #73506 ) ;
#70621=DIRECTION ( 'NONE',  ( -3.100000000000000258E-29, 3.100000000000000044E-14, 1.000000000000000000 ) ) ;
#70626=CARTESIAN_POINT ( 'NONE',  ( 147.0793590841609841, -69.57571276584434372, 247.4899279706389734 ) ) ;
#70642=EDGE_CURVE ( 'NONE', #86777, #46470, #7050, .T. ) ;
#70648=CARTESIAN_POINT ( 'NONE',  ( 105.5982380168385930, -102.8532777164006262, -19.78219314458207378 ) ) ;
#70655=ORIENTED_EDGE ( 'NONE', *, *, #43413, .F. ) ;
#70667=DIRECTION ( 'NONE',  ( -3.100000000000000258E-29, 3.100000000000000044E-14, 1.000000000000000000 ) ) ;
#70672=CARTESIAN_POINT ( 'NONE',  ( 147.0667039024457665, -137.6758868153238780, 245.5072646551060132 ) ) ;
#70681=CARTESIAN_POINT ( 'NONE',  ( 100.4020455594773722, -108.7036397175021136, -19.78219314458187839 ) ) ;
#70684=CARTESIAN_POINT ( 'NONE',  ( 122.2221484686746322, -104.2784471599418055, -11.78219314458200984 ) ) ;
#70689=EDGE_LOOP ( 'NONE', ( #74732, #80443, #16964, #54509, #19767, #5413, #57004, #81487, #42399, #41406, #35651, #48044 ) ) ;
#70705=EDGE_CURVE ( 'NONE', #1627, #27673, #37656, .T. ) ;
#70708=CARTESIAN_POINT ( 'NONE',  ( 68.06670390244704549, -114.5284471599409812, 45.21780685541799727 ) ) ;
#70710=CARTESIAN_POINT ( 'NONE',  ( 85.06670390244700286, -74.11757344603526576, 222.2178068554179902 ) ) ;
#70711=CARTESIAN_POINT ( 'NONE',  ( 93.91125933621933086, -96.68314769832137756, -21.78219314458224076 ) ) ;
#70722=CARTESIAN_POINT ( 'NONE',  ( 140.0667039024470171, -90.27844715994091018, 51.21780685541800437 ) ) ;
#70724=VECTOR ( 'NONE', #42135, 1000.000000000000000 ) ;
#70730=DIRECTION ( 'NONE',  ( -0.7396053187813123042, -0.6730408400909958511, 0.000000000000000000 ) ) ;
#70743=ORIENTED_EDGE ( 'NONE', *, *, #59975, .T. ) ;
#70744=EDGE_LOOP ( 'NONE', ( #24728, #31280, #40220, #48802 ) ) ;
#70756=ORIENTED_EDGE ( 'NONE', *, *, #58899, .T. ) ;
#70784=DIRECTION ( 'NONE',  ( -3.100000000000000258E-29, 3.100000000000000044E-14, 1.000000000000000000 ) ) ;
#70803=CARTESIAN_POINT ( 'NONE',  ( 70.06968321367156705, -140.6784088069870222, 245.5331728854790185 ) ) ;
#70808=VERTEX_POINT ( 'NONE', #14772 ) ;
#70817=EDGE_CURVE ( 'NONE', #88126, #86096, #63810, .T. ) ;
#70826=VECTOR ( 'NONE', #9543, 1000.000000000000000 ) ;
#70827=ORIENTED_EDGE ( 'NONE', *, *, #19869, .T. ) ;
#70844=VERTEX_POINT ( 'NONE', #8400 ) ;
#70855=LINE ( 'NONE', #57644, #24739 ) ;
#70858=ORIENTED_EDGE ( 'NONE', *, *, #3023, .F. ) ;
#70870=FACE_OUTER_BOUND ( 'NONE', #17698, .T. ) ;
#70877=ADVANCED_FACE ( 'NONE', ( #71528 ), #8857, .F. ) ;
#70895=DIRECTION ( 'NONE',  ( 1.000000000000000000, 0.000000000000000000, 0.000000000000000000 ) ) ;
#70902=CARTESIAN_POINT ( 'NONE',  ( 67.06670390244704549, -104.4390062815841844, 245.7240875270999823 ) ) ;
#70908=( NAMED_UNIT ( * ) SI_UNIT ( $, .STERADIAN. ) SOLID_ANGLE_UNIT ( ) );
#70951=CARTESIAN_POINT ( 'NONE',  ( 74.06670390244701707, -90.27844715994098124, 45.21780685541799727 ) ) ;
#70990=CIRCLE ( 'NONE', #73890, 3.000000864267343026 ) ;
#70997=DIRECTION ( 'NONE',  ( -1.000000000000000000, -8.163404592832032979E-16, 0.000000000000000000 ) ) ;
#71006=DIRECTION ( 'NONE',  ( -0.000000000000000000, -0.000000000000000000, 1.000000000000000000 ) ) ;
#71010=FACE_OUTER_BOUND ( 'NONE', #80257, .T. ) ;
#71018=CARTESIAN_POINT ( 'NONE',  ( 53.06670390244699576, -67.87844715994100397, 180.4678068554179902 ) ) ;
#71019=VERTEX_POINT ( 'NONE', #53709 ) ;
#71037=DIRECTION ( 'NONE',  ( 0.000000000000000000, 0.000000000000000000, -1.000000000000000000 ) ) ;
#71042=CARTESIAN_POINT ( 'NONE',  ( 98.06670390244705970, -124.7784471599409528, 55.21780685541800437 ) ) ;
#71047=CARTESIAN_POINT ( 'NONE',  ( 147.0990821866028568, -137.6460688757850050, 245.8354721159570033 ) ) ;
#71062=VECTOR ( 'NONE', #54857, 1000.000000000000000 ) ;
#71063=DIRECTION ( 'NONE',  ( -1.000000000000000078E-15, 1.000000000000000000, 0.000000000000000000 ) ) ;
#71081=EDGE_LOOP ( 'NONE', ( #59873, #83031, #27846, #63919 ) ) ;
#71085=EDGE_LOOP ( 'NONE', ( #78171, #77652, #6310, #4400, #77311, #45378, #81686, #66574, #63520, #8507, #46865, #27729 ) ) ;
#71091=ORIENTED_EDGE ( 'NONE', *, *, #5397, .F. ) ;
#71112=ORIENTED_EDGE ( 'NONE', *, *, #60431, .T. ) ;
#71120=CARTESIAN_POINT ( 'NONE',  ( 127.4058501689331280, -85.76982405743856930, 250.2178068554179902 ) ) ;
#71132=VERTEX_POINT ( 'NONE', #22822 ) ;
#71152=ADVANCED_FACE ( 'NONE', ( #1923 ), #70516, .F. ) ;
#71158=CARTESIAN_POINT ( 'NONE',  ( 154.5667039024470171, -79.67844715994088745, 190.2178068554179902 ) ) ;
#71159=EDGE_CURVE ( 'NONE', #20491, #31568, #75300, .T. ) ;
#71173=CARTESIAN_POINT ( 'NONE',  ( 115.0439452383991892, -99.09543445804983719, -19.78219314458218392 ) ) ;
#71195=ORIENTED_EDGE ( 'NONE', *, *, #19973, .F. ) ;
#71198=EDGE_CURVE ( 'NONE', #4290, #5461, #44570, .T. ) ;
#71213=ORIENTED_EDGE ( 'NONE', *, *, #20765, .F. ) ;
#71215=ORIENTED_EDGE ( 'NONE', *, *, #58701, .T. ) ;
#71218=DIRECTION ( 'NONE',  ( -1.000000000000000000, -1.734723475976808672E-15, 0.000000000000000000 ) ) ;
#71251=AXIS2_PLACEMENT_3D ( 'NONE', #6944, #49153, #27830 ) ;
#71269=CARTESIAN_POINT ( 'NONE',  ( 105.0982380168385930, -104.8375911996990766, -19.78219314458198852 ) ) ;
#71270=DIRECTION ( 'NONE',  ( 0.000000000000000000, 0.000000000000000000, -1.000000000000000000 ) ) ;
#71273=EDGE_CURVE ( 'NONE', #18666, #51113, #74079, .T. ) ;
#71280=DIRECTION ( 'NONE',  ( -1.000000000000000000, -8.163404592832032979E-16, 0.000000000000000000 ) ) ;
#71305=CARTESIAN_POINT ( 'NONE',  ( 71.06670390244705970, -118.2784471599409812, 230.7030882296565721 ) ) ;
#71320=FACE_OUTER_BOUND ( 'NONE', #70689, .T. ) ;
#71362=EDGE_LOOP ( 'NONE', ( #84266, #7631 ) ) ;
#71378=EDGE_CURVE ( 'NONE', #4111, #28081, #916, .T. ) ;
#71384=EDGE_CURVE ( 'NONE', #20155, #55721, #7731, .T. ) ;
#71392=CIRCLE ( 'NONE', #3171, 32.50000000000000711 ) ;
#71397=PLANE ( 'NONE',  #3842 ) ;
#71407=DIRECTION ( 'NONE',  ( 1.000000000000000000, 1.000000000000000078E-15, 0.000000000000000000 ) ) ;
#71422=DIRECTION ( 'NONE',  ( 0.000000000000000000, 0.000000000000000000, 1.000000000000000000 ) ) ;
#71429=ORIENTED_EDGE ( 'NONE', *, *, #58122, .T. ) ;
#71447=LINE ( 'NONE', #37355, #4358 ) ;
#71448=DIRECTION ( 'NONE',  ( 0.000000000000000000, 0.000000000000000000, 1.000000000000000000 ) ) ;
#71449=CARTESIAN_POINT ( 'NONE',  ( 70.62220382094542970, -139.6100950337742290, 247.3042842130787733 ) ) ;
#71461=CARTESIAN_POINT ( 'NONE',  ( 68.96471483387718138, -139.0359911094384699, 246.8427143030575337 ) ) ;
#71485=LINE ( 'NONE', #9685, #34133 ) ;
#71494=CARTESIAN_POINT ( 'NONE',  ( 145.3303304183568514, -139.4148206440309821, 246.0960064844549890 ) ) ;
#71528=FACE_OUTER_BOUND ( 'NONE', #72040, .T. ) ;
#71532=DIRECTION ( 'NONE',  ( -1.000000000000000000, 0.000000000000000000, 0.000000000000000000 ) ) ;
#71540=VECTOR ( 'NONE', #37708, 1000.000000000000000 ) ;
#71554=CARTESIAN_POINT ( 'NONE',  ( 68.77555145974430673, -69.40287493179035039, 247.4783998280180128 ) ) ;
#71571=EDGE_CURVE ( 'NONE', #24085, #56828, #86273, .T. ) ;
#71576=CARTESIAN_POINT ( 'NONE',  ( 146.4497560438693711, -137.3344668342741670, 246.9543106399991075 ) ) ;
#71587=DIRECTION ( 'NONE',  ( 0.000000000000000000, 0.000000000000000000, 1.000000000000000000 ) ) ;
#71590=AXIS2_PLACEMENT_3D ( 'NONE', #53787, #26556, #60161 ) ;
#71604=ORIENTED_EDGE ( 'NONE', *, *, #23811, .F. ) ;
#71607=DIRECTION ( 'NONE',  ( 0.000000000000000000, 0.000000000000000000, 1.000000000000000000 ) ) ;
#71611=DIRECTION ( 'NONE',  ( 1.000000000000000078E-15, -1.000000000000000000, 0.000000000000000000 ) ) ;
#71614=CARTESIAN_POINT ( 'NONE',  ( 67.06670390244700286, -67.87844716047356997, 245.4920193514540188 ) ) ;
#71623=VECTOR ( 'NONE', #46638, 1000.000000000000000 ) ;
#71630=VERTEX_POINT ( 'NONE', #63897 ) ;
#71641=EDGE_CURVE ( 'NONE', #65538, #18397, #56148, .T. ) ;
#71684=CARTESIAN_POINT ( 'NONE',  ( 111.3555650440039528, -119.3022720253473210, -21.78219314458154798 ) ) ;
#71687=ORIENTED_EDGE ( 'NONE', *, *, #63457, .T. ) ;
#71692=EDGE_LOOP ( 'NONE', ( #71744, #41569, #75821, #42230, #9621, #21758 ) ) ;
#71697=PLANE ( 'NONE',  #8391 ) ;
#71704=ORIENTED_EDGE ( 'NONE', *, *, #82116, .T. ) ;
#71707=LINE ( 'NONE', #38952, #65170 ) ;
#71716=ORIENTED_EDGE ( 'NONE', *, *, #29229, .F. ) ;
#71721=( BOUNDED_CURVE ( )  B_SPLINE_CURVE ( 2, ( #21044, #48717, #587 ),
 .UNSPECIFIED., .F., .T. ) 
 B_SPLINE_CURVE_WITH_KNOTS ( ( 3, 3 ),
 ( 0.01169420784673960018, 0.5170228498526580063 ),
 .UNSPECIFIED. ) 
 CURVE ( )  GEOMETRIC_REPRESENTATION_ITEM ( )  RATIONAL_B_SPLINE_CURVE ( ( 1.000420656333759872, 1.009299002520659849, 1.000000000000000000 ) ) 
 REPRESENTATION_ITEM ( '' )  );
#71742=PLANE ( 'NONE',  #25546 ) ;
#71744=ORIENTED_EDGE ( 'NONE', *, *, #23771, .F. ) ;
#71749=AXIS2_PLACEMENT_3D ( 'NONE', #80608, #79720, #18357 ) ;
#71768=DIRECTION ( 'NONE',  ( 3.100000000000000258E-29, -3.100000000000000044E-14, -1.000000000000000000 ) ) ;
#71772=LINE ( 'NONE', #77692, #70826 ) ;
#71819=CARTESIAN_POINT ( 'NONE',  ( 103.3797721312301405, -102.7271463785358492, -19.78219314458207378 ) ) ;
#71854=FACE_OUTER_BOUND ( 'NONE', #32307, .T. ) ;
#71855=ADVANCED_FACE ( 'NONE', ( #30184 ), #22486, .F. ) ;
#71888=CARTESIAN_POINT ( 'NONE',  ( 97.81670390244700286, -67.87844715994096134, 222.2178068554179902 ) ) ;
#71890=DIRECTION ( 'NONE',  ( -5.773159642023980606E-15, -5.773159642023980170E-30, -1.000000000000000000 ) ) ;
#71918=ORIENTED_EDGE ( 'NONE', *, *, #51843, .T. ) ;
#71922=CARTESIAN_POINT ( 'NONE',  ( 161.5667039024469886, -68.37844715994089029, 222.2178068554179902 ) ) ;
#71926=CARTESIAN_POINT ( 'NONE',  ( 68.06670390244701707, -86.77844715994098124, 55.21780685541800437 ) ) ;
#71936=CARTESIAN_POINT ( 'NONE',  ( 115.5439452383992176, -108.5954344580498372, -19.78219314458187839 ) ) ;
#71938=EDGE_CURVE ( 'NONE', #54510, #74974, #30629, .T. ) ;
#71952=EDGE_CURVE ( 'NONE', #51807, #79449, #87829, .T. ) ;
#71967=VERTEX_POINT ( 'NONE', #18779 ) ;
#71975=CARTESIAN_POINT ( 'NONE',  ( 140.0667039024470171, -90.27844715994091018, 230.7030882296565721 ) ) ;
#71994=VERTEX_POINT ( 'NONE', #31061 ) ;
#72012=CARTESIAN_POINT ( 'NONE',  ( 67.53185150639035328, -137.4071337290076826, 246.7901045206692459 ) ) ;
#72024=DIRECTION ( 'NONE',  ( 3.100000000000000258E-29, -3.100000000000000044E-14, -1.000000000000000000 ) ) ;
#72036=LINE ( 'NONE', #30692, #6257 ) ;
#72040=EDGE_LOOP ( 'NONE', ( #413, #4443, #15731, #73967 ) ) ;
#72068=EDGE_CURVE ( 'NONE', #74492, #82359, #74200, .T. ) ;
#72077=CARTESIAN_POINT ( 'NONE',  ( 85.06670390244701707, -80.35669973212957018, 55.21780685541800437 ) ) ;
#72083=ORIENTED_EDGE ( 'NONE', *, *, #46466, .F. ) ;
#72094=EDGE_LOOP ( 'NONE', ( #21508, #57039 ) ) ;
#72116=CARTESIAN_POINT ( 'NONE',  ( 77.74851419028676958, -134.1785091737438051, 248.4142799812389910 ) ) ;
#72188=AXIS2_PLACEMENT_3D ( 'NONE', #10896, #66300, #72245 ) ;
#72208=CIRCLE ( 'NONE', #21501, 30.99999999999998579 ) ;
#72216=EDGE_CURVE ( 'NONE', #27685, #39084, #24648, .T. ) ;
#72245=DIRECTION ( 'NONE',  ( 1.000000000000000000, 0.000000000000000000, 0.000000000000000000 ) ) ;
#72246=DIRECTION ( 'NONE',  ( 1.075267683398002218E-15, -1.000000000000000000, 3.100000000000000044E-14 ) ) ;
#72251=CARTESIAN_POINT ( 'NONE',  ( 67.06670390244707392, -137.6773508471079595, 245.4788304630789924 ) ) ;
#72256=( BOUNDED_CURVE ( )  B_SPLINE_CURVE ( 3, ( #25373, #9976, #37681, #46241 ),
 .UNSPECIFIED., .F., .T. ) 
 B_SPLINE_CURVE_WITH_KNOTS ( ( 4, 4 ),
 ( 2.671434693666588700, 3.141592653589793116 ),
 .UNSPECIFIED. ) 
 CURVE ( )  GEOMETRIC_REPRESENTATION_ITEM ( )  RATIONAL_B_SPLINE_CURVE ( ( 1.000000000000000000, 0.9816639655796102204, 0.9816639655796102204, 1.000000000000000000 ) ) 
 REPRESENTATION_ITEM ( '' )  );
#72259=ADVANCED_FACE ( 'NONE', ( #5613 ), #33305, .F. ) ;
#72262=VECTOR ( 'NONE', #33626, 1000.000000000000000 ) ;
#72270=CARTESIAN_POINT ( 'NONE',  ( 107.0667039024470313, -104.2784471599408676, 19.21780685541799016 ) ) ;
#72281=EDGE_CURVE ( 'NONE', #37406, #56556, #83258, .T. ) ;
#72282=DIRECTION ( 'NONE',  ( 0.000000000000000000, 0.000000000000000000, -1.000000000000000000 ) ) ;
#72284=DIRECTION ( 'NONE',  ( -3.100000000000000258E-29, 3.100000000000000044E-14, 1.000000000000000000 ) ) ;
#72287=ORIENTED_EDGE ( 'NONE', *, *, #64557, .F. ) ;
#72292=CYLINDRICAL_SURFACE ( 'NONE', #18626, 32.50000000000000711 ) ;
#72294=CARTESIAN_POINT ( 'NONE',  ( 68.91678303834669350, -69.56165394957326953, 247.5002289977139753 ) ) ;
#72315=ORIENTED_EDGE ( 'NONE', *, *, #28687, .T. ) ;
#72319=ORIENTED_EDGE ( 'NONE', *, *, #76280, .T. ) ;
#72328=ORIENTED_EDGE ( 'NONE', *, *, #7140, .T. ) ;
#72344=CARTESIAN_POINT ( 'NONE',  ( 68.94728689011853362, -139.0532934344234093, 246.8082357644148317 ) ) ;
#72388=B_SPLINE_CURVE_WITH_KNOTS ( 'NONE', 3,
 ( #29003, #56688, #14021, #55330, #35347, #20838 ),
 .UNSPECIFIED., .F., .F.,
 ( 4, 1, 1, 4 ),
 ( 0.000000000000000000, 0.5730588445129599640, 0.7191761746442985048, 1.000000000000000000 ),
 .UNSPECIFIED. ) ;
#72401=CARTESIAN_POINT ( 'NONE',  ( 94.91729554090750298, -74.61471936332451094, 249.3134381260879877 ) ) ;
#72407=DIRECTION ( 'NONE',  ( 1.000000000000000000, 1.000000000000000078E-15, 0.000000000000000000 ) ) ;
#72413=AXIS2_PLACEMENT_3D ( 'NONE', #48940, #55749, #33545 ) ;
#72448=DIRECTION ( 'NONE',  ( 0.000000000000000000, 0.000000000000000000, 1.000000000000000000 ) ) ;
#72470=CARTESIAN_POINT ( 'NONE',  ( 85.06670390244700286, -71.37844715994096134, 55.21780685541800437 ) ) ;
#72472=EDGE_CURVE ( 'NONE', #9965, #59337, #1929, .T. ) ;
#72474=ADVANCED_FACE ( 'NONE', ( #57772 ), #23291, .T. ) ;
#72483=EDGE_CURVE ( 'NONE', #81489, #15404, #18880, .T. ) ;
#72495=DIRECTION ( 'NONE',  ( -8.538276166416950255E-16, 1.000000000000000000, -3.100000000000000044E-14 ) ) ;
#72498=DIRECTION ( 'NONE',  ( 1.000000000000000000, 1.000000000000000078E-15, 0.000000000000000000 ) ) ;
#72522=ORIENTED_EDGE ( 'NONE', *, *, #83582, .F. ) ;
#72532=STYLED_ITEM ( 'NONE', ( #28766 ), #20639 ) ;
#72571=ORIENTED_EDGE ( 'NONE', *, *, #71384, .F. ) ;
#72589=CARTESIAN_POINT ( 'NONE',  ( 107.0667039024470313, -104.2784471599418197, -11.78219314458200984 ) ) ;
#72606=LINE ( 'NONE', #10370, #66095 ) ;
#72638=DIRECTION ( 'NONE',  ( -3.100000000000000258E-29, 3.100000000000000044E-14, 1.000000000000000000 ) ) ;
#72640=CARTESIAN_POINT ( 'NONE',  ( 103.8797721312301405, -101.8611209747507189, 2.217806855417919998 ) ) ;
#72642=ORIENTED_EDGE ( 'NONE', *, *, #33511, .F. ) ;
#72649=DIRECTION ( 'NONE',  ( 0.7967329428042202455, -0.6043315462976655006, 1.908195823574484964E-14 ) ) ;
#72664=DIRECTION ( 'NONE',  ( 3.100000000000000258E-29, -3.100000000000000044E-14, -1.000000000000000000 ) ) ;
#72668=ORIENTED_EDGE ( 'NONE', *, *, #14423, .T. ) ;
#72680=ORIENTED_EDGE ( 'NONE', *, *, #63026, .F. ) ;
#72684=LINE ( 'NONE', #65844, #36563 ) ;
#72685=VERTEX_POINT ( 'NONE', #34077 ) ;
#72709=ORIENTED_EDGE ( 'NONE', *, *, #83582, .T. ) ;
#72713=ORIENTED_EDGE ( 'NONE', *, *, #69862, .F. ) ;
#72722=CARTESIAN_POINT ( 'NONE',  ( 81.84766347661003749, -124.7784471599409670, 55.21780685541800437 ) ) ;
#72726=ORIENTED_EDGE ( 'NONE', *, *, #58519, .T. ) ;
#72734=AXIS2_PLACEMENT_3D ( 'NONE', #29111, #49527, #70445 ) ;
#72755=ORIENTED_EDGE ( 'NONE', *, *, #80928, .T. ) ;
#72767=EDGE_CURVE ( 'NONE', #56556, #1304, #53610, .T. ) ;
#72772=PLANE ( 'NONE',  #31598 ) ;
#72786=CARTESIAN_POINT ( 'NONE',  ( 70.56670390244700286, -68.87844715994098976, 55.21780685541800437 ) ) ;
#72788=EDGE_CURVE ( 'NONE', #34853, #35731, #86335, .T. ) ;
#72789=DIRECTION ( 'NONE',  ( -1.000000000000000078E-15, 1.000000000000000000, -3.100000000000000044E-14 ) ) ;
#72819=AXIS2_PLACEMENT_3D ( 'NONE', #33973, #47595, #81268 ) ;
#72836=CARTESIAN_POINT ( 'NONE',  ( 145.9076452860354891, -68.98966598118471438, 247.3116641508191549 ) ) ;
#72855=CARTESIAN_POINT ( 'NONE',  ( 70.06670390244707392, -137.6784471599409869, 55.21780685541800437 ) ) ;
#72879=DIRECTION ( 'NONE',  ( -1.000000000000000000, -1.000000000000000078E-15, 0.000000000000000000 ) ) ;
#72881=CARTESIAN_POINT ( 'NONE',  ( 143.8111385288040651, -140.2566682859662706, 246.7635256640583918 ) ) ;
#72883=CARTESIAN_POINT ( 'NONE',  ( 144.5667039024470171, -90.27844715994091018, 45.21780685541799727 ) ) ;
#72889=ADVANCED_FACE ( 'NONE', ( #64497, #43131, #921, #84955, #29081, #71320 ), #42678, .T. ) ;
#72896=DIRECTION ( 'NONE',  ( -1.000000000000000000, -1.734723475976808672E-15, 0.000000000000000000 ) ) ;
#72913=DIRECTION ( 'NONE',  ( 1.000000000000000078E-15, -1.000000000000000000, 0.000000000000000000 ) ) ;
#72975=CARTESIAN_POINT ( 'NONE',  ( 68.69171528984767860, -139.3034585473416769, 245.6607614303540004 ) ) ;
#72995=EDGE_CURVE ( 'NONE', #28990, #65875, #62451, .T. ) ;
#73007=DIRECTION ( 'NONE',  ( 8.538276166416950255E-16, -1.000000000000000000, 3.100000000000000044E-14 ) ) ;
#73026=VECTOR ( 'NONE', #53438, 1000.000000000000000 ) ;
#73036=ORIENTED_EDGE ( 'NONE', *, *, #52215, .F. ) ;
#73045=LINE ( 'NONE', #66682, #52265 ) ;
#73067=AXIS2_PLACEMENT_3D ( 'NONE', #29090, #71768, #77687 ) ;
#73075=CARTESIAN_POINT ( 'NONE',  ( 112.7812478461076040, -67.87844715994094713, 245.8358747327640117 ) ) ;
#73079=ORIENTED_EDGE ( 'NONE', *, *, #25606, .T. ) ;
#73108=ORIENTED_EDGE ( 'NONE', *, *, #31325, .F. ) ;
#73118=ORIENTED_EDGE ( 'NONE', *, *, #30789, .T. ) ;
#73181=ORIENTED_EDGE ( 'NONE', *, *, #60837, .F. ) ;
#73184=ORIENTED_EDGE ( 'NONE', *, *, #39381, .T. ) ;
#73191=PLANE ( 'NONE',  #12379 ) ;
#73195=ORIENTED_EDGE ( 'NONE', *, *, #30979, .T. ) ;
#73204=DIRECTION ( 'NONE',  ( 1.000000000000000000, 1.000000000000000078E-15, 0.000000000000000000 ) ) ;
#73211=VECTOR ( 'NONE', #53606, 1000.000000000000000 ) ;
#73219=CARTESIAN_POINT ( 'NONE',  ( 145.7544960090152983, -67.86889861335799878, 247.4138443563959981 ) ) ;
#73225=CARTESIAN_POINT ( 'NONE',  ( 110.0667047667142953, -70.87844715994094713, 173.2178068554179902 ) ) ;
#73239=FACE_OUTER_BOUND ( 'NONE', #88647, .T. ) ;
#73254=EDGE_CURVE ( 'NONE', #4351, #25758, #36226, .T. ) ;
#73262=EDGE_LOOP ( 'NONE', ( #79317, #3479, #71604, #76796 ) ) ;
#73265=CARTESIAN_POINT ( 'NONE',  ( 80.58723842074230959, -73.69558419411040973, 248.4067532124560103 ) ) ;
#73268=CARTESIAN_POINT ( 'NONE',  ( 59.56670390244700997, -79.67844715994098692, 190.2178068554179902 ) ) ;
#73278=EDGE_LOOP ( 'NONE', ( #29869, #33809, #15330, #33077, #73350, #59429 ) ) ;
#73289=ORIENTED_EDGE ( 'NONE', *, *, #20358, .T. ) ;
#73293=ORIENTED_EDGE ( 'NONE', *, *, #85717, .T. ) ;
#73296=ORIENTED_EDGE ( 'NONE', *, *, #51566, .T. ) ;
#73322=CARTESIAN_POINT ( 'NONE',  ( 143.5504647578642050, -139.6982893664599885, 247.2544030524684615 ) ) ;
#73323=CARTESIAN_POINT ( 'NONE',  ( 154.5667039024469886, -67.87844715994090450, 85.21780685541799016 ) ) ;
#73350=ORIENTED_EDGE ( 'NONE', *, *, #74356, .F. ) ;
#73357=CARTESIAN_POINT ( 'NONE',  ( 122.2221484686745470, -111.9799080603168022, -11.78219314458175937 ) ) ;
#73365=ORIENTED_EDGE ( 'NONE', *, *, #58117, .F. ) ;
#73382=LINE ( 'NONE', #4354, #86526 ) ;
#73401=AXIS2_PLACEMENT_3D ( 'NONE', #60632, #53351, #11614 ) ;
#73402=ORIENTED_EDGE ( 'NONE', *, *, #54319, .T. ) ;
#73421=LINE ( 'NONE', #2164, #37267 ) ;
#73434=CARTESIAN_POINT ( 'NONE',  ( 107.0667039024470313, -104.2784471599414502, 0.2178068554180012661 ) ) ;
#73439=DIRECTION ( 'NONE',  ( 1.000000000000000000, 0.000000000000000000, 0.000000000000000000 ) ) ;
#73451=CYLINDRICAL_SURFACE ( 'NONE', #45217, 3.000000000000002665 ) ;
#73460=CARTESIAN_POINT ( 'NONE',  ( 129.9696172393100539, -140.6784471630960240, 245.6313762643000018 ) ) ;
#73463=DIRECTION ( 'NONE',  ( -2.195856868753399715E-16, -1.000000000000000000, 0.000000000000000000 ) ) ;
#73464=CARTESIAN_POINT ( 'NONE',  ( 69.55244702860527184, -138.4431012436765798, 247.5929369389089914 ) ) ;
#73465=AXIS2_PLACEMENT_3D ( 'NONE', #86500, #85172, #65148 ) ;
#73474=AXIS2_PLACEMENT_3D ( 'NONE', #70951, #35962, #36425 ) ;
#73494=ORIENTED_EDGE ( 'NONE', *, *, #7351, .F. ) ;
#73506=DIRECTION ( 'NONE',  ( -0.8660254037844381525, -0.5000000000000007772, 1.549999999999999706E-14 ) ) ;
#73508=CARTESIAN_POINT ( 'NONE',  ( 74.68590548172718968, -67.87844715994097555, 245.5622121550900090 ) ) ;
#73518=VERTEX_POINT ( 'NONE', #52929 ) ;
#73521=DIRECTION ( 'NONE',  ( -1.000000000000000000, -1.000000000000000078E-15, 0.000000000000000000 ) ) ;
#73547=ORIENTED_EDGE ( 'NONE', *, *, #46780, .T. ) ;
#73581=ORIENTED_EDGE ( 'NONE', *, *, #14142, .F. ) ;
#73590=EDGE_CURVE ( 'NONE', #83707, #34621, #21176, .T. ) ;
#73598=VECTOR ( 'NONE', #72789, 1000.000000000000000 ) ;
#73606=PLANE ( 'NONE',  #19789 ) ;
#73628=EDGE_LOOP ( 'NONE', ( #76941, #76409, #80492, #42166 ) ) ;
#73663=VECTOR ( 'NONE', #70127, 1000.000000000000000 ) ;
#73672=PLANE ( 'NONE',  #23501 ) ;
#73678=FACE_OUTER_BOUND ( 'NONE', #88521, .T. ) ;
#73688=DIRECTION ( 'NONE',  ( -3.100000000000000258E-29, 3.100000000000000044E-14, 1.000000000000000000 ) ) ;
#73691=ORIENTED_EDGE ( 'NONE', *, *, #43620, .F. ) ;
#73702=LINE ( 'NONE', #2885, #3710 ) ;
#73706=DIRECTION ( 'NONE',  ( 0.9217329428042198014, 0.3878251953515564066, -1.214306433183767175E-14 ) ) ;
#73709=ORIENTED_EDGE ( 'NONE', *, *, #1907, .F. ) ;
#73714=DIRECTION ( 'NONE',  ( 1.000000000000000000, 0.000000000000000000, 0.000000000000000000 ) ) ;
#73716=DIRECTION ( 'NONE',  ( 3.100000000000000258E-29, -3.100000000000000044E-14, -1.000000000000000000 ) ) ;
#73720=LINE ( 'NONE', #74170, #56011 ) ;
#73724=CARTESIAN_POINT ( 'NONE',  ( 133.3679539845121269, -80.39464238368842075, 249.3134381260879877 ) ) ;
#73725=CARTESIAN_POINT ( 'NONE',  ( 147.0242276106250756, -67.91655684465823128, 245.8961201463810085 ) ) ;
#73762=CARTESIAN_POINT ( 'NONE',  ( 92.81551872686563343, -113.5468731908971307, -11.78219314458173272 ) ) ;
#73782=ADVANCED_FACE ( 'NONE', ( #70193 ), #7966, .F. ) ;
#73784=CARTESIAN_POINT ( 'NONE',  ( 144.0667039024470739, -137.6784471599409017, 55.21780685541800437 ) ) ;
#73785=CARTESIAN_POINT ( 'NONE',  ( 69.15045923641616810, -139.7622024939100811, 245.5930228695460187 ) ) ;
#73797=DIRECTION ( 'NONE',  ( -3.100000000000000258E-29, 3.100000000000000044E-14, 1.000000000000000000 ) ) ;
#73803=ORIENTED_EDGE ( 'NONE', *, *, #58531, .T. ) ;
#73828=CARTESIAN_POINT ( 'NONE',  ( 67.06796439462205228, -67.87878520888916967, 245.5492565716537001 ) ) ;
#73843=ORIENTED_EDGE ( 'NONE', *, *, #31602, .F. ) ;
#73845=LINE ( 'NONE', #26591, #73927 ) ;
#73849=DIRECTION ( 'NONE',  ( -3.100000000000000258E-29, 3.100000000000000044E-14, 1.000000000000000000 ) ) ;
#73876=CARTESIAN_POINT ( 'NONE',  ( 52.06670390244699576, -67.87844715994100397, 55.21780685541800437 ) ) ;
#73887=EDGE_CURVE ( 'NONE', #63654, #25238, #3126, .T. ) ;
#73890=AXIS2_PLACEMENT_3D ( 'NONE', #67168, #74441, #86737 ) ;
#73894=ADVANCED_FACE ( 'NONE', ( #44256 ), #6041, .F. ) ;
#73898=ORIENTED_EDGE ( 'NONE', *, *, #119, .F. ) ;
#73915=DIRECTION ( 'NONE',  ( 0.000000000000000000, 0.000000000000000000, 1.000000000000000000 ) ) ;
#73919=FACE_OUTER_BOUND ( 'NONE', #13846, .T. ) ;
#73927=VECTOR ( 'NONE', #18430, 1000.000000000000000 ) ;
#73928=VERTEX_POINT ( 'NONE', #62711 ) ;
#73961=CARTESIAN_POINT ( 'NONE',  ( 131.8286707874590036, -67.87844715994091871, 245.6137563247699802 ) ) ;
#73966=CARTESIAN_POINT ( 'NONE',  ( 85.06670390244700286, -71.37844715994096134, 55.21780685541800437 ) ) ;
#73967=ORIENTED_EDGE ( 'NONE', *, *, #22866, .T. ) ;
#73968=EDGE_CURVE ( 'NONE', #4351, #31932, #41354, .T. ) ;
#73980=CARTESIAN_POINT ( 'NONE',  ( 50.11670390244700712, -75.72844715994099829, 55.21780685541800437 ) ) ;
#74018=CARTESIAN_POINT ( 'NONE',  ( 154.5667039024469886, -67.87844715994090450, 85.21780685541799016 ) ) ;
#74029=LINE ( 'NONE', #12708, #79078 ) ;
#74043=CARTESIAN_POINT ( 'NONE',  ( 154.5667039024469886, -67.87844715994090450, 85.21780685541799016 ) ) ;
#74078=VECTOR ( 'NONE', #69672, 1000.000000000000000 ) ;
#74079=LINE ( 'NONE', #48141, #20195 ) ;
#74101=CARTESIAN_POINT ( 'NONE',  ( 162.0667039024469886, -67.87844715994089029, 55.21780685541800437 ) ) ;
#74104=CARTESIAN_POINT ( 'NONE',  ( 74.76629182358846037, -133.7001020459428844, 248.3919653347779786 ) ) ;
#74111=DIRECTION ( 'NONE',  ( 0.000000000000000000, 0.000000000000000000, -1.000000000000000000 ) ) ;
#74112=ORIENTED_EDGE ( 'NONE', *, *, #27466, .F. ) ;
#74134=FACE_BOUND ( 'NONE', #17535, .T. ) ;
#74148=VECTOR ( 'NONE', #63192, 1000.000000000000000 ) ;
#74166=FACE_OUTER_BOUND ( 'NONE', #84280, .T. ) ;
#74170=CARTESIAN_POINT ( 'NONE',  ( 110.7536356736639078, -102.7271463785358492, -19.78219314458207378 ) ) ;
#74171=B_SPLINE_SURFACE_WITH_KNOTS ( 'NONE', 3, 3, ( 
 ( #87364, #24243, #45108, #3356 ),
 ( #31046, #73265, #24683, #65126 ),
 ( #2909, #57862, #72401, #37874 ),
 ( #86038, #9720, #39198, #17864 ),
 ( #3794, #65574, #38306, #30161 ),
 ( #31481, #80552, #85596, #25124 ),
 ( #2466, #52350, #73724, #51913 ) ),
 .UNSPECIFIED., .F., .F., .F.,
 ( 4, 1, 1, 1, 4 ),
 ( 4, 4 ),
 ( -0.0007720614341078669424, 0.2857142857142860315, 0.5714285714285709528, 0.8571428571428569843, 1.000772061434110016 ),
 ( 0.09408714780213320306, 1.000772061434110016 ),
 .UNSPECIFIED. ) ;
#74188=CARTESIAN_POINT ( 'NONE',  ( 98.06670458790040357, -71.37844715994094713, 55.21780685541800437 ) ) ;
#74190=VERTEX_POINT ( 'NONE', #79943 ) ;
#74200=LINE ( 'NONE', #32849, #76797 ) ;
#74220=DIRECTION ( 'NONE',  ( -3.100000000000000258E-29, 3.100000000000000044E-14, 1.000000000000000000 ) ) ;
#74226=CARTESIAN_POINT ( 'NONE',  ( 69.94616667561825807, -138.0587426493221699, 247.6570821721479945 ) ) ;
#74228=EDGE_LOOP ( 'NONE', ( #68182, #75407, #68507, #37052, #6149, #62924 ) ) ;
#74250=EDGE_CURVE ( 'NONE', #77633, #54044, #30739, .T. ) ;
#74256=FACE_OUTER_BOUND ( 'NONE', #41527, .T. ) ;
#74274=VERTEX_POINT ( 'NONE', #32655 ) ;
#74300=EDGE_CURVE ( 'NONE', #61315, #72685, #48060, .T. ) ;
#74338=PLANE ( 'NONE',  #35413 ) ;
#74343=FACE_OUTER_BOUND ( 'NONE', #53884, .T. ) ;
#74356=EDGE_CURVE ( 'NONE', #49237, #1627, #6057, .T. ) ;
#74372=CARTESIAN_POINT ( 'NONE',  ( 144.9304472658408258, -138.7995020472562828, 247.3025957270601225 ) ) ;
#74380=ADVANCED_FACE ( 'NONE', ( #13561 ), #19032, .F. ) ;
#74391=ORIENTED_EDGE ( 'NONE', *, *, #29560, .F. ) ;
#74413=LINE ( 'NONE', #83038, #65775 ) ;
#74441=DIRECTION ( 'NONE',  ( 1.000000000000000078E-15, -1.000000000000000000, 0.000000000000000000 ) ) ;
#74490=CARTESIAN_POINT ( 'NONE',  ( 107.0667039024470313, -104.2784471599420755, -19.78219314458201694 ) ) ;
#74492=VERTEX_POINT ( 'NONE', #89885 ) ;
#74501=CARTESIAN_POINT ( 'NONE',  ( 107.0667039024470171, -89.08784823670062281, -21.78219314458248945 ) ) ;
#74506=ORIENTED_EDGE ( 'NONE', *, *, #4765, .F. ) ;
#74523=VECTOR ( 'NONE', #76612, 1000.000000000000000 ) ;
#74539=ORIENTED_EDGE ( 'NONE', *, *, #89462, .T. ) ;
#74544=DIRECTION ( 'NONE',  ( 1.000000000000000000, 0.000000000000000000, 0.000000000000000000 ) ) ;
#74549=CARTESIAN_POINT ( 'NONE',  ( 78.94219608136785382, -124.1415542323586720, 249.3055308415380011 ) ) ;
#74556=CARTESIAN_POINT ( 'NONE',  ( 86.61913848402866734, -135.9065445298735710, 248.4142799812389910 ) ) ;
#74558=VECTOR ( 'NONE', #22411, 1000.000000000000000 ) ;
#74596=DIRECTION ( 'NONE',  ( -3.555032108465730541E-16, 1.000000000000000000, 0.000000000000000000 ) ) ;
#74615=EDGE_CURVE ( 'NONE', #47600, #34651, #62643, .T. ) ;
#74625=( BOUNDED_CURVE ( )  B_SPLINE_CURVE ( 2, ( #13194, #82697, #63120 ),
 .UNSPECIFIED., .F., .T. ) 
 B_SPLINE_CURVE_WITH_KNOTS ( ( 3, 3 ),
 ( 0.000000000000000000, 0.5053286420056740669 ),
 .UNSPECIFIED. ) 
 CURVE ( )  GEOMETRIC_REPRESENTATION_ITEM ( )  RATIONAL_B_SPLINE_CURVE ( ( 1.000000000000000000, 1.009299002520649857, 1.000420656333769864 ) ) 
 REPRESENTATION_ITEM ( '' )  );
#74651=CARTESIAN_POINT ( 'NONE',  ( 146.0667039024470171, -86.77844715994089597, 55.21780685541800437 ) ) ;
#74675=CARTESIAN_POINT ( 'NONE',  ( 122.2221484686747317, -96.68314769832136335, -21.78219314458224076 ) ) ;
#74676=CARTESIAN_POINT ( 'NONE',  ( 115.0439452383992318, -109.4614598618342853, -19.78219314458184996 ) ) ;
#74700=EDGE_CURVE ( 'NONE', #24432, #21921, #17647, .T. ) ;
#74716=CIRCLE ( 'NONE', #34112, 8.999999999999994671 ) ;
#74718=VECTOR ( 'NONE', #17953, 1000.000000000000227 ) ;
#74724=CARTESIAN_POINT ( 'NONE',  ( 70.06670417066790435, -71.37844715994097555, 55.21780685541800437 ) ) ;
#74728=CARTESIAN_POINT ( 'NONE',  ( 59.67056972692184758, -130.5939552371641810, 126.9238073910411941 ) ) ;
#74732=ORIENTED_EDGE ( 'NONE', *, *, #13978, .F. ) ;
#74740=VERTEX_POINT ( 'NONE', #52075 ) ;
#74785=CARTESIAN_POINT ( 'NONE',  ( 154.5667039024470171, -79.67844715994088745, 85.21780685541799016 ) ) ;
#74796=CARTESIAN_POINT ( 'NONE',  ( 59.56670390244699576, -67.87844715994098976, 190.2178068554179902 ) ) ;
#74818=CARTESIAN_POINT ( 'NONE',  ( 145.3840438162638407, -139.2490617783571167, 246.2187065265057413 ) ) ;
#74821=CARTESIAN_POINT ( 'NONE',  ( 70.10184668782046913, -140.7135899453143963, 245.8512780488630085 ) ) ;
#74829=VECTOR ( 'NONE', #47367, 999.9999999999998863 ) ;
#74839=ADVANCED_FACE ( 'NONE', ( #60691 ), #5304, .F. ) ;
#74840=ORIENTED_EDGE ( 'NONE', *, *, #65811, .F. ) ;
#74889=CARTESIAN_POINT ( 'NONE',  ( 162.0667039024469886, -68.87844715994089029, 96.96780685541800437 ) ) ;
#74893=PLANE ( 'NONE',  #55021 ) ;
#74895=CARTESIAN_POINT ( 'NONE',  ( 110.2536356736639220, -106.6957733451327215, -19.78219314458193168 ) ) ;
#74904=FACE_OUTER_BOUND ( 'NONE', #70181, .T. ) ;
#74910=DIRECTION ( 'NONE',  ( -3.100000000000000258E-29, 3.100000000000000044E-14, 1.000000000000000000 ) ) ;
#74919=FACE_OUTER_BOUND ( 'NONE', #36179, .T. ) ;
#74920=ORIENTED_EDGE ( 'NONE', *, *, #7369, .T. ) ;
#74943=ORIENTED_EDGE ( 'NONE', *, *, #55940, .F. ) ;
#74954=CARTESIAN_POINT ( 'NONE',  ( 147.0667039024469886, -67.87844715994090450, 222.2178068554179902 ) ) ;
#74957=ORIENTED_EDGE ( 'NONE', *, *, #89170, .F. ) ;
#74961=CARTESIAN_POINT ( 'NONE',  ( 107.0667039024470313, -104.2784471599409528, 222.2178068554179902 ) ) ;
#74962=LINE ( 'NONE', #25923, #15760 ) ;
#74973=ADVANCED_FACE ( 'NONE', ( #74343 ), #27087, .F. ) ;
#74974=VERTEX_POINT ( 'NONE', #89776 ) ;
#75010=AXIS2_PLACEMENT_3D ( 'NONE', #60818, #74910, #12693 ) ;
#75012=VERTEX_POINT ( 'NONE', #41144 ) ;
#75023=CARTESIAN_POINT ( 'NONE',  ( 147.0667039024470739, -137.6786872052068134, 246.0480660933869785 ) ) ;
#75028=EDGE_CURVE ( 'NONE', #55721, #63478, #25736, .T. ) ;
#75037=CARTESIAN_POINT ( 'NONE',  ( 145.5844531081931166, -75.99209099266981582, 247.4783998280190076 ) ) ;
#75093=CONICAL_SURFACE ( 'NONE', #47528, 16.25000000000000000, 0.5235987755982992597 ) ;
#75115=ORIENTED_EDGE ( 'NONE', *, *, #86746, .T. ) ;
#75154=ADVANCED_FACE ( 'NONE', ( #85211 ), #48844, .F. ) ;
#75168=( BOUNDED_CURVE ( )  B_SPLINE_CURVE ( 2, ( #7895, #48762, #21083 ),
 .UNSPECIFIED., .F., .T. ) 
 B_SPLINE_CURVE_WITH_KNOTS ( ( 3, 3 ),
 ( 0.000000000000000000, 0.5053286420056790629 ),
 .UNSPECIFIED. ) 
 CURVE ( )  GEOMETRIC_REPRESENTATION_ITEM ( )  RATIONAL_B_SPLINE_CURVE ( ( 1.000000000000000000, 1.009299002520649857, 1.000420656333769864 ) ) 
 REPRESENTATION_ITEM ( '' )  );
#75171=FACE_BOUND ( 'NONE', #21456, .T. ) ;
#75172=DIRECTION ( 'NONE',  ( 0.000000000000000000, 0.000000000000000000, 1.000000000000000000 ) ) ;
#75217=FACE_OUTER_BOUND ( 'NONE', #5527, .T. ) ;
#75241=LINE ( 'NONE', #47947, #42278 ) ;
#75242=CARTESIAN_POINT ( 'NONE',  ( 140.0667039024470455, -118.2784471599408960, 45.21780685541799727 ) ) ;
#75262=VERTEX_POINT ( 'NONE', #37481 ) ;
#75268=CARTESIAN_POINT ( 'NONE',  ( 130.5667039024470455, -104.2784471599409386, 24.21780685541800082 ) ) ;
#75270=CARTESIAN_POINT ( 'NONE',  ( 112.3535505598876654, -140.6782308490354296, 246.2059492953349888 ) ) ;
#75273=CARTESIAN_POINT ( 'NONE',  ( 145.4199999577330402, -139.2838544871431168, 246.0004081004534555 ) ) ;
#75291=B_SPLINE_CURVE_WITH_KNOTS ( 'NONE', 3,
 ( #56590, #22540, #50671, #43852, #42061, #14834 ),
 .UNSPECIFIED., .F., .F.,
 ( 4, 2, 4 ),
 ( -0.009166911786111989549, -0.004585838005518491980, 0.000000000000000000 ),
 .UNSPECIFIED. ) ;
#75300=CIRCLE ( 'NONE', #85506, 1.999999999999995781 ) ;
#75315=VERTEX_POINT ( 'NONE', #38807 ) ;
#75320=FACE_BOUND ( 'NONE', #625, .T. ) ;
#75352=VERTEX_POINT ( 'NONE', #66059 ) ;
#75366=SHAPE_DEFINITION_REPRESENTATION ( #40083, #14421 ) ;
#75370=ORIENTED_EDGE ( 'NONE', *, *, #83229, .F. ) ;
#75371=CARTESIAN_POINT ( 'NONE',  ( 106.1656040943334602, -121.2545485715093463, -19.18411693322849487 ) ) ;
#75377=FACE_OUTER_BOUND ( 'NONE', #12462, .T. ) ;
#75387=VECTOR ( 'NONE', #46152, 1000.000000000000000 ) ;
#75402=ADVANCED_FACE ( 'NONE', ( #46945 ), #54645, .F. ) ;
#75407=ORIENTED_EDGE ( 'NONE', *, *, #51162, .T. ) ;
#75430=EDGE_CURVE ( 'NONE', #15550, #82481, #68763, .T. ) ;
#75452=ORIENTED_EDGE ( 'NONE', *, *, #36168, .T. ) ;
#75464=EDGE_LOOP ( 'NONE', ( #73184, #45581, #33761, #19769, #61265 ) ) ;
#75468=CARTESIAN_POINT ( 'NONE',  ( 124.4804366973139622, -125.9844606681579364, 250.2203867545810283 ) ) ;
#75495=DIRECTION ( 'NONE',  ( -0.7071067811865453523, -0.7071067811865496822, 0.000000000000000000 ) ) ;
#75502=CARTESIAN_POINT ( 'NONE',  ( 68.80307738653738170, -139.4148206440312947, 246.0960064844549890 ) ) ;
#75510=CARTESIAN_POINT ( 'NONE',  ( 160.0667039024470171, -79.67844715994088745, 96.96780685541800437 ) ) ;
#75537=DIRECTION ( 'NONE',  ( 0.000000000000000000, 0.000000000000000000, -1.000000000000000000 ) ) ;
#75552=ORIENTED_EDGE ( 'NONE', *, *, #31463, .F. ) ;
#75555=VERTEX_POINT ( 'NONE', #61931 ) ;
#75557=EDGE_CURVE ( 'NONE', #19483, #21921, #80613, .T. ) ;
#75564=DIRECTION ( 'NONE',  ( 0.000000000000000000, 0.000000000000000000, -1.000000000000000000 ) ) ;
#75568=EDGE_LOOP ( 'NONE', ( #18740, #553 ) ) ;
#75569=ORIENTED_EDGE ( 'NONE', *, *, #79631, .T. ) ;
#75622=EDGE_CURVE ( 'NONE', #52976, #1304, #26527, .T. ) ;
#75625=CARTESIAN_POINT ( 'NONE',  ( 70.06695561434436570, -140.6784471599409869, 245.4721420304120159 ) ) ;
#75656=DIRECTION ( 'NONE',  ( 0.8660254037844392627, -0.4999999999999990008, 1.549999999999999706E-14 ) ) ;
#75663=ADVANCED_FACE ( 'NONE', ( #84646 ), #62380, .T. ) ;
#75671=CARTESIAN_POINT ( 'NONE',  ( 106.1656040943334318, -87.30234574837474781, -19.18411693322955003 ) ) ;
#75678=VERTEX_POINT ( 'NONE', #69656 ) ;
#75679=AXIS2_PLACEMENT_3D ( 'NONE', #53088, #12245, #85551 ) ;
#75680=DIRECTION ( 'NONE',  ( 1.000000000000000000, 8.953411488912556626E-16, 0.000000000000000000 ) ) ;
#75718=CARTESIAN_POINT ( 'NONE',  ( 110.7536356736639220, -105.8297479413476054, 2.217806855418058554 ) ) ;
#75729=CARTESIAN_POINT ( 'NONE',  ( 104.0667030381800942, -67.87844715994094713, 155.9678077345870122 ) ) ;
#75742=VECTOR ( 'NONE', #46742, 999.9999999999998863 ) ;
#75744=CIRCLE ( 'NONE', #72819, 1.999999999999995781 ) ;
#75746=DIRECTION ( 'NONE',  ( 1.000000000000000000, 1.000000000000000078E-15, 0.000000000000000000 ) ) ;
#75751=VERTEX_POINT ( 'NONE', #72786 ) ;
#75793=CARTESIAN_POINT ( 'NONE',  ( 122.2189888861419433, -111.9861225405538221, -11.78219314458175937 ) ) ;
#75795=DIRECTION ( 'NONE',  ( 1.000000000000000078E-15, -1.000000000000000000, 0.000000000000000000 ) ) ;
#75800=ORIENTED_EDGE ( 'NONE', *, *, #12782, .T. ) ;
#75805=CARTESIAN_POINT ( 'NONE',  ( 122.2221484686747459, -108.0760968907524955, -21.78219314458190681 ) ) ;
#75807=CARTESIAN_POINT ( 'NONE',  ( 144.0667052733537901, -83.77844715994091018, 222.2178068554179902 ) ) ;
#75812=VERTEX_POINT ( 'NONE', #2858 ) ;
#75821=ORIENTED_EDGE ( 'NONE', *, *, #88767, .T. ) ;
#75834=ORIENTED_EDGE ( 'NONE', *, *, #53019, .F. ) ;
#75839=LINE ( 'NONE', #24673, #61134 ) ;
#75851=VERTEX_POINT ( 'NONE', #9226 ) ;
#75864=B_SPLINE_CURVE_WITH_KNOTS ( 'NONE', 3,
 ( #80660, #53801, #81567, #73828, #39306, #67011, #87911, #81121, #15189, #28354, #55141, #50134, #22457, #42869, #56046, #76969, #83791, #77413, #20663, #77870, #29269, #62875, #651, #14753, #61977, #41087, #70604, #8378, #28823, #89715, #7920, #82903, #1567, #211, #48329, #35164, #21111, #68809, #21565, #35620, #13843, #62432, #27912, #41525, #42422 ),
 .UNSPECIFIED., .F., .F.,
 ( 4, 1, 1, 2, 2, 2, 1, 2, 2, 2, 2, 2, 1, 2, 2, 2, 2, 1, 1, 2, 2, 2, 1, 2, 2, 4 ),
 ( 0.000000000000000000, 0.007812499999944476706, 0.01171874999991686685, 0.01367187499991590408, 0.01562499999991493957, 0.02343749999997512753, 0.02734375000000554071, 0.02929687500002081321, 0.03125000000003608919, 0.06249999999996937172, 0.09374999999990264732, 0.1249999999998359368, 0.1874999999997302436, 0.2187499999996694866, 0.2499999999996087019, 0.3749999999993610111, 0.4374999999992401634, 0.4687499999991869282, 0.4843749999991663890, 0.4921874999991687205, 0.4999999999991709965, 0.6249999999993580690, 0.6874999999994604316, 0.7187499999995111688, 0.7499999999995617950, 1.000000000000000000 ),
 .UNSPECIFIED. ) ;
#75874=ORIENTED_EDGE ( 'NONE', *, *, #13603, .T. ) ;
#75908=CARTESIAN_POINT ( 'NONE',  ( 102.9783262188089594, -135.0490206179280506, 249.3173333679100097 ) ) ;
#75914=( NAMED_UNIT ( * ) PLANE_ANGLE_UNIT ( ) SI_UNIT ( $, .RADIAN. ) );
#75917=CARTESIAN_POINT ( 'NONE',  ( 68.49979375445622054, -104.6923134067608743, 247.6412730378945639 ) ) ;
#75921=CARTESIAN_POINT ( 'NONE',  ( 69.56670390244705970, -123.2784471599409812, 55.21780685541800437 ) ) ;
#75932=CARTESIAN_POINT ( 'NONE',  ( 135.2338238997143378, -107.2609675061132180, 250.2191008560389776 ) ) ;
#75943=CARTESIAN_POINT ( 'NONE',  ( 95.56670390244703128, -104.2784471599408818, 19.21780685541799016 ) ) ;
#75945=ADVANCED_FACE ( 'NONE', ( #31885 ), #73672, .F. ) ;
#75949=ORIENTED_EDGE ( 'NONE', *, *, #77825, .F. ) ;
#75955=CIRCLE ( 'NONE', #7805, 4.500000000000003553 ) ;
#75976=EDGE_LOOP ( 'NONE', ( #43187, #19904 ) ) ;
#75987=ORIENTED_EDGE ( 'NONE', *, *, #38964, .F. ) ;
#76019=CIRCLE ( 'NONE', #38336, 8.999999999999994671 ) ;
#76020=CARTESIAN_POINT ( 'NONE',  ( 63.06670390244700997, -79.67844715994098692, 190.2178068554179902 ) ) ;
#76034=ORIENTED_EDGE ( 'NONE', *, *, #31086, .T. ) ;
#76045=DIRECTION ( 'NONE',  ( -1.000000000000000000, -1.000000000000000078E-15, 0.000000000000000000 ) ) ;
#76050=ORIENTED_EDGE ( 'NONE', *, *, #44856, .F. ) ;
#76075=LINE ( 'NONE', #42881, #21857 ) ;
#76079=ORIENTED_EDGE ( 'NONE', *, *, #24991, .F. ) ;
#76083=CIRCLE ( 'NONE', #66091, 3.500000000000003109 ) ;
#76084=CARTESIAN_POINT ( 'NONE',  ( 144.1872411114284773, -138.0587426716868151, 247.6570821702239869 ) ) ;
#76096=VERTEX_POINT ( 'NONE', #85833 ) ;
#76112=AXIS2_PLACEMENT_3D ( 'NONE', #46519, #32448, #66982 ) ;
#76143=CIRCLE ( 'NONE', #661, 32.50000000000001421 ) ;
#76157=CARTESIAN_POINT ( 'NONE',  ( 145.3822798034300945, -139.2473393705360536, 246.2271668860497300 ) ) ;
#76165=VERTEX_POINT ( 'NONE', #28382 ) ;
#76171=LINE ( 'NONE', #75729, #69775 ) ;
#76175=ADVANCED_FACE ( 'NONE', ( #82147 ), #68046, .F. ) ;
#76204=ORIENTED_EDGE ( 'NONE', *, *, #24160, .T. ) ;
#76217=DIRECTION ( 'NONE',  ( 3.100000000000000258E-29, -3.100000000000000044E-14, -1.000000000000000000 ) ) ;
#76238=CARTESIAN_POINT ( 'NONE',  ( 107.5667039024470455, -113.7784471599413791, 2.217806855418308132 ) ) ;
#76243=FACE_BOUND ( 'NONE', #38365, .T. ) ;
#76245=ORIENTED_EDGE ( 'NONE', *, *, #45683, .F. ) ;
#76256=ORIENTED_EDGE ( 'NONE', *, *, #52240, .T. ) ;
#76260=CARTESIAN_POINT ( 'NONE',  ( 107.0667039024470313, -104.2784471599409528, 222.2178068554179902 ) ) ;
#76266=VERTEX_POINT ( 'NONE', #12639 ) ;
#76269=CIRCLE ( 'NONE', #50187, 8.999999999999994671 ) ;
#76280=EDGE_CURVE ( 'NONE', #67362, #4351, #82954, .T. ) ;
#76304=DIRECTION ( 'NONE',  ( -1.000000000000000000, -8.953411488912552682E-16, 0.000000000000000000 ) ) ;
#76318=DIRECTION ( 'NONE',  ( 1.000000000000000000, 1.000000000000000078E-15, 0.000000000000000000 ) ) ;
#76330=ORIENTED_EDGE ( 'NONE', *, *, #41989, .T. ) ;
#76357=EDGE_CURVE ( 'NONE', #16796, #11319, #75744, .T. ) ;
#76362=VECTOR ( 'NONE', #78420, 1000.000000000000000 ) ;
#76378=CARTESIAN_POINT ( 'NONE',  ( 133.3763278023386647, -128.2462349309375043, 249.3055338466990065 ) ) ;
#76386=LINE ( 'NONE', #15964, #89377 ) ;
#76394=ORIENTED_EDGE ( 'NONE', *, *, #85582, .T. ) ;
#76399=VECTOR ( 'NONE', #16536, 1000.000000000000000 ) ;
#76404=CARTESIAN_POINT ( 'NONE',  ( 121.3178890780284434, -113.5468731908973439, -19.18411693322874356 ) ) ;
#76409=ORIENTED_EDGE ( 'NONE', *, *, #89164, .T. ) ;
#76421=EDGE_LOOP ( 'NONE', ( #75834, #2929, #18644, #85054, #33752, #21158 ) ) ;
#76427=DIRECTION ( 'NONE',  ( 1.000000000000000000, 1.000000000000000078E-15, 0.000000000000000000 ) ) ;
#76441=EDGE_CURVE ( 'NONE', #6854, #82398, #18116, .T. ) ;
#76455=CIRCLE ( 'NONE', #43115, 7.999999999999992895 ) ;
#76461=VECTOR ( 'NONE', #5707, 1000.000000000000000 ) ;
#76466=DIRECTION ( 'NONE',  ( -1.000000000000000078E-15, 1.000000000000000000, 0.000000000000000000 ) ) ;
#76472=CARTESIAN_POINT ( 'NONE',  ( 92.81551872686561921, -95.01002112898675023, -19.18411693322930134 ) ) ;
#76473=EDGE_CURVE ( 'NONE', #38611, #22233, #42130, .T. ) ;
#76497=CARTESIAN_POINT ( 'NONE',  ( 70.06174462629407174, -138.9592723264546521, 247.5160078862170110 ) ) ;
#76508=DIRECTION ( 'NONE',  ( -3.100000000000000258E-29, 3.100000000000000044E-14, 1.000000000000000000 ) ) ;
#76522=CARTESIAN_POINT ( 'NONE',  ( 145.5835616515379627, -69.28104898940431156, 247.4312010763500211 ) ) ;
#76527=CIRCLE ( 'NONE', #72188, 4.500000000000003553 ) ;
#76531=ORIENTED_EDGE ( 'NONE', *, *, #8377, .F. ) ;
#76537=ORIENTED_EDGE ( 'NONE', *, *, #72472, .T. ) ;
#76551=ORIENTED_EDGE ( 'NONE', *, *, #22638, .T. ) ;
#76564=VERTEX_POINT ( 'NONE', #43019 ) ;
#76570=VECTOR ( 'NONE', #24371, 1000.000000000000000 ) ;
#76605=AXIS2_PLACEMENT_3D ( 'NONE', #24877, #80304, #18053 ) ;
#76609=AXIS2_PLACEMENT_3D ( 'NONE', #74961, #68152, #39540 ) ;
#76612=DIRECTION ( 'NONE',  ( -1.000000000000000078E-15, 1.000000000000000000, 0.000000000000000000 ) ) ;
#76613=AXIS2_PLACEMENT_3D ( 'NONE', #25847, #72664, #59453 ) ;
#76635=AXIS2_PLACEMENT_3D ( 'NONE', #37876, #65576, #3358 ) ;
#76644=ORIENTED_EDGE ( 'NONE', *, *, #28247, .F. ) ;
#76649=VECTOR ( 'NONE', #79721, 1000.000000000000000 ) ;
#76656=DIRECTION ( 'NONE',  ( -1.000000000000000000, 0.000000000000000000, 0.000000000000000000 ) ) ;
#76671=EDGE_LOOP ( 'NONE', ( #31823, #22709 ) ) ;
#76672=AXIS2_PLACEMENT_3D ( 'NONE', #61519, #61969, #60172 ) ;
#76678=CARTESIAN_POINT ( 'NONE',  ( 162.0667039024469886, -67.87844715994089029, 222.2178068554179902 ) ) ;
#76681=DIRECTION ( 'NONE',  ( 0.000000000000000000, 0.000000000000000000, -1.000000000000000000 ) ) ;
#76696=DIRECTION ( 'NONE',  ( 1.000000000000000000, 0.000000000000000000, 0.000000000000000000 ) ) ;
#76713=DIRECTION ( 'NONE',  ( 1.000000000000000000, 0.000000000000000000, 0.000000000000000000 ) ) ;
#76714=AXIS2_PLACEMENT_3D ( 'NONE', #78279, #51860, #59129 ) ;
#76724=DIRECTION ( 'NONE',  ( -3.100000000000000258E-29, 3.100000000000000044E-14, 1.000000000000000000 ) ) ;
#76745=CARTESIAN_POINT ( 'NONE',  ( 114.6444261855608175, -117.4034471599418055, -11.78219314458159239 ) ) ;
#76783=VERTEX_POINT ( 'NONE', #57098 ) ;
#76796=ORIENTED_EDGE ( 'NONE', *, *, #17170, .F. ) ;
#76797=VECTOR ( 'NONE', #51932, 1000.000000000000000 ) ;
#76804=AXIS2_PLACEMENT_3D ( 'NONE', #67406, #47851, #66969 ) ;
#76807=DIRECTION ( 'NONE',  ( -1.087812297297669405E-15, 1.000000000000000000, -3.100000000000000044E-14 ) ) ;
#76810=( NAMED_UNIT ( * ) SI_UNIT ( $, .STERADIAN. ) SOLID_ANGLE_UNIT ( ) );
#76818=DIRECTION ( 'NONE',  ( 1.075267683398002218E-15, -1.000000000000000000, 3.100000000000000044E-14 ) ) ;
#76823=CARTESIAN_POINT ( 'NONE',  ( 76.06670390244703128, -104.2784471599409812, 45.21780685541799727 ) ) ;
#76827=CARTESIAN_POINT ( 'NONE',  ( 74.06670390244701707, -90.27844715994098124, 230.7030882296565721 ) ) ;
#76838=CARTESIAN_POINT ( 'NONE',  ( 69.57145439714845736, -138.4421226178978941, 247.5996244233720063 ) ) ;
#76843=VECTOR ( 'NONE', #69870, 1000.000000000000000 ) ;
#76868=DIRECTION ( 'NONE',  ( 3.100000000000000258E-29, -3.100000000000000044E-14, -1.000000000000000000 ) ) ;
#76876=EDGE_LOOP ( 'NONE', ( #16217, #10329, #80094, #49378, #34630, #61573 ) ) ;
#76906=DIRECTION ( 'NONE',  ( -0.7967329428042217998, 0.6043315462976631691, -1.908195823574488750E-14 ) ) ;
#76919=CARTESIAN_POINT ( 'NONE',  ( 68.71165106495583075, -139.2855573909722011, 245.9906543998875748 ) ) ;
#76920=DIRECTION ( 'NONE',  ( 1.000000000000000000, 0.000000000000000000, 0.000000000000000000 ) ) ;
#76921=CARTESIAN_POINT ( 'NONE',  ( 107.0667039024470313, -104.2784471599409528, 55.21780685541800437 ) ) ;
#76941=ORIENTED_EDGE ( 'NONE', *, *, #80928, .F. ) ;
#76955=VECTOR ( 'NONE', #46672, 1000.000000000000000 ) ;
#76966=CARTESIAN_POINT ( 'NONE',  ( 107.0667039024470313, -104.2784471599413934, 2.217806855418003043 ) ) ;
#76969=CARTESIAN_POINT ( 'NONE',  ( 67.07577529756494528, -67.88575619384793924, 245.6832122914381387 ) ) ;
#76971=EDGE_LOOP ( 'NONE', ( #65965, #85522, #82600, #31674, #62263, #53275 ) ) ;
#77049=DIRECTION ( 'NONE',  ( 0.000000000000000000, 0.000000000000000000, 1.000000000000000000 ) ) ;
#77054=LINE ( 'NONE', #22103, #84295 ) ;
#77059=ORIENTED_EDGE ( 'NONE', *, *, #28715, .F. ) ;
#77065=LINE ( 'NONE', #13935, #74523 ) ;
#77074=VERTEX_POINT ( 'NONE', #44257 ) ;
#77081=DIRECTION ( 'NONE',  ( 1.000000000000000000, 0.000000000000000000, 0.000000000000000000 ) ) ;
#77092=VECTOR ( 'NONE', #76807, 1000.000000000000000 ) ;
#77101=VERTEX_POINT ( 'NONE', #73762 ) ;
#77111=ORIENTED_EDGE ( 'NONE', *, *, #69816, .F. ) ;
#77122=CIRCLE ( 'NONE', #23458, 8.999999999999994671 ) ;
#77155=AXIS2_PLACEMENT_3D ( 'NONE', #34006, #81745, #54879 ) ;
#77156=CARTESIAN_POINT ( 'NONE',  ( 115.5439452383992176, -108.5954344580491551, 2.217806855418142042 ) ) ;
#77167=CARTESIAN_POINT ( 'NONE',  ( 93.91125933621933086, -96.68314769832107913, -11.78219314458223188 ) ) ;
#77168=DIRECTION ( 'NONE',  ( 1.000000000000000000, 1.122464679914735423E-15, 0.000000000000000000 ) ) ;
#77171=CARTESIAN_POINT ( 'NONE',  ( 56.06670390244699576, -67.87844715994098976, 85.21780685541799016 ) ) ;
#77187=AXIS2_PLACEMENT_3D ( 'NONE', #52738, #67756, #53644 ) ;
#77192=EDGE_CURVE ( 'NONE', #42534, #73518, #48216, .T. ) ;
#77204=CARTESIAN_POINT ( 'NONE',  ( 95.56670390244703128, -104.2784471599411660, 7.717806855417980394 ) ) ;
#77214=CIRCLE ( 'NONE', #22115, 17.00000000000000000 ) ;
#77229=CARTESIAN_POINT ( 'NONE',  ( 144.2411641744344593, -140.0674981546435163, 246.8991607896899723 ) ) ;
#77233=CARTESIAN_POINT ( 'NONE',  ( 121.2221484686747459, -113.6057974291316839, -19.26696060647573105 ) ) ;
#77256=DIRECTION ( 'NONE',  ( 1.000000000000000000, 0.000000000000000000, 0.000000000000000000 ) ) ;
#77311=ORIENTED_EDGE ( 'NONE', *, *, #23231, .T. ) ;
#77367=CARTESIAN_POINT ( 'NONE',  ( 154.5667039024469886, -67.87844715994090450, 120.2178068554179902 ) ) ;
#77369=LINE ( 'NONE', #41929, #56419 ) ;
#77384=ORIENTED_EDGE ( 'NONE', *, *, #16078, .F. ) ;
#77388=FACE_OUTER_BOUND ( 'NONE', #64885, .T. ) ;
#77389=ORIENTED_EDGE ( 'NONE', *, *, #51404, .T. ) ;
#77391=LINE ( 'NONE', #50111, #33017 ) ;
#77394=PLANE ( 'NONE',  #21101 ) ;
#77402=ORIENTED_EDGE ( 'NONE', *, *, #60323, .T. ) ;
#77409=DIRECTION ( 'NONE',  ( 0.000000000000000000, 0.000000000000000000, 1.000000000000000000 ) ) ;
#77413=CARTESIAN_POINT ( 'NONE',  ( 67.08803875813310924, -67.89720537647744436, 245.7828803018591657 ) ) ;
#77428=CONICAL_SURFACE ( 'NONE', #36778, 16.25000000000000000, 0.5235987755982992597 ) ;
#77436=B_SPLINE_CURVE_WITH_KNOTS ( 'NONE', 3,
 ( #17125, #4829, #38887, #17565, #87949, #10302 ),
 .UNSPECIFIED., .F., .F.,
 ( 4, 1, 1, 4 ),
 ( -7.513558482637090030, -5.399388959130909882, -4.342301322120899698, -0.1139565347578015420 ),
 .UNSPECIFIED. ) ;
#77515=EDGE_LOOP ( 'NONE', ( #41392, #48702, #15034, #86660 ) ) ;
#77526=CARTESIAN_POINT ( 'NONE',  ( 147.0665874381622018, -67.87844715994090450, 245.5130140176639770 ) ) ;
#77567=EDGE_CURVE ( 'NONE', #55635, #42534, #42799, .T. ) ;
#77579=EDGE_CURVE ( 'NONE', #77633, #19525, #8308, .T. ) ;
#77590=DIRECTION ( 'NONE',  ( -3.100000000000000258E-29, 3.100000000000000044E-14, 1.000000000000000000 ) ) ;
#77593=CARTESIAN_POINT ( 'NONE',  ( 107.0667039024470313, -104.2784471599421323, -21.78219314458201694 ) ) ;
#77603=EDGE_CURVE ( 'NONE', #56720, #65259, #16416, .T. ) ;
#77608=ORIENTED_EDGE ( 'NONE', *, *, #23771, .T. ) ;
#77626=PLANE ( 'NONE',  #3730 ) ;
#77633=VERTEX_POINT ( 'NONE', #47617 ) ;
#77639=CARTESIAN_POINT ( 'NONE',  ( 147.0667039024469886, -67.87844715994090450, 222.2178068554179902 ) ) ;
#77652=ORIENTED_EDGE ( 'NONE', *, *, #61511, .F. ) ;
#77660=CARTESIAN_POINT ( 'NONE',  ( 147.1762241153655282, -83.77844715994089597, 222.2178068554179902 ) ) ;
#77663=EDGE_LOOP ( 'NONE', ( #53064, #50795, #46645 ) ) ;
#77665=CARTESIAN_POINT ( 'NONE',  ( 128.8167039024470455, -104.2784471599409244, 19.21780685541800437 ) ) ;
#77671=ORIENTED_EDGE ( 'NONE', *, *, #25886, .F. ) ;
#77687=DIRECTION ( 'NONE',  ( -1.000000000000000000, -8.163404592832032979E-16, 0.000000000000000000 ) ) ;
#77692=CARTESIAN_POINT ( 'NONE',  ( 106.5667039024470171, -94.77844715994137914, 2.217806855417697953 ) ) ;
#77700=ORIENTED_EDGE ( 'NONE', *, *, #10620, .T. ) ;
#77703=DIRECTION ( 'NONE',  ( 0.8660254037844382635, 0.5000000000000008882, -1.550000000000000022E-14 ) ) ;
#77704=ORIENTED_EDGE ( 'NONE', *, *, #29802, .T. ) ;
#77707=ORIENTED_EDGE ( 'NONE', *, *, #19754, .F. ) ;
#77714=VECTOR ( 'NONE', #21999, 1000.000000000000000 ) ;
#77715=CIRCLE ( 'NONE', #80560, 8.999999999999994671 ) ;
#77716=SURFACE_STYLE_USAGE ( .BOTH. , #8679 ) ;
#77735=AXIS2_PLACEMENT_3D ( 'NONE', #1424, #37276, #44069 ) ;
#77766=CARTESIAN_POINT ( 'NONE',  ( 142.0294495518149915, -69.53963562688741717, 247.5178273157324327 ) ) ;
#77775=CIRCLE ( 'NONE', #12477, 4.500000000000003553 ) ;
#77776=DIRECTION ( 'NONE',  ( -9.437404618277395057E-08, 0.000000000000000000, -0.9999999999999955591 ) ) ;
#77795=VECTOR ( 'NONE', #23888, 1000.000000000000000 ) ;
#77797=ADVANCED_FACE ( 'NONE', ( #379 ), #830, .F. ) ;
#77809=CARTESIAN_POINT ( 'NONE',  ( 70.82666682523679924, -139.1379245046460085, 247.4850519812006553 ) ) ;
#77812=EDGE_LOOP ( 'NONE', ( #49677, #86489, #5821, #26872 ) ) ;
#77817=DIRECTION ( 'NONE',  ( 1.000000000000000000, 1.000000000000000078E-15, 0.000000000000000000 ) ) ;
#77819=CARTESIAN_POINT ( 'NONE',  ( 68.73082703990547770, -139.2670877096359447, 246.1201790234991620 ) ) ;
#77823=ADVANCED_FACE ( 'NONE', ( #22188 ), #83965, .F. ) ;
#77825=EDGE_CURVE ( 'NONE', #18276, #37103, #70321, .T. ) ;
#77826=CARTESIAN_POINT ( 'NONE',  ( 140.0667039024470171, -90.27844715994091018, 51.21780685541800437 ) ) ;
#77827=DIRECTION ( 'NONE',  ( -0.8660254037844389297, 0.4999999999999993894, -1.550000000000000968E-14 ) ) ;
#77830=CARTESIAN_POINT ( 'NONE',  ( 86.72755763596096301, -122.7870702624433648, 250.2178068554179902 ) ) ;
#77850=LINE ( 'NONE', #71042, #43977 ) ;
#77853=CARTESIAN_POINT ( 'NONE',  ( 146.4789389236947557, -138.2662121386931062, 245.5138901987649831 ) ) ;
#77859=EDGE_CURVE ( 'NONE', #63478, #46794, #68979, .T. ) ;
#77865=LINE ( 'NONE', #21106, #59558 ) ;
#77866=DIRECTION ( 'NONE',  ( 1.000000000000000078E-15, -1.000000000000000000, 0.000000000000000000 ) ) ;
#77868=PLANE ( 'NONE',  #50334 ) ;
#77870=CARTESIAN_POINT ( 'NONE',  ( 67.10568820078560748, -67.91409804406747242, 245.8838271276815988 ) ) ;
#77888=ORIENTED_EDGE ( 'NONE', *, *, #86615, .T. ) ;
#77899=EDGE_LOOP ( 'NONE', ( #17592, #71687, #11289, #82935 ) ) ;
#77907=ADVANCED_FACE ( 'NONE', ( #20829 ), #62603, .F. ) ;
#77922=AXIS2_PLACEMENT_3D ( 'NONE', #31750, #37691, #44927 ) ;
#77952=CARTESIAN_POINT ( 'NONE',  ( 146.0667039024470171, -94.02844715994091018, 45.21780685541799727 ) ) ;
#77965=DIRECTION ( 'NONE',  ( 1.000000000000000000, 0.000000000000000000, 0.000000000000000000 ) ) ;
#77966=CIRCLE ( 'NONE', #14079, 23.50000000000000711 ) ;
#77969=VERTEX_POINT ( 'NONE', #52517 ) ;
#77972=AXIS2_PLACEMENT_3D ( 'NONE', #60610, #88353, #62853 ) ;
#77975=VECTOR ( 'NONE', #89728, 1000.000000000000000 ) ;
#78005=CARTESIAN_POINT ( 'NONE',  ( 107.5667039024470313, -100.3098201933451605, -19.78219314458212708 ) ) ;
#78007=VECTOR ( 'NONE', #7440, 1000.000000000000114 ) ;
#78031=ORIENTED_EDGE ( 'NONE', *, *, #41875, .F. ) ;
#78033=CARTESIAN_POINT ( 'NONE',  ( 99.53451269431035087, -109.2045100507364737, 2.217806855418169576 ) ) ;
#78045=EDGE_LOOP ( 'NONE', ( #39760, #7190, #54067, #56598 ) ) ;
#78046=DIRECTION ( 'NONE',  ( 3.100000000000000258E-29, -3.100000000000000044E-14, -1.000000000000000000 ) ) ;
#78050=LINE ( 'NONE', #1741, #28195 ) ;
#78053=ADVANCED_FACE ( 'NONE', ( #3956 ), #51197, .T. ) ;
#78066=DIRECTION ( 'NONE',  ( 1.000000000000000078E-15, -1.000000000000000000, 0.000000000000000000 ) ) ;
#78075=DIRECTION ( 'NONE',  ( -0.8660254037844382635, -0.5000000000000008882, 1.550000000000000022E-14 ) ) ;
#78082=VERTEX_POINT ( 'NONE', #64849 ) ;
#78089=CARTESIAN_POINT ( 'NONE',  ( 77.06670390244701707, -90.27844715994098124, 222.2178068554179902 ) ) ;
#78096=VECTOR ( 'NONE', #7449, 1000.000000000000000 ) ;
#78098=( BOUNDED_CURVE ( )  B_SPLINE_CURVE ( 3, ( #66143, #11649, #31627, #45679 ),
 .UNSPECIFIED., .F., .F. ) 
 B_SPLINE_CURVE_WITH_KNOTS ( ( 4, 4 ),
 ( 5.813027347256380040, 6.283185307179586232 ),
 .UNSPECIFIED. ) 
 CURVE ( )  GEOMETRIC_REPRESENTATION_ITEM ( )  RATIONAL_B_SPLINE_CURVE ( ( 1.000000000000000000, 0.9816639655796099984, 0.9816639655796099984, 1.000000000000000000 ) ) 
 REPRESENTATION_ITEM ( '' )  );
#78112=VERTEX_POINT ( 'NONE', #46614 ) ;
#78123=LINE ( 'NONE', #15884, #27658 ) ;
#78127=LINE ( 'NONE', #71305, #85041 ) ;
#78134=ORIENTED_EDGE ( 'NONE', *, *, #31285, .T. ) ;
#78151=ORIENTED_EDGE ( 'NONE', *, *, #86425, .F. ) ;
#78155=DIRECTION ( 'NONE',  ( 1.000000000000000000, 1.000000000000000078E-15, 0.000000000000000000 ) ) ;
#78162=ORIENTED_EDGE ( 'NONE', *, *, #89792, .T. ) ;
#78168=EDGE_CURVE ( 'NONE', #54510, #22506, #62885, .T. ) ;
#78171=ORIENTED_EDGE ( 'NONE', *, *, #71952, .T. ) ;
#78203=CARTESIAN_POINT ( 'NONE',  ( 107.0667039024470313, -104.2784471599409102, 17.71780685541799016 ) ) ;
#78224=CARTESIAN_POINT ( 'NONE',  ( 106.0667039024470171, -87.35579742913164125, -19.26696060647653397 ) ) ;
#78225=VERTEX_POINT ( 'NONE', #26192 ) ;
#78229=DIRECTION ( 'NONE',  ( 1.000000000000000078E-15, -1.000000000000000000, 0.000000000000000000 ) ) ;
#78251=DIRECTION ( 'NONE',  ( 1.000000000000000000, 1.132880637372608296E-15, 0.000000000000000000 ) ) ;
#78252=ORIENTED_EDGE ( 'NONE', *, *, #36168, .F. ) ;
#78255=VERTEX_POINT ( 'NONE', #41589 ) ;
#78256=ORIENTED_EDGE ( 'NONE', *, *, #16404, .T. ) ;
#78266=ORIENTED_EDGE ( 'NONE', *, *, #46994, .F. ) ;
#78270=EDGE_CURVE ( 'NONE', #75751, #4284, #55208, .T. ) ;
#78279=CARTESIAN_POINT ( 'NONE',  ( 140.0667039024470171, -90.27844715994091018, 222.2178068554179902 ) ) ;
#78287=FACE_BOUND ( 'NONE', #6663, .T. ) ;
#78294=CARTESIAN_POINT ( 'NONE',  ( 85.06670390244701707, -80.35669973212957018, 55.21780685541800437 ) ) ;
#78304=VECTOR ( 'NONE', #44688, 1000.000000000000000 ) ;
#78307=DIRECTION ( 'NONE',  ( -1.000000000000000078E-15, 1.000000000000000000, 0.000000000000000000 ) ) ;
#78359=VERTEX_POINT ( 'NONE', #1179 ) ;
#78369=AXIS2_PLACEMENT_3D ( 'NONE', #68283, #20583, #6063 ) ;
#78376=CARTESIAN_POINT ( 'NONE',  ( 74.25553510437300986, -77.53446767201269552, 248.3919653347779786 ) ) ;
#78381=AXIS2_PLACEMENT_3D ( 'NONE', #38142, #2745, #70895 ) ;
#78384=EDGE_LOOP ( 'NONE', ( #44043, #3858, #1569, #3022 ) ) ;
#78420=DIRECTION ( 'NONE',  ( -0.7349399772593263602, 0.6687953793059858709, 0.1121426343770439427 ) ) ;
#78436=LINE ( 'NONE', #31141, #52759 ) ;
#78447=LINE ( 'NONE', #78886, #32210 ) ;
#78457=ORIENTED_EDGE ( 'NONE', *, *, #30139, .F. ) ;
#78462=AXIS2_PLACEMENT_3D ( 'NONE', #64459, #8611, #23150 ) ;
#78474=CARTESIAN_POINT ( 'NONE',  ( 68.06670390244701707, -86.77844715994098124, 45.21780685541799727 ) ) ;
#78484=DIRECTION ( 'NONE',  ( 0.000000000000000000, 0.000000000000000000, -1.000000000000000000 ) ) ;
#78485=ORIENTED_EDGE ( 'NONE', *, *, #53180, .F. ) ;
#78490=DIRECTION ( 'NONE',  ( 0.000000000000000000, 0.000000000000000000, 1.000000000000000000 ) ) ;
#78500=ORIENTED_EDGE ( 'NONE', *, *, #23594, .F. ) ;
#78529=FACE_OUTER_BOUND ( 'NONE', #51116, .T. ) ;
#78534=EDGE_CURVE ( 'NONE', #9292, #87042, #58535, .T. ) ;
#78546=CIRCLE ( 'NONE', #5980, 121.3994834559399862 ) ;
#78562=ORIENTED_EDGE ( 'NONE', *, *, #25147, .T. ) ;
#78564=ORIENTED_EDGE ( 'NONE', *, *, #58899, .F. ) ;
#78596=CARTESIAN_POINT ( 'NONE',  ( 77.06670390244703128, -118.2784471599409812, 222.2178068554179902 ) ) ;
#78620=DIRECTION ( 'NONE',  ( 0.8660254037844382635, 0.5000000000000008882, -1.550000000000000022E-14 ) ) ;
#78639=DIRECTION ( 'NONE',  ( 3.100000000000000258E-29, -3.100000000000000044E-14, -1.000000000000000000 ) ) ;
#78651=CARTESIAN_POINT ( 'NONE',  ( 59.56670390244699576, -67.87844715994098976, 120.2178068554179902 ) ) ;
#78662=ORIENTED_EDGE ( 'NONE', *, *, #28715, .T. ) ;
#78674=DIRECTION ( 'NONE',  ( 1.000000000000000000, 8.953411488912556626E-16, 0.000000000000000000 ) ) ;
#78696=LINE ( 'NONE', #57769, #58152 ) ;
#78712=AXIS2_PLACEMENT_3D ( 'NONE', #20853, #35813, #407 ) ;
#78726=EDGE_CURVE ( 'NONE', #41047, #9127, #32886, .T. ) ;
#78728=CARTESIAN_POINT ( 'NONE',  ( 69.36306272520799610, -138.6409717137631503, 247.3638974706309455 ) ) ;
#78733=EDGE_CURVE ( 'NONE', #88193, #9096, #69232, .T. ) ;
#78735=FACE_BOUND ( 'NONE', #17105, .T. ) ;
#78760=CARTESIAN_POINT ( 'NONE',  ( 110.7536356736639220, -105.8297479413482733, -19.78219314458196010 ) ) ;
#78823=VERTEX_POINT ( 'NONE', #41042 ) ;
#78828=CARTESIAN_POINT ( 'NONE',  ( 143.5397427877413747, -139.6742706447616058, 247.2684776741174062 ) ) ;
#78843=ADVANCED_FACE ( 'NONE', ( #62828 ), #21061, .F. ) ;
#78867=DIRECTION ( 'NONE',  ( -1.000000000000000078E-15, 1.000000000000000000, 0.000000000000000000 ) ) ;
#78880=DIRECTION ( 'NONE',  ( -0.8660254037844380415, -0.5000000000000012212, 1.550000000000001284E-14 ) ) ;
#78881=DIRECTION ( 'NONE',  ( -3.100000000000000258E-29, 3.100000000000000044E-14, 1.000000000000000000 ) ) ;
#78886=CARTESIAN_POINT ( 'NONE',  ( 77.06670390244703128, -118.2784471599409812, 230.7030882296565721 ) ) ;
#78890=AXIS2_PLACEMENT_3D ( 'NONE', #21201, #84343, #22112 ) ;
#78894=ORIENTED_EDGE ( 'NONE', *, *, #66208, .T. ) ;
#78901=CARTESIAN_POINT ( 'NONE',  ( 97.81670390244700286, -68.87844715994096134, 55.21780685541800437 ) ) ;
#78924=EDGE_LOOP ( 'NONE', ( #40984, #32672, #22816, #56245 ) ) ;
#78927=CYLINDRICAL_SURFACE ( 'NONE', #37753, 3.499999999999996003 ) ;
#78935=DIRECTION ( 'NONE',  ( 0.000000000000000000, 0.000000000000000000, 1.000000000000000000 ) ) ;
#78958=ORIENTED_EDGE ( 'NONE', *, *, #24995, .F. ) ;
#78959=EDGE_CURVE ( 'NONE', #42534, #9271, #85096, .T. ) ;
#78967=DIRECTION ( 'NONE',  ( -0.7071067811865473507, -0.7071067811865477948, 0.000000000000000000 ) ) ;
#79003=CARTESIAN_POINT ( 'NONE',  ( 68.82702071641912767, -69.48851445456057263, 247.4865261645284136 ) ) ;
#79019=VECTOR ( 'NONE', #35041, 1000.000000000000000 ) ;
#79033=CARTESIAN_POINT ( 'NONE',  ( 154.5667039024470171, -79.67844715994088745, 120.2178068554179902 ) ) ;
#79063=DIRECTION ( 'NONE',  ( -3.100000000000000258E-29, 3.100000000000000044E-14, 1.000000000000000000 ) ) ;
#79069=CARTESIAN_POINT ( 'NONE',  ( 106.5667039024470171, -94.77844715994137914, 2.217806855417697953 ) ) ;
#79074=DIRECTION ( 'NONE',  ( -1.000000000000000000, -8.953411488912552682E-16, 0.000000000000000000 ) ) ;
#79078=VECTOR ( 'NONE', #18160, 1000.000000000000000 ) ;
#79105=ORIENTED_EDGE ( 'NONE', *, *, #68766, .T. ) ;
#79117=CARTESIAN_POINT ( 'NONE',  ( 107.0667039024470313, -104.2784471599409528, 45.21780685541799727 ) ) ;
#79132=CARTESIAN_POINT ( 'NONE',  ( 107.0667039024470171, -79.67844715994094429, 138.7178068554180186 ) ) ;
#79156=ORIENTED_EDGE ( 'NONE', *, *, #88312, .F. ) ;
#79157=VECTOR ( 'NONE', #89919, 999.9999999999998863 ) ;
#79171=CARTESIAN_POINT ( 'NONE',  ( 69.38693536744452217, -138.6172649514752777, 247.3844049223929176 ) ) ;
#79179=LINE ( 'NONE', #71018, #23987 ) ;
#79190=CIRCLE ( 'NONE', #11005, 7.999999999999992895 ) ;
#79202=LINE ( 'NONE', #65104, #64489 ) ;
#79206=VERTEX_POINT ( 'NONE', #10015 ) ;
#79216=PLANE ( 'NONE',  #66906 ) ;
#79222=EDGE_LOOP ( 'NONE', ( #50525, #84060, #4764, #82865 ) ) ;
#79225=CARTESIAN_POINT ( 'NONE',  ( 147.0183410955044678, -67.92213675950819152, 245.9229835953497911 ) ) ;
#79248=ORIENTED_EDGE ( 'NONE', *, *, #85795, .F. ) ;
#79261=CARTESIAN_POINT ( 'NONE',  ( 73.74475183977565962, -128.3542712181327943, 248.3919653347779786 ) ) ;
#79267=AXIS2_PLACEMENT_3D ( 'NONE', #20997, #48673, #78674 ) ;
#79277=CARTESIAN_POINT ( 'NONE',  ( 143.7785205373602082, -140.1898562409545548, 246.8437313719147994 ) ) ;
#79284=CARTESIAN_POINT ( 'NONE',  ( 67.97654527815089409, -137.2003834803944926, 247.1835444442183984 ) ) ;
#79313=DIRECTION ( 'NONE',  ( -3.100000000000000258E-29, 3.100000000000000044E-14, 1.000000000000000000 ) ) ;
#79317=ORIENTED_EDGE ( 'NONE', *, *, #72281, .F. ) ;
#79325=CARTESIAN_POINT ( 'NONE',  ( 107.0667039024470313, -104.2784471599420755, -19.78219314458201694 ) ) ;
#79346=ORIENTED_EDGE ( 'NONE', *, *, #58210, .T. ) ;
#79349=EDGE_CURVE ( 'NONE', #36478, #55038, #7909, .T. ) ;
#79350=DIRECTION ( 'NONE',  ( 3.100000000000000258E-29, -3.100000000000000044E-14, -1.000000000000000000 ) ) ;
#79356=AXIS2_PLACEMENT_3D ( 'NONE', #46596, #82507, #61574 ) ;
#79357=EDGE_CURVE ( 'NONE', #56828, #56526, #46447, .T. ) ;
#79373=DIRECTION ( 'NONE',  ( -1.000000000000000000, -1.000000000000000078E-15, 0.000000000000000000 ) ) ;
#79390=CARTESIAN_POINT ( 'NONE',  ( 102.3035641816324102, -119.0284471599421181, -21.78219314458157285 ) ) ;
#79391=CARTESIAN_POINT ( 'NONE',  ( 86.71802151318415497, -122.7425185119399629, 250.2203867545810283 ) ) ;
#79395=CIRCLE ( 'NONE', #6810, 7.999999999999992895 ) ;
#79404=FACE_OUTER_BOUND ( 'NONE', #29641, .T. ) ;
#79449=VERTEX_POINT ( 'NONE', #51767 ) ;
#79464=CYLINDRICAL_SURFACE ( 'NONE', #15465, 1.999999999999995781 ) ;
#79471=EDGE_CURVE ( 'NONE', #2833, #4111, #60823, .T. ) ;
#79488=CARTESIAN_POINT ( 'NONE',  ( 63.06670390244699576, -67.87844715994098976, 190.2178068554179902 ) ) ;
#79489=CARTESIAN_POINT ( 'NONE',  ( 107.0667039024470313, -104.2784471599413791, 2.217806855418003043 ) ) ;
#79492=CARTESIAN_POINT ( 'NONE',  ( 81.84766347661002328, -83.77844715994096703, 45.21780685541799727 ) ) ;
#79533=ORIENTED_EDGE ( 'NONE', *, *, #46360, .T. ) ;
#79534=VECTOR ( 'NONE', #70610, 1000.000000000000000 ) ;
#79541=FACE_OUTER_BOUND ( 'NONE', #34083, .T. ) ;
#79547=CARTESIAN_POINT ( 'NONE',  ( 91.91441891875203396, -96.57077177933014411, -21.78219314458226918 ) ) ;
#79554=PLANE ( 'NONE',  #55130 ) ;
#79560=ORIENTED_EDGE ( 'NONE', *, *, #4463, .T. ) ;
#79561=FACE_BOUND ( 'NONE', #55561, .T. ) ;
#79569=ORIENTED_EDGE ( 'NONE', *, *, #73887, .T. ) ;
#79576=DIRECTION ( 'NONE',  ( 1.000000000000000000, 1.132880637372608296E-15, 0.000000000000000000 ) ) ;
#79582=ORIENTED_EDGE ( 'NONE', *, *, #9319, .F. ) ;
#79606=CARTESIAN_POINT ( 'NONE',  ( 102.3035641816324102, -119.0284471599421181, -21.78219314458157285 ) ) ;
#79619=DIRECTION ( 'NONE',  ( 1.000000000000000000, 0.000000000000000000, 0.000000000000000000 ) ) ;
#79620=FACE_BOUND ( 'NONE', #47582, .T. ) ;
#79631=EDGE_CURVE ( 'NONE', #52525, #13042, #84777, .T. ) ;
#79635=EDGE_CURVE ( 'NONE', #39084, #27685, #32523, .T. ) ;
#79642=DIRECTION ( 'NONE',  ( 3.100000000000000258E-29, -3.100000000000000044E-14, -1.000000000000000000 ) ) ;
#79644=ADVANCED_FACE ( 'NONE', ( #74919 ), #40386, .T. ) ;
#79645=AXIS2_PLACEMENT_3D ( 'NONE', #56450, #56907, #84643 ) ;
#79647=CARTESIAN_POINT ( 'NONE',  ( 145.3020554092476857, -139.4430956531403183, 245.6798494796449859 ) ) ;
#79653=VECTOR ( 'NONE', #314, 1000.000000000000000 ) ;
#79668=ORIENTED_EDGE ( 'NONE', *, *, #52220, .F. ) ;
#79672=FACE_OUTER_BOUND ( 'NONE', #81460, .T. ) ;
#79697=VERTEX_POINT ( 'NONE', #22997 ) ;
#79710=ORIENTED_EDGE ( 'NONE', *, *, #3984, .T. ) ;
#79720=DIRECTION ( 'NONE',  ( 0.000000000000000000, -0.000000000000000000, 1.000000000000000000 ) ) ;
#79721=DIRECTION ( 'NONE',  ( -3.100000000000000258E-29, 3.100000000000000044E-14, 1.000000000000000000 ) ) ;
#79728=CARTESIAN_POINT ( 'NONE',  ( 68.08801065749622694, -137.1506278873062286, 247.2512423094629810 ) ) ;
#79729=( GEOMETRIC_REPRESENTATION_CONTEXT ( 3 ) GLOBAL_UNCERTAINTY_ASSIGNED_CONTEXT ( ( #56901 ) ) GLOBAL_UNIT_ASSIGNED_CONTEXT ( ( #69550, #21405, #76810 ) ) REPRESENTATION_CONTEXT ( 'NONE', 'WORKASPACE' ) );
#79744=DIRECTION ( 'NONE',  ( 1.000000000000000000, 1.000000000000000078E-15, 0.000000000000000000 ) ) ;
#79756=DIRECTION ( 'NONE',  ( -3.100000000000000258E-29, 3.100000000000000044E-14, 1.000000000000000000 ) ) ;
#79757=EDGE_CURVE ( 'NONE', #63429, #36556, #23449, .T. ) ;
#79765=ADVANCED_FACE ( 'NONE', ( #39277 ), #68334, .F. ) ;
#79785=ADVANCED_FACE ( 'NONE', ( #74256 ), #40618, .F. ) ;
#79787=CIRCLE ( 'NONE', #40586, 3.499999999999996003 ) ;
#79789=ORIENTED_EDGE ( 'NONE', *, *, #70642, .T. ) ;
#79824=CARTESIAN_POINT ( 'NONE',  ( 111.8298436232616240, -89.52844715994213232, -21.78219314458246103 ) ) ;
#79841=AXIS2_PLACEMENT_3D ( 'NONE', #34130, #81427, #20077 ) ;
#79850=EDGE_CURVE ( 'NONE', #4517, #18229, #18379, .T. ) ;
#79862=FACE_OUTER_BOUND ( 'NONE', #70250, .T. ) ;
#79872=ORIENTED_EDGE ( 'NONE', *, *, #53543, .F. ) ;
#79907=CARTESIAN_POINT ( 'NONE',  ( 89.90578320442969584, -68.21248437868196390, 247.0699965152190032 ) ) ;
#79943=CARTESIAN_POINT ( 'NONE',  ( 143.2522959336310748, -139.0102598546870922, 247.5112310255240118 ) ) ;
#79949=AXIS2_PLACEMENT_3D ( 'NONE', #58475, #86206, #52533 ) ;
#79962=LINE ( 'NONE', #4976, #63153 ) ;
#79971=ADVANCED_FACE ( 'NONE', ( #7298 ), #15006, .T. ) ;
#79981=EDGE_CURVE ( 'NONE', #29010, #11533, #5291, .T. ) ;
#79991=DIRECTION ( 'NONE',  ( 1.000000000000000000, 0.000000000000000000, 0.000000000000000000 ) ) ;
#80000=ORIENTED_EDGE ( 'NONE', *, *, #18263, .T. ) ;
#80009=CARTESIAN_POINT ( 'NONE',  ( 70.06670417066791856, -83.77844715994098124, 55.21780685541800437 ) ) ;
#80020=ORIENTED_EDGE ( 'NONE', *, *, #54600, .T. ) ;
#80038=DIRECTION ( 'NONE',  ( 0.000000000000000000, 0.000000000000000000, 1.000000000000000000 ) ) ;
#80044=FACE_OUTER_BOUND ( 'NONE', #10001, .T. ) ;
#80063=CARTESIAN_POINT ( 'NONE',  ( 139.9417039024470455, -127.9034471599408960, 55.21780685541800437 ) ) ;
#80088=DIRECTION ( 'NONE',  ( -0.000000000000000000, -0.000000000000000000, -1.000000000000000000 ) ) ;
#80090=AXIS2_PLACEMENT_3D ( 'NONE', #68477, #53461, #68021 ) ;
#80094=ORIENTED_EDGE ( 'NONE', *, *, #16515, .T. ) ;
#80099=CARTESIAN_POINT ( 'NONE',  ( 118.5667039024470313, -104.2784471599411376, 7.717806855417980394 ) ) ;
#80103=DIRECTION ( 'NONE',  ( 1.000000000000000000, 1.000000000000000078E-15, 0.000000000000000000 ) ) ;
#80111=ORIENTED_EDGE ( 'NONE', *, *, #89908, .F. ) ;
#80114=CARTESIAN_POINT ( 'NONE',  ( 107.0667039024470313, -104.2784471599420755, -19.78219314458201694 ) ) ;
#80124=EDGE_LOOP ( 'NONE', ( #62698, #75452, #47674, #6942, #39197 ) ) ;
#80133=CARTESIAN_POINT ( 'NONE',  ( 139.9417039024470171, -80.65344715994091018, 55.21780685541800437 ) ) ;
#80152=AXIS2_PLACEMENT_3D ( 'NONE', #16987, #22468, #10603 ) ;
#80172=CARTESIAN_POINT ( 'NONE',  ( 68.76053423562146349, -136.8603496727827746, 247.4879725229279757 ) ) ;
#80173=DIRECTION ( 'NONE',  ( 0.000000000000000000, 0.000000000000000000, 1.000000000000000000 ) ) ;
#80182=CARTESIAN_POINT ( 'NONE',  ( 110.2536356736639220, -106.6957733451327215, -19.78219314458193168 ) ) ;
#80183=DIRECTION ( 'NONE',  ( 0.000000000000000000, -0.000000000000000000, 1.000000000000000000 ) ) ;
#80186=LINE ( 'NONE', #72470, #34913 ) ;
#80194=ORIENTED_EDGE ( 'NONE', *, *, #81496, .T. ) ;
#80209=CARTESIAN_POINT ( 'NONE',  ( 115.5439452383991892, -99.96145986183427112, -19.78219314458215550 ) ) ;
#80225=AXIS2_PLACEMENT_3D ( 'NONE', #16457, #64606, #44137 ) ;
#80236=LINE ( 'NONE', #60198, #3757 ) ;
#80257=EDGE_LOOP ( 'NONE', ( #81833, #1602, #14923, #18786 ) ) ;
#80263=CARTESIAN_POINT ( 'NONE',  ( 147.0667039024469886, -67.87844716047348470, 245.4920193514540188 ) ) ;
#80295=DIRECTION ( 'NONE',  ( -3.100000000000000258E-29, 3.100000000000000044E-14, 1.000000000000000000 ) ) ;
#80304=DIRECTION ( 'NONE',  ( 0.000000000000000000, -0.000000000000000000, 1.000000000000000000 ) ) ;
#80305=CARTESIAN_POINT ( 'NONE',  ( 70.06684293446046752, -140.6784485900457753, 245.9352930260599805 ) ) ;
#80307=DIRECTION ( 'NONE',  ( -1.000000000000000000, 2.195856868753399715E-16, 0.000000000000000000 ) ) ;
#80325=EDGE_LOOP ( 'NONE', ( #25724, #28377, #78151, #72522, #86321, #12150, #76551, #25650, #72571, #42129, #16832, #33849, #8567, #29344, #22476, #47276, #38992, #78031 ) ) ;
#80342=CARTESIAN_POINT ( 'NONE',  ( 154.5667039024469886, -67.87844715994090450, 155.2178068554179902 ) ) ;
#80369=VECTOR ( 'NONE', #24028, 1000.000000000000000 ) ;
#80372=LINE ( 'NONE', #18121, #10693 ) ;
#80374=DIRECTION ( 'NONE',  ( 1.000000000000000078E-15, -1.000000000000000000, 0.000000000000000000 ) ) ;
#80377=EDGE_CURVE ( 'NONE', #65034, #70844, #67274, .T. ) ;
#80391=EDGE_CURVE ( 'NONE', #84281, #29010, #28317, .T. ) ;
#80401=CARTESIAN_POINT ( 'NONE',  ( 91.91125933621934507, -111.8737466215628160, -19.26696060647578435 ) ) ;
#80420=DIRECTION ( 'NONE',  ( -0.9217329428042198014, -0.3878251953515564066, 1.214306433183767175E-14 ) ) ;
#80428=EDGE_CURVE ( 'NONE', #16796, #87491, #31860, .T. ) ;
#80443=ORIENTED_EDGE ( 'NONE', *, *, #65811, .T. ) ;
#80448=PLANE ( 'NONE',  #15779 ) ;
#80456=ADVANCED_FACE ( 'NONE', ( #24609 ), #73191, .T. ) ;
#80476=VECTOR ( 'NONE', #69432, 1000.000000000000000 ) ;
#80477=CARTESIAN_POINT ( 'NONE',  ( 135.5667039024470171, -90.27844715994091018, 45.21780685541799727 ) ) ;
#80492=ORIENTED_EDGE ( 'NONE', *, *, #47258, .F. ) ;
#80500=DIRECTION ( 'NONE',  ( -3.100000000000000258E-29, 3.100000000000000044E-14, 1.000000000000000000 ) ) ;
#80502=CARTESIAN_POINT ( 'NONE',  ( 144.0667052733537901, -71.37844715994090450, 55.21780685541800437 ) ) ;
#80517=ORIENTED_EDGE ( 'NONE', *, *, #23231, .F. ) ;
#80528=CARTESIAN_POINT ( 'NONE',  ( 108.0667039024470455, -121.2010968907524529, -19.26696060647547881 ) ) ;
#80532=ORIENTED_EDGE ( 'NONE', *, *, #14096, .F. ) ;
#80539=CARTESIAN_POINT ( 'NONE',  ( 154.5667039024469886, -67.87844715994090450, 155.2178068554179902 ) ) ;
#80549=VERTEX_POINT ( 'NONE', #50410 ) ;
#80552=CARTESIAN_POINT ( 'NONE',  ( 136.4247830841161999, -74.33686277290898659, 248.4067532124560103 ) ) ;
#80553=CARTESIAN_POINT ( 'NONE',  ( 147.0665874381622018, -67.87844715994090450, 245.5130140176639770 ) ) ;
#80555=CARTESIAN_POINT ( 'NONE',  ( 106.1586424053105873, -87.30271670975442078, -11.78219314458253741 ) ) ;
#80560=AXIS2_PLACEMENT_3D ( 'NONE', #8369, #76508, #15637 ) ;
#80584=ORIENTED_EDGE ( 'NONE', *, *, #20397, .F. ) ;
#80608=CARTESIAN_POINT ( 'NONE',  ( 162.0667039024469886, -67.87844715994089029, 222.2178068554179902 ) ) ;
#80613=LINE ( 'NONE', #62826, #32281 ) ;
#80616=PLANE ( 'NONE',  #67707 ) ;
#80644=DIRECTION ( 'NONE',  ( -0.4999999999999994449, -0.8660254037844390407, 2.684678751731759347E-14 ) ) ;
#80654=LINE ( 'NONE', #51135, #89721 ) ;
#80660=CARTESIAN_POINT ( 'NONE',  ( 67.06681736700808472, -67.87844715931913697, 245.5130139978070076 ) ) ;
#80665=CARTESIAN_POINT ( 'NONE',  ( 107.0667039024470313, -104.2784471599409528, 24.21780685541800082 ) ) ;
#80673=DIRECTION ( 'NONE',  ( -3.100000000000000258E-29, 3.100000000000000044E-14, 1.000000000000000000 ) ) ;
#80705=CYLINDRICAL_SURFACE ( 'NONE', #79356, 3.499999999999996003 ) ;
#80721=VERTEX_POINT ( 'NONE', #5403 ) ;
#80737=EDGE_LOOP ( 'NONE', ( #41090, #2481 ) ) ;
#80743=CARTESIAN_POINT ( 'NONE',  ( 125.5177273812784193, -99.45575754528751133, 55.21780685541800437 ) ) ;
#80745=CARTESIAN_POINT ( 'NONE',  ( 70.45481371026527029, -138.5762527540429971, 247.5817532094160072 ) ) ;
#80748=ORIENTED_EDGE ( 'NONE', *, *, #46892, .F. ) ;
#80749=EDGE_LOOP ( 'NONE', ( #66850, #26949, #2264, #14094 ) ) ;
#80759=EDGE_CURVE ( 'NONE', #14739, #24467, #66262, .T. ) ;
#80777=EDGE_CURVE ( 'NONE', #41770, #35035, #39988, .T. ) ;
#80778=CARTESIAN_POINT ( 'NONE',  ( 100.4020455594773580, -99.85325460238202311, -19.78219314458215550 ) ) ;
#80798=EDGE_LOOP ( 'NONE', ( #38687, #65536, #60279, #71195 ) ) ;
#80812=VERTEX_POINT ( 'NONE', #11768 ) ;
#80833=DIRECTION ( 'NONE',  ( -1.000000000000000000, -8.163404592832032979E-16, 0.000000000000000000 ) ) ;
#80854=CARTESIAN_POINT ( 'NONE',  ( 91.91125933621934507, -111.9108492392177396, -19.23816774841976951 ) ) ;
#80856=ORIENTED_EDGE ( 'NONE', *, *, #74356, .T. ) ;
#80864=ORIENTED_EDGE ( 'NONE', *, *, #29449, .T. ) ;
#80867=ADVANCED_FACE ( 'NONE', ( #54856 ), #40802, .F. ) ;
#80877=VERTEX_POINT ( 'NONE', #69866 ) ;
#80878=LINE ( 'NONE', #25444, #50122 ) ;
#80887=AXIS2_PLACEMENT_3D ( 'NONE', #15435, #69941, #34956 ) ;
#80890=ADVANCED_FACE ( 'NONE', ( #61684 ), #7636, .F. ) ;
#80903=CARTESIAN_POINT ( 'NONE',  ( 80.55084967033837984, -151.1625929292324884, 73.15139425023529895 ) ) ;
#80909=ADVANCED_FACE ( 'NONE', ( #82619 ), #68968, .F. ) ;
#80926=ORIENTED_EDGE ( 'NONE', *, *, #57521, .F. ) ;
#80928=EDGE_CURVE ( 'NONE', #67043, #87073, #26284, .T. ) ;
#80946=DIRECTION ( 'NONE',  ( 0.000000000000000000, 0.000000000000000000, -1.000000000000000000 ) ) ;
#80966=CARTESIAN_POINT ( 'NONE',  ( 146.7395179759399184, -101.1118038811399913, 247.0601187889650134 ) ) ;
#80991=EDGE_CURVE ( 'NONE', #41462, #13431, #23525, .T. ) ;
#81003=PLANE ( 'NONE',  #16219 ) ;
#81005=CARTESIAN_POINT ( 'NONE',  ( 162.0667039024469886, -67.87844715994089029, 222.2178068554179902 ) ) ;
#81034=CARTESIAN_POINT ( 'NONE',  ( 96.20012047777625241, -115.5046222945369436, -21.78219314458165812 ) ) ;
#81038=CARTESIAN_POINT ( 'NONE',  ( 84.40120044323725779, -147.4828892783847607, 72.80491794383669912 ) ) ;
#81043=ORIENTED_EDGE ( 'NONE', *, *, #41883, .F. ) ;
#81050=CARTESIAN_POINT ( 'NONE',  ( 127.0667052882549797, -69.62844715994097555, 55.21780685541800437 ) ) ;
#81071=LINE ( 'NONE', #32888, #31240 ) ;
#81074=DIRECTION ( 'NONE',  ( -3.100000000000000258E-29, 3.100000000000000044E-14, 1.000000000000000000 ) ) ;
#81075=ORIENTED_EDGE ( 'NONE', *, *, #8791, .T. ) ;
#81082=CARTESIAN_POINT ( 'NONE',  ( 162.0667039024469886, -67.87844715994089029, 222.2178068554179902 ) ) ;
#81086=DIRECTION ( 'NONE',  ( 1.000000000000000078E-15, -1.000000000000000000, 0.000000000000000000 ) ) ;
#81094=AXIS2_PLACEMENT_3D ( 'NONE', #35400, #69495, #7272 ) ;
#81102=AXIS2_PLACEMENT_3D ( 'NONE', #34721, #84242, #62425 ) ;
#81112=CARTESIAN_POINT ( 'NONE',  ( 145.6286013927122553, -101.3636183722299222, 247.6387710704172491 ) ) ;
#81116=LINE ( 'NONE', #47439, #49520 ) ;
#81121=CARTESIAN_POINT ( 'NONE',  ( 67.06803645764867383, -67.87922922289656924, 245.5675989924858698 ) ) ;
#81126=DIRECTION ( 'NONE',  ( 1.000000000000000000, 1.276118419109374860E-15, 0.000000000000000000 ) ) ;
#81133=DIRECTION ( 'NONE',  ( 0.7759704746411385523, -0.6307692307692301936, 0.000000000000000000 ) ) ;
#81136=DIRECTION ( 'NONE',  ( -1.000000000000000000, -8.953411488912552682E-16, 0.000000000000000000 ) ) ;
#81163=AXIS2_PLACEMENT_3D ( 'NONE', #32891, #55101, #53758 ) ;
#81197=ORIENTED_EDGE ( 'NONE', *, *, #68486, .F. ) ;
#81205=CARTESIAN_POINT ( 'NONE',  ( 87.67246433899146041, -140.4240802520271529, 246.9378847324709909 ) ) ;
#81207=AXIS2_PLACEMENT_3D ( 'NONE', #24752, #72024, #86103 ) ;
#81211=VERTEX_POINT ( 'NONE', #58891 ) ;
#81268=DIRECTION ( 'NONE',  ( 0.5000000000000015543, -0.8660254037844377084, 2.688821387764056676E-14 ) ) ;
#81286=CARTESIAN_POINT ( 'NONE',  ( 146.0667039024470171, -83.77844715994089597, 55.21780685541800437 ) ) ;
#81292=CARTESIAN_POINT ( 'NONE',  ( 110.9303245704231102, -101.4704344580498514, -19.78219314458209865 ) ) ;
#81294=ORIENTED_EDGE ( 'NONE', *, *, #46236, .F. ) ;
#81333=CARTESIAN_POINT ( 'NONE',  ( 147.0667039024471592, -67.87844715994090450, 245.4990136654952835 ) ) ;
#81346=DIRECTION ( 'NONE',  ( -3.100000000000000258E-29, 3.100000000000000044E-14, 1.000000000000000000 ) ) ;
#81381=VERTEX_POINT ( 'NONE', #51088 ) ;
#81401=EDGE_CURVE ( 'NONE', #69984, #1742, #14357, .T. ) ;
#81415=CARTESIAN_POINT ( 'NONE',  ( 135.5667039024470171, -90.27844715994091018, 45.21780685541799727 ) ) ;
#81416=CYLINDRICAL_SURFACE ( 'NONE', #83357, 4.500000000000003553 ) ;
#81422=CARTESIAN_POINT ( 'NONE',  ( 146.6554688966711808, -67.87104837875700980, 246.9811635433789831 ) ) ;
#81427=DIRECTION ( 'NONE',  ( -1.000000000000000078E-15, 1.000000000000000000, 0.000000000000000000 ) ) ;
#81441=DIRECTION ( 'NONE',  ( -3.100000000000000258E-29, 3.100000000000000044E-14, 1.000000000000000000 ) ) ;
#81454=LINE ( 'NONE', #81005, #44621 ) ;
#81455=FACE_OUTER_BOUND ( 'NONE', #12148, .T. ) ;
#81460=EDGE_LOOP ( 'NONE', ( #34444, #67997, #26138, #24775 ) ) ;
#81464=DIRECTION ( 'NONE',  ( -1.000000000000000000, -1.734723475976808672E-15, 0.000000000000000000 ) ) ;
#81483=DIRECTION ( 'NONE',  ( 0.7071067811865496822, -0.7071067811865453523, 0.000000000000000000 ) ) ;
#81487=ORIENTED_EDGE ( 'NONE', *, *, #65864, .T. ) ;
#81489=VERTEX_POINT ( 'NONE', #66049 ) ;
#81496=EDGE_CURVE ( 'NONE', #15404, #81489, #5038, .T. ) ;
#81535=DIRECTION ( 'NONE',  ( 1.000000000000000000, 1.000000000000000078E-15, 0.000000000000000000 ) ) ;
#81542=AXIS2_PLACEMENT_3D ( 'NONE', #81286, #26293, #75795 ) ;
#81551=DIRECTION ( 'NONE',  ( 1.000000000000000000, 0.000000000000000000, 0.000000000000000000 ) ) ;
#81564=DIRECTION ( 'NONE',  ( 3.100000000000000258E-29, -3.100000000000000044E-14, -1.000000000000000000 ) ) ;
#81567=CARTESIAN_POINT ( 'NONE',  ( 67.06770054697865646, -67.87853365652237869, 245.5343369445640462 ) ) ;
#81577=AXIS2_PLACEMENT_3D ( 'NONE', #67027, #18425, #51597 ) ;
#81616=ORIENTED_EDGE ( 'NONE', *, *, #68486, .T. ) ;
#81644=DIRECTION ( 'NONE',  ( -1.000000000000000000, 0.000000000000000000, 0.000000000000000000 ) ) ;
#81647=ORIENTED_EDGE ( 'NONE', *, *, #33623, .T. ) ;
#81650=LINE ( 'NONE', #6227, #8842 ) ;
#81652=CARTESIAN_POINT ( 'NONE',  ( 121.3140869715381456, -113.5527167097541508, -11.78219314458173272 ) ) ;
#81653=CARTESIAN_POINT ( 'NONE',  ( 145.4069151017104105, -139.2712999699453462, 246.0952024083894401 ) ) ;
#81654=PLANE ( 'NONE',  #70005 ) ;
#81672=ORIENTED_EDGE ( 'NONE', *, *, #46236, .T. ) ;
#81678=DIRECTION ( 'NONE',  ( 0.9217329428042198014, 0.3878251953515564066, -1.214306433183767175E-14 ) ) ;
#81680=ORIENTED_EDGE ( 'NONE', *, *, #53750, .T. ) ;
#81682=CARTESIAN_POINT ( 'NONE',  ( 107.0667039024470313, -104.2784471599409528, 24.21780685541800082 ) ) ;
#81686=ORIENTED_EDGE ( 'NONE', *, *, #31763, .T. ) ;
#81691=CARTESIAN_POINT ( 'NONE',  ( 144.0667039024470455, -124.7784471599409102, 222.2178068554179902 ) ) ;
#81699=VERTEX_POINT ( 'NONE', #20608 ) ;
#81702=FACE_OUTER_BOUND ( 'NONE', #63547, .T. ) ;
#81703=ORIENTED_EDGE ( 'NONE', *, *, #22866, .F. ) ;
#81733=DIRECTION ( 'NONE',  ( -1.000000000000000000, -1.206764157201257538E-15, 0.000000000000000000 ) ) ;
#81745=DIRECTION ( 'NONE',  ( -1.000000000000000078E-15, 1.000000000000000000, 0.000000000000000000 ) ) ;
#81755=DIRECTION ( 'NONE',  ( 0.5000000000000012212, -0.8660254037844379305, 2.684678751731759347E-14 ) ) ;
#81793=DIRECTION ( 'NONE',  ( -3.100000000000000258E-29, 3.100000000000000044E-14, 1.000000000000000000 ) ) ;
#81833=ORIENTED_EDGE ( 'NONE', *, *, #79631, .F. ) ;
#81834=EDGE_CURVE ( 'NONE', #29924, #21942, #81957, .T. ) ;
#81840=CARTESIAN_POINT ( 'NONE',  ( 107.0667039024470313, -104.2784471599413934, 2.217806855418003043 ) ) ;
#81851=CYLINDRICAL_SURFACE ( 'NONE', #70379, 4.000000000000002665 ) ;
#81862=CARTESIAN_POINT ( 'NONE',  ( 145.4416927396864878, -139.3034583227001804, 245.6607614918409865 ) ) ;
#81876=LINE ( 'NONE', #19189, #27517 ) ;
#81895=CARTESIAN_POINT ( 'NONE',  ( 125.5177273812784762, -131.0330679306342461, 222.2178068554179902 ) ) ;
#81903=FACE_OUTER_BOUND ( 'NONE', #60660, .T. ) ;
#81905=LINE ( 'NONE', #38751, #51145 ) ;
#81907=AXIS2_PLACEMENT_3D ( 'NONE', #74018, #39497, #38597 ) ;
#81957=CIRCLE ( 'NONE', #29755, 2.999999999999988898 ) ;
#81963=CARTESIAN_POINT ( 'NONE',  ( 131.5667039024470455, -104.2784471599409244, 22.21780685541800082 ) ) ;
#81972=DIRECTION ( 'NONE',  ( 1.000000000000000000, 0.000000000000000000, 0.000000000000000000 ) ) ;
#81976=DIRECTION ( 'NONE',  ( 0.000000000000000000, 0.000000000000000000, 1.000000000000000000 ) ) ;
#81988=CARTESIAN_POINT ( 'NONE',  ( 71.06670390244705970, -124.7784471599409812, 45.21780685541799727 ) ) ;
#81989=DIRECTION ( 'NONE',  ( 3.100000000000000258E-29, -3.100000000000000044E-14, -1.000000000000000000 ) ) ;
#82002=LINE ( 'NONE', #89257, #45039 ) ;
#82003=EDGE_CURVE ( 'NONE', #82155, #38959, #42815, .T. ) ;
#82022=AXIS2_PLACEMENT_3D ( 'NONE', #55102, #21065, #35574 ) ;
#82027=ORIENTED_EDGE ( 'NONE', *, *, #68548, .T. ) ;
#82029=CARTESIAN_POINT ( 'NONE',  ( 144.1785682890445628, -138.0502943055581966, 247.6584922886219999 ) ) ;
#82035=DIRECTION ( 'NONE',  ( 3.100000000000000258E-29, -3.100000000000000044E-14, -1.000000000000000000 ) ) ;
#82049=LINE ( 'NONE', #27066, #62678 ) ;
#82055=ORIENTED_EDGE ( 'NONE', *, *, #40112, .F. ) ;
#82057=FACE_OUTER_BOUND ( 'NONE', #29327, .T. ) ;
#82088=LINE ( 'NONE', #18481, #25883 ) ;
#82091=CARTESIAN_POINT ( 'NONE',  ( 114.6444261855608175, -117.4034471599418055, -11.78219314458159239 ) ) ;
#82095=ORIENTED_EDGE ( 'NONE', *, *, #63457, .F. ) ;
#82103=CARTESIAN_POINT ( 'NONE',  ( 144.0731096511982798, -140.3870298840350017, 246.8745206071880034 ) ) ;
#82116=EDGE_CURVE ( 'NONE', #56525, #31932, #2263, .T. ) ;
#82134=EDGE_CURVE ( 'NONE', #4517, #27286, #19618, .T. ) ;
#82147=FACE_OUTER_BOUND ( 'NONE', #77899, .T. ) ;
#82151=ORIENTED_EDGE ( 'NONE', *, *, #4803, .F. ) ;
#82155=VERTEX_POINT ( 'NONE', #28307 ) ;
#82168=DIRECTION ( 'NONE',  ( 0.000000000000000000, 0.000000000000000000, 1.000000000000000000 ) ) ;
#82218=FACE_OUTER_BOUND ( 'NONE', #59829, .T. ) ;
#82224=CARTESIAN_POINT ( 'NONE',  ( 69.95046282694566742, -138.0544793580991723, 247.6577929086349741 ) ) ;
#82227=PLANE ( 'NONE',  #24017 ) ;
#82249=CARTESIAN_POINT ( 'NONE',  ( 91.91125933621934507, -111.8737466215629013, -21.78219314458179667 ) ) ;
#82254=AXIS2_PLACEMENT_3D ( 'NONE', #77826, #23326, #43729 ) ;
#82256=VECTOR ( 'NONE', #20113, 1000.000000000000000 ) ;
#82261=VERTEX_POINT ( 'NONE', #22871 ) ;
#82271=AXIS2_PLACEMENT_3D ( 'NONE', #79325, #44774, #72498 ) ;
#82281=CARTESIAN_POINT ( 'NONE',  ( 59.56670390244699576, -67.87844715994098976, 155.2178068554179902 ) ) ;
#82299=ORIENTED_EDGE ( 'NONE', *, *, #77567, .T. ) ;
#82314=AXIS2_PLACEMENT_3D ( 'NONE', #53948, #21255, #62580 ) ;
#82330=LINE ( 'NONE', #20092, #55759 ) ;
#82344=EDGE_CURVE ( 'NONE', #80812, #86777, #79179, .T. ) ;
#82351=ORIENTED_EDGE ( 'NONE', *, *, #28038, .F. ) ;
#82359=VERTEX_POINT ( 'NONE', #57360 ) ;
#82383=VECTOR ( 'NONE', #69824, 1000.000000000000000 ) ;
#82398=VERTEX_POINT ( 'NONE', #32326 ) ;
#82399=EDGE_CURVE ( 'NONE', #82603, #17863, #60026, .T. ) ;
#82427=CARTESIAN_POINT ( 'NONE',  ( 120.2221484686747317, -111.8737466215628871, -21.78219314458179667 ) ) ;
#82447=ORIENTED_EDGE ( 'NONE', *, *, #16301, .T. ) ;
#82466=ADVANCED_FACE ( 'NONE', ( #73678 ), #45839, .F. ) ;
#82470=ADVANCED_FACE ( 'NONE', ( #74134, #5089 ), #87315, .T. ) ;
#82471=AXIS2_PLACEMENT_3D ( 'NONE', #64852, #69880, #43942 ) ;
#82474=CARTESIAN_POINT ( 'NONE',  ( 122.2189888861420286, -96.57077177933004464, -19.18411693322927292 ) ) ;
#82476=ORIENTED_EDGE ( 'NONE', *, *, #31763, .F. ) ;
#82481=VERTEX_POINT ( 'NONE', #34125 ) ;
#82483=CARTESIAN_POINT ( 'NONE',  ( 107.0667039024470313, -104.2784471599421323, -21.78219314458201694 ) ) ;
#82507=DIRECTION ( 'NONE',  ( 1.000000000000000078E-15, -1.000000000000000000, 0.000000000000000000 ) ) ;
#82521=CARTESIAN_POINT ( 'NONE',  ( 154.5667039024469886, -67.87844715994090450, 190.2178068554179902 ) ) ;
#82528=VECTOR ( 'NONE', #52336, 1000.000000000000000 ) ;
#82533=ADVANCED_FACE ( 'NONE', ( #34578 ), #28664, .T. ) ;
#82544=CARTESIAN_POINT ( 'NONE',  ( 107.0667039024470313, -104.2784471599418197, -11.78219314458200984 ) ) ;
#82561=ORIENTED_EDGE ( 'NONE', *, *, #86345, .T. ) ;
#82589=CARTESIAN_POINT ( 'NONE',  ( 145.2166182285888851, -69.56242951228074389, 247.5001056298889921 ) ) ;
#82600=ORIENTED_EDGE ( 'NONE', *, *, #21249, .F. ) ;
#82603=VERTEX_POINT ( 'NONE', #27318 ) ;
#82619=FACE_OUTER_BOUND ( 'NONE', #85607, .T. ) ;
#82621=LINE ( 'NONE', #6293, #71062 ) ;
#82634=CARTESIAN_POINT ( 'NONE',  ( 107.0667039024470313, -104.2784471599409528, 250.2178068554179902 ) ) ;
#82667=CARTESIAN_POINT ( 'NONE',  ( 115.0667039024470313, -104.2784471599420897, -21.78219314458201694 ) ) ;
#82697=CARTESIAN_POINT ( 'NONE',  ( 122.2221484686747601, -109.6038751290258944, -21.02845593540793345 ) ) ;
#82700=CARTESIAN_POINT ( 'NONE',  ( 140.0667039024470171, -90.27844715994091018, 45.21780685541799727 ) ) ;
#82721=CIRCLE ( 'NONE', #78381, 3.000000864267354572 ) ;
#82733=AXIS2_PLACEMENT_3D ( 'NONE', #1172, #85645, #16588 ) ;
#82738=ADVANCED_FACE ( 'NONE', ( #30464 ), #43174, .F. ) ;
#82751=ADVANCED_FACE ( 'NONE', ( #17286 ), #22769, .F. ) ;
#82770=FACE_OUTER_BOUND ( 'NONE', #73278, .T. ) ;
#82774=CARTESIAN_POINT ( 'NONE',  ( 107.0667039024470313, -104.2784471599409528, 24.21780685541800082 ) ) ;
#82781=CARTESIAN_POINT ( 'NONE',  ( 67.06670390123206005, -137.6784471587259873, 245.4218662566639750 ) ) ;
#82795=CYLINDRICAL_SURFACE ( 'NONE', #73474, 4.500000000000003553 ) ;
#82796=AXIS2_PLACEMENT_3D ( 'NONE', #82427, #32445, #32903 ) ;
#82828=ORIENTED_EDGE ( 'NONE', *, *, #44334, .T. ) ;
#82858=ADVANCED_FACE ( 'NONE', ( #86771 ), #4089, .F. ) ;
#82865=ORIENTED_EDGE ( 'NONE', *, *, #1851, .F. ) ;
#82894=ORIENTED_EDGE ( 'NONE', *, *, #70412, .F. ) ;
#82899=CARTESIAN_POINT ( 'NONE',  ( 162.0667039024470171, -79.67844715994088745, 222.2178068554179902 ) ) ;
#82903=CARTESIAN_POINT ( 'NONE',  ( 67.62649790207950673, -68.41612585961607351, 246.8806801031981877 ) ) ;
#82926=ORIENTED_EDGE ( 'NONE', *, *, #7652, .F. ) ;
#82935=ORIENTED_EDGE ( 'NONE', *, *, #40224, .T. ) ;
#82943=CARTESIAN_POINT ( 'NONE',  ( 107.0667039024470313, -104.2784471599409528, 25.71780685541800437 ) ) ;
#82954=CIRCLE ( 'NONE', #25091, 4.000000000000002665 ) ;
#82963=DIRECTION ( 'NONE',  ( 1.000000000000000000, 0.000000000000000000, 0.000000000000000000 ) ) ;
#82967=ADVANCED_FACE ( 'NONE', ( #59928 ), #19062, .F. ) ;
#82971=CIRCLE ( 'NONE', #55359, 3.500000000000003109 ) ;
#82975=EDGE_LOOP ( 'NONE', ( #33639, #27218, #59344, #17436, #59362 ) ) ;
#82986=DIRECTION ( 'NONE',  ( 1.000000000000000078E-15, -1.000000000000000000, 0.000000000000000000 ) ) ;
#82994=CARTESIAN_POINT ( 'NONE',  ( 145.3961078426698066, -139.2608187703180249, 246.1574457750005251 ) ) ;
#82997=AXIS2_PLACEMENT_3D ( 'NONE', #58578, #51760, #44951 ) ;
#83005=CYLINDRICAL_SURFACE ( 'NONE', #23781, 2.000000000000001776 ) ;
#83018=CIRCLE ( 'NONE', #16290, 3.000000000000002665 ) ;
#83023=VECTOR ( 'NONE', #50201, 1000.000000000000000 ) ;
#83031=ORIENTED_EDGE ( 'NONE', *, *, #62807, .T. ) ;
#83038=CARTESIAN_POINT ( 'NONE',  ( 90.06670420047028358, -137.6784471599409585, 55.21780685541800437 ) ) ;
#83061=AXIS2_PLACEMENT_3D ( 'NONE', #31606, #80673, #37984 ) ;
#83063=CARTESIAN_POINT ( 'NONE',  ( 122.2221484686747317, -101.0284471599423171, -21.78219314458213063 ) ) ;
#83069=DIRECTION ( 'NONE',  ( 3.100000000000000258E-29, -3.100000000000000044E-14, -1.000000000000000000 ) ) ;
#83084=DIRECTION ( 'NONE',  ( 7.076552332833900719E-16, -1.000000000000000000, 3.100000000000000044E-14 ) ) ;
#83100=FACE_OUTER_BOUND ( 'NONE', #20835, .T. ) ;
#83101=PLANE ( 'NONE',  #48548 ) ;
#83114=DIRECTION ( 'NONE',  ( -0.8660254037844380415, -0.5000000000000012212, 1.550000000000001284E-14 ) ) ;
#83127=ORIENTED_EDGE ( 'NONE', *, *, #80377, .F. ) ;
#83146=AXIS2_PLACEMENT_3D ( 'NONE', #63048, #78046, #14470 ) ;
#83150=DIRECTION ( 'NONE',  ( -3.100000000000000258E-29, 3.100000000000000044E-14, 1.000000000000000000 ) ) ;
#83152=ORIENTED_EDGE ( 'NONE', *, *, #81834, .F. ) ;
#83155=EDGE_CURVE ( 'NONE', #1627, #61361, #59272, .T. ) ;
#83185=CARTESIAN_POINT ( 'NONE',  ( 151.0667039024469886, -67.87844715994090450, 155.2178068554179902 ) ) ;
#83198=CARTESIAN_POINT ( 'NONE',  ( 107.0667039024470313, -104.2784471599409528, 19.21780685541800437 ) ) ;
#83209=CARTESIAN_POINT ( 'NONE',  ( 139.3670970868850532, -133.7001840312377396, 248.3919668373590071 ) ) ;
#83216=CARTESIAN_POINT ( 'NONE',  ( 105.1589286322272585, -76.77844715994095282, 250.2178068554180470 ) ) ;
#83218=CARTESIAN_POINT ( 'NONE',  ( 67.77264411201586825, -137.9410731809939819, 246.8967413324789959 ) ) ;
#83222=VERTEX_POINT ( 'NONE', #24763 ) ;
#83227=AXIS2_PLACEMENT_3D ( 'NONE', #51667, #64877, #78967 ) ;
#83229=EDGE_CURVE ( 'NONE', #60182, #78082, #10244, .T. ) ;
#83230=EDGE_CURVE ( 'NONE', #75851, #82261, #47291, .T. ) ;
#83242=CARTESIAN_POINT ( 'NONE',  ( 56.06670390244699576, -67.87844715994098976, 155.2178068554179902 ) ) ;
#83247=CYLINDRICAL_SURFACE ( 'NONE', #18043, 1.999999999999995781 ) ;
#83258=LINE ( 'NONE', #35081, #87039 ) ;
#83281=AXIS2_PLACEMENT_3D ( 'NONE', #8279, #1013, #29168 ) ;
#83285=VECTOR ( 'NONE', #53494, 1000.000000000000000 ) ;
#83305=CARTESIAN_POINT ( 'NONE',  ( 107.0667039024470313, -104.2784471599420755, -19.78219314458201694 ) ) ;
#83319=CARTESIAN_POINT ( 'NONE',  ( 70.57087804374656059, -139.4754646311776867, 247.4327973477450087 ) ) ;
#83328=CARTESIAN_POINT ( 'NONE',  ( 133.3245970085671388, -112.6232539059702731, 250.2178068554180470 ) ) ;
#83330=CARTESIAN_POINT ( 'NONE',  ( 70.88111044991026688, -139.0101909505960691, 247.5112285516309782 ) ) ;
#83338=CARTESIAN_POINT ( 'NONE',  ( 95.56670390244703128, -104.2784471599408818, 19.21780685541799016 ) ) ;
#83346=CARTESIAN_POINT ( 'NONE',  ( 145.5337519030156557, -69.32260879017363209, 247.4441250540085946 ) ) ;
#83357=AXIS2_PLACEMENT_3D ( 'NONE', #11452, #39147, #54094 ) ;
#83391=B_SPLINE_CURVE_WITH_KNOTS ( 'NONE', 3,
 ( #64794, #86585, #37975, #50707, #3901, #17968, #31599, #37542, #58849, #29835, #59299, #52465, #58412, #16209, #9384, #24357, #37093, #30717 ),
 .UNSPECIFIED., .F., .F.,
 ( 4, 2, 2, 2, 2, 2, 2, 2, 4 ),
 ( 0.000000000000000000, 0.1250000000000000000, 0.2500000000000000000, 0.3750000000000000000, 0.5000000000000000000, 0.6250000000000000000, 0.7500000000000000000, 0.8750000000000000000, 1.000000000000000000 ),
 .UNSPECIFIED. ) ;
#83400=ORIENTED_EDGE ( 'NONE', *, *, #68567, .T. ) ;
#83404=CARTESIAN_POINT ( 'NONE',  ( 147.0667039024470739, -137.6624395622106078, 245.7309020619233593 ) ) ;
#83406=ORIENTED_EDGE ( 'NONE', *, *, #31602, .T. ) ;
#83428=ADVANCED_FACE ( 'NONE', ( #54671 ), #41062, .F. ) ;
#83430=AXIS2_PLACEMENT_3D ( 'NONE', #12033, #32454, #19738 ) ;
#83435=DIRECTION ( 'NONE',  ( -0.7396053187813123042, -0.6730408400909958511, 0.000000000000000000 ) ) ;
#83446=CYLINDRICAL_SURFACE ( 'NONE', #85051, 4.000000000000006217 ) ;
#83522=EDGE_CURVE ( 'NONE', #54219, #81211, #75168, .T. ) ;
#83523=ORIENTED_EDGE ( 'NONE', *, *, #66494, .T. ) ;
#83526=ADVANCED_FACE ( 'NONE', ( #77388 ), #56931, .T. ) ;
#83558=ORIENTED_EDGE ( 'NONE', *, *, #35842, .F. ) ;
#83564=AXIS2_PLACEMENT_3D ( 'NONE', #83198, #35466, #62282 ) ;
#83582=EDGE_CURVE ( 'NONE', #1742, #8767, #71485, .T. ) ;
#83583=CARTESIAN_POINT ( 'NONE',  ( 107.0667039024470313, -104.2784471599418197, -11.78219314458200984 ) ) ;
#83588=EDGE_LOOP ( 'NONE', ( #57776, #84517, #65063, #88362 ) ) ;
#83620=ORIENTED_EDGE ( 'NONE', *, *, #82399, .T. ) ;
#83624=ORIENTED_EDGE ( 'NONE', *, *, #68372, .T. ) ;
#83625=CYLINDRICAL_SURFACE ( 'NONE', #33156, 4.500000000000003553 ) ;
#83629=CARTESIAN_POINT ( 'NONE',  ( 67.35034461891076774, -127.7125575906254937, 246.8833065113800274 ) ) ;
#83636=DIRECTION ( 'NONE',  ( 0.7071067811865453523, 0.7071067811865496822, 0.000000000000000000 ) ) ;
#83651=LINE ( 'NONE', #63646, #21974 ) ;
#83707=VERTEX_POINT ( 'NONE', #46412 ) ;
#83710=ORIENTED_EDGE ( 'NONE', *, *, #14096, .T. ) ;
#83712=DIRECTION ( 'NONE',  ( -1.000000000000000000, 0.000000000000000000, 0.000000000000000000 ) ) ;
#83713=CARTESIAN_POINT ( 'NONE',  ( 92.81551872686563343, -113.5468731908974291, -21.78219314458173983 ) ) ;
#83721=CARTESIAN_POINT ( 'NONE',  ( 59.56670390244700997, -79.67844715994098692, 155.2178068554179902 ) ) ;
#83724=CARTESIAN_POINT ( 'NONE',  ( 70.86177220334050730, -139.0548940191880263, 247.5038799219895225 ) ) ;
#83728=CIRCLE ( 'NONE', #25753, 7.999999999999992895 ) ;
#83735=CARTESIAN_POINT ( 'NONE',  ( 107.0667039024470313, -104.2784471599418197, -11.78219314458200984 ) ) ;
#83747=VECTOR ( 'NONE', #76681, 1000.000000000000000 ) ;
#83751=CARTESIAN_POINT ( 'NONE',  ( 110.8821949118858612, -131.5792096921222196, 250.2178068554180470 ) ) ;
#83756=LINE ( 'NONE', #36039, #78007 ) ;
#83759=DIRECTION ( 'NONE',  ( -3.100000000000000258E-29, 3.100000000000000044E-14, 1.000000000000000000 ) ) ;
#83769=DIRECTION ( 'NONE',  ( -1.000000000000000078E-15, 1.000000000000000000, 0.000000000000000000 ) ) ;
#83775=DIRECTION ( 'NONE',  ( 0.000000000000000000, 0.000000000000000000, 1.000000000000000000 ) ) ;
#83784=CARTESIAN_POINT ( 'NONE',  ( 134.4101120871804653, -100.8945472140119080, 250.2178068554180470 ) ) ;
#83791=CARTESIAN_POINT ( 'NONE',  ( 67.08338700029372603, -67.89281568731828997, 245.7496557518025782 ) ) ;
#83797=CARTESIAN_POINT ( 'NONE',  ( 117.0667039024470313, -98.59953881414097054, 7.717806855417813416 ) ) ;
#83810=AXIS2_PLACEMENT_3D ( 'NONE', #70722, #63907, #50249 ) ;
#83812=ORIENTED_EDGE ( 'NONE', *, *, #88767, .F. ) ;
#83828=EDGE_LOOP ( 'NONE', ( #40694, #64988, #61867, #63722, #5377, #82476 ) ) ;
#83853=FACE_BOUND ( 'NONE', #17469, .T. ) ;
#83858=EDGE_CURVE ( 'NONE', #23110, #45687, #45720, .T. ) ;
#83860=EDGE_CURVE ( 'NONE', #61847, #79697, #61836, .T. ) ;
#83862=CARTESIAN_POINT ( 'NONE',  ( 92.91125933621934507, -113.6057974291316981, -19.26696060647573105 ) ) ;
#83865=EDGE_CURVE ( 'NONE', #29557, #26687, #41319, .T. ) ;
#83871=CARTESIAN_POINT ( 'NONE',  ( 107.0667039024470313, -104.2784471599409528, 24.21780685541800082 ) ) ;
#83876=DIRECTION ( 'NONE',  ( 0.8660254037844392627, -0.4999999999999990008, 1.549999999999999706E-14 ) ) ;
#83878=DIRECTION ( 'NONE',  ( 0.000000000000000000, 0.000000000000000000, 1.000000000000000000 ) ) ;
#83881=ORIENTED_EDGE ( 'NONE', *, *, #52958, .F. ) ;
#83893=VECTOR ( 'NONE', #37714, 1000.000000000000000 ) ;
#83896=VERTEX_POINT ( 'NONE', #975 ) ;
#83911=FACE_OUTER_BOUND ( 'NONE', #73628, .T. ) ;
#83917=EDGE_CURVE ( 'NONE', #27883, #9196, #49549, .T. ) ;
#83918=CARTESIAN_POINT ( 'NONE',  ( 107.0667039024470313, -104.2784471599413791, 2.217806855418003043 ) ) ;
#83938=CARTESIAN_POINT ( 'NONE',  ( 86.72755763596092038, -85.76982405743865456, 250.2178068554179902 ) ) ;
#83949=AXIS2_PLACEMENT_3D ( 'NONE', #77593, #70784, #835 ) ;
#83965=PLANE ( 'NONE',  #83146 ) ;
#83968=EDGE_CURVE ( 'NONE', #34789, #62435, #11377, .T. ) ;
#83989=EDGE_CURVE ( 'NONE', #49274, #66921, #6588, .T. ) ;
#84002=VECTOR ( 'NONE', #3266, 1000.000000000000000 ) ;
#84010=ORIENTED_EDGE ( 'NONE', *, *, #32673, .T. ) ;
#84016=FACE_OUTER_BOUND ( 'NONE', #62069, .T. ) ;
#84036=CARTESIAN_POINT ( 'NONE',  ( 151.0667039024469886, -67.87844715994090450, 85.21780685541799016 ) ) ;
#84044=ORIENTED_EDGE ( 'NONE', *, *, #26302, .F. ) ;
#84060=ORIENTED_EDGE ( 'NONE', *, *, #42027, .T. ) ;
#84087=EDGE_LOOP ( 'NONE', ( #34189, #75987, #39182, #62265 ) ) ;
#84102=CARTESIAN_POINT ( 'NONE',  ( 110.7536356736639078, -102.7271463785351528, 2.217806855417947531 ) ) ;
#84110=ORIENTED_EDGE ( 'NONE', *, *, #26882, .T. ) ;
#84114=CARTESIAN_POINT ( 'NONE',  ( 88.01156830653434326, -84.35882332054471533, 250.2178068554179902 ) ) ;
#84116=VECTOR ( 'NONE', #66072, 1000.000000000000000 ) ;
#84117=DIRECTION ( 'NONE',  ( -1.000000000000000078E-15, 1.000000000000000000, 0.000000000000000000 ) ) ;
#84152=EDGE_CURVE ( 'NONE', #82481, #86394, #17296, .T. ) ;
#84165=ORIENTED_EDGE ( 'NONE', *, *, #78726, .F. ) ;
#84173=DIRECTION ( 'NONE',  ( 3.100000000000000258E-29, -3.100000000000000044E-14, -1.000000000000000000 ) ) ;
#84184=CARTESIAN_POINT ( 'NONE',  ( 146.0667039024470171, -86.77844715994089597, 55.21780685541800437 ) ) ;
#84185=CARTESIAN_POINT ( 'NONE',  ( 70.40000325710290952, -140.0960478153407109, 246.9444450209567776 ) ) ;
#84209=CARTESIAN_POINT ( 'NONE',  ( 121.5948191693372138, -127.7054288962554409, 250.2178068554180470 ) ) ;
#84222=VECTOR ( 'NONE', #81483, 1000.000000000000000 ) ;
#84240=CARTESIAN_POINT ( 'NONE',  ( 133.7890526427665066, -97.56809487397632097, 250.2178068554180470 ) ) ;
#84242=DIRECTION ( 'NONE',  ( 3.100000000000000258E-29, -3.100000000000000044E-14, -1.000000000000000000 ) ) ;
#84244=LINE ( 'NONE', #22015, #20505 ) ;
#84266=ORIENTED_EDGE ( 'NONE', *, *, #87139, .T. ) ;
#84271=ORIENTED_EDGE ( 'NONE', *, *, #31635, .F. ) ;
#84280=EDGE_LOOP ( 'NONE', ( #85444, #1361, #41716, #48894, #21554 ) ) ;
#84281=VERTEX_POINT ( 'NONE', #87228 ) ;
#84295=VECTOR ( 'NONE', #83876, 1000.000000000000000 ) ;
#84330=FACE_OUTER_BOUND ( 'NONE', #41011, .T. ) ;
#84334=ORIENTED_EDGE ( 'NONE', *, *, #54319, .F. ) ;
#84343=DIRECTION ( 'NONE',  ( 3.100000000000000258E-29, -3.100000000000000044E-14, -1.000000000000000000 ) ) ;
#84361=VECTOR ( 'NONE', #15507, 1000.000000000000000 ) ;
#84366=CARTESIAN_POINT ( 'NONE',  ( 130.5667039024470455, -104.2784471599409386, 23.21780685541800082 ) ) ;
#84388=VERTEX_POINT ( 'NONE', #82667 ) ;
#84389=EDGE_LOOP ( 'NONE', ( #76644, #21552, #86250, #45254, #46803, #2691, #51445, #23740, #81680, #75569, #56976, #80020, #16582, #50465, #46975, #3391, #7594, #32704, #36109, #72680, #21475, #13624, #36456, #68264 ) ) ;
#84400=AXIS2_PLACEMENT_3D ( 'NONE', #74785, #88428, #12565 ) ;
#84425=DIRECTION ( 'NONE',  ( -1.000000000000000078E-15, 1.000000000000000000, 0.000000000000000000 ) ) ;
#84431=CARTESIAN_POINT ( 'NONE',  ( 140.0667039024470455, -118.2784471599408960, 51.21780685541800437 ) ) ;
#84433=DIRECTION ( 'NONE',  ( -3.100000000000000258E-29, 3.100000000000000044E-14, 1.000000000000000000 ) ) ;
#84440=ORIENTED_EDGE ( 'NONE', *, *, #55593, .F. ) ;
#84453=ORIENTED_EDGE ( 'NONE', *, *, #23863, .T. ) ;
#84477=ADVANCED_FACE ( 'NONE', ( #26771 ), #42185, .T. ) ;
#84486=ADVANCED_FACE ( 'NONE', ( #82218 ), #77626, .T. ) ;
#84513=LINE ( 'NONE', #22270, #67879 ) ;
#84515=VECTOR ( 'NONE', #58739, 1000.000000000000000 ) ;
#84517=ORIENTED_EDGE ( 'NONE', *, *, #85700, .T. ) ;
#84518=CARTESIAN_POINT ( 'NONE',  ( 107.0667039024470313, -104.2784471599418197, -11.78219314458200984 ) ) ;
#84559=CYLINDRICAL_SURFACE ( 'NONE', #20471, 23.50000000000000711 ) ;
#84565=CARTESIAN_POINT ( 'NONE',  ( 164.0167039024470057, -75.72844715994088460, 222.2178068554179902 ) ) ;
#84582=EDGE_CURVE ( 'NONE', #86385, #47600, #72606, .T. ) ;
#84632=LINE ( 'NONE', #22392, #24583 ) ;
#84643=DIRECTION ( 'NONE',  ( 1.000000000000000000, 1.000000000000000078E-15, 0.000000000000000000 ) ) ;
#84646=FACE_OUTER_BOUND ( 'NONE', #43634, .T. ) ;
#84659=CARTESIAN_POINT ( 'NONE',  ( 107.0667039024470313, -104.2784471599413934, 2.217806855418003043 ) ) ;
#84662=ORIENTED_EDGE ( 'NONE', *, *, #76357, .T. ) ;
#84667=EDGE_CURVE ( 'NONE', #36009, #1539, #58808, .T. ) ;
#84675=CARTESIAN_POINT ( 'NONE',  ( 124.0667039024470313, -104.2784471599414360, 0.2178068554180012661 ) ) ;
#84678=CARTESIAN_POINT ( 'NONE',  ( 145.7671917778935438, -138.5331951669010948, 246.9855771338589818 ) ) ;
#84684=AXIS2_PLACEMENT_3D ( 'NONE', #44684, #3370, #71532 ) ;
#84687=CARTESIAN_POINT ( 'NONE',  ( 129.5675368918761876, -88.37796714256971597, 250.2178068554179902 ) ) ;
#84757=CARTESIAN_POINT ( 'NONE',  ( 107.0667039024470313, -104.2784471599413791, 2.217806855418003043 ) ) ;
#84761=DIRECTION ( 'NONE',  ( 0.000000000000000000, 0.000000000000000000, -1.000000000000000000 ) ) ;
#84777=LINE ( 'NONE', #12699, #9350 ) ;
#84793=ORIENTED_EDGE ( 'NONE', *, *, #25970, .F. ) ;
#84798=CARTESIAN_POINT ( 'NONE',  ( 107.0667039024470313, -104.2784471599409528, 249.2178068554179902 ) ) ;
#84803=CARTESIAN_POINT ( 'NONE',  ( 151.0667039024469886, -79.67844715994088745, 120.2178068554179902 ) ) ;
#84806=VECTOR ( 'NONE', #76045, 1000.000000000000000 ) ;
#84850=AXIS2_PLACEMENT_3D ( 'NONE', #10900, #10028, #59038 ) ;
#84863=VERTEX_POINT ( 'NONE', #26514 ) ;
#84877=DIRECTION ( 'NONE',  ( -0.8660254037844392627, 0.4999999999999990008, -1.549999999999999706E-14 ) ) ;
#84897=ORIENTED_EDGE ( 'NONE', *, *, #33244, .F. ) ;
#84923=ORIENTED_EDGE ( 'NONE', *, *, #12561, .T. ) ;
#84941=ORIENTED_EDGE ( 'NONE', *, *, #47635, .F. ) ;
#84943=ORIENTED_EDGE ( 'NONE', *, *, #63109, .F. ) ;
#84952=CARTESIAN_POINT ( 'NONE',  ( 144.5809607762889470, -138.4431012436764377, 247.5929369389089914 ) ) ;
#84955=FACE_BOUND ( 'NONE', #29132, .T. ) ;
#84959=VERTEX_POINT ( 'NONE', #74226 ) ;
#84960=ORIENTED_EDGE ( 'NONE', *, *, #6036, .T. ) ;
#84963=CARTESIAN_POINT ( 'NONE',  ( 70.06670390244705970, -124.7784471599409812, 55.21780685541800437 ) ) ;
#84979=ORIENTED_EDGE ( 'NONE', *, *, #26843, .F. ) ;
#84992=CARTESIAN_POINT ( 'NONE',  ( 107.0667039024470313, -104.2784471599421323, -21.78219314458201694 ) ) ;
#84997=CARTESIAN_POINT ( 'NONE',  ( 99.03451269431035087, -108.3384846469520255, 2.217806855418142042 ) ) ;
#85022=EDGE_LOOP ( 'NONE', ( #20019, #34915, #57499, #64516 ) ) ;
#85024=DIRECTION ( 'NONE',  ( -3.100000000000000258E-29, 3.100000000000000044E-14, 1.000000000000000000 ) ) ;
#85029=DIRECTION ( 'NONE',  ( 0.000000000000000000, 0.000000000000000000, 1.000000000000000000 ) ) ;
#85041=VECTOR ( 'NONE', #2707, 1000.000000000000000 ) ;
#85050=CARTESIAN_POINT ( 'NONE',  ( 107.0667039024470313, -104.2784471599418197, -11.78219314458200984 ) ) ;
#85051=AXIS2_PLACEMENT_3D ( 'NONE', #48438, #14414, #88921 ) ;
#85054=ORIENTED_EDGE ( 'NONE', *, *, #38865, .T. ) ;
#85092=CARTESIAN_POINT ( 'NONE',  ( 130.5667039024470455, -104.2784471599409386, 23.21780685541800082 ) ) ;
#85096=LINE ( 'NONE', #29224, #74558 ) ;
#85102=VERTEX_POINT ( 'NONE', #32396 ) ;
#85103=LINE ( 'NONE', #48291, #75742 ) ;
#85107=VECTOR ( 'NONE', #69393, 1000.000000000000000 ) ;
#85131=VECTOR ( 'NONE', #32294, 1000.000000000000000 ) ;
#85157=CARTESIAN_POINT ( 'NONE',  ( 154.5667039024469886, -67.87844715994090450, 155.2178068554179902 ) ) ;
#85164=CARTESIAN_POINT ( 'NONE',  ( 52.06670390244699576, -67.87844715994100397, 222.2178068554179902 ) ) ;
#85165=CARTESIAN_POINT ( 'NONE',  ( 125.5177273812784193, -99.45575754528751133, 222.2178068554179902 ) ) ;
#85167=DIRECTION ( 'NONE',  ( -1.000000000000000000, 0.000000000000000000, 0.000000000000000000 ) ) ;
#85172=DIRECTION ( 'NONE',  ( -3.100000000000000258E-29, 3.100000000000000044E-14, 1.000000000000000000 ) ) ;
#85186=FACE_OUTER_BOUND ( 'NONE', #14592, .T. ) ;
#85189=CARTESIAN_POINT ( 'NONE',  ( 81.98010489515323229, -91.89993919647076837, 250.2190963482990185 ) ) ;
#85190=ORIENTED_EDGE ( 'NONE', *, *, #64249, .F. ) ;
#85211=FACE_OUTER_BOUND ( 'NONE', #55615, .T. ) ;
#85216=CARTESIAN_POINT ( 'NONE',  ( 146.2220825168437841, -137.2276697249587869, 247.1459391770515595 ) ) ;
#85224=CARTESIAN_POINT ( 'NONE',  ( 107.0667036193247696, -70.87844715994094713, 90.21780599115065513 ) ) ;
#85229=VERTEX_POINT ( 'NONE', #5161 ) ;
#85246=ORIENTED_EDGE ( 'NONE', *, *, #89868, .F. ) ;
#85250=APPLICATION_CONTEXT ( 'automotive_design' ) ;
#85277=CARTESIAN_POINT ( 'NONE',  ( 97.06670390244701707, -98.59953881414068633, 17.71780685541782319 ) ) ;
#85281=EDGE_LOOP ( 'NONE', ( #11640, #85856, #81647, #47445, #7511, #24760 ) ) ;
#85291=FACE_OUTER_BOUND ( 'NONE', #25649, .T. ) ;
#85320=CARTESIAN_POINT ( 'NONE',  ( 74.06670390244701707, -90.27844715994098124, 51.21780685541800437 ) ) ;
#85321=ORIENTED_EDGE ( 'NONE', *, *, #48140, .T. ) ;
#85336=ORIENTED_EDGE ( 'NONE', *, *, #59782, .F. ) ;
#85339=ORIENTED_EDGE ( 'NONE', *, *, #48140, .F. ) ;
#85348=CARTESIAN_POINT ( 'NONE',  ( 107.0667039024470313, -104.2784471599413934, 2.217806855418003043 ) ) ;
#85356=DIRECTION ( 'NONE',  ( -1.000000000000000000, 0.000000000000000000, 0.000000000000000000 ) ) ;
#85402=VECTOR ( 'NONE', #47149, 1000.000000000000000 ) ;
#85433=ORIENTED_EDGE ( 'NONE', *, *, #5030, .F. ) ;
#85443=DIRECTION ( 'NONE',  ( 3.100000000000000258E-29, -3.100000000000000044E-14, -1.000000000000000000 ) ) ;
#85444=ORIENTED_EDGE ( 'NONE', *, *, #27551, .F. ) ;
#85460=ORIENTED_EDGE ( 'NONE', *, *, #9319, .T. ) ;
#85467=FACE_OUTER_BOUND ( 'NONE', #23338, .T. ) ;
#85493=DIRECTION ( 'NONE',  ( -7.559289460184346452E-16, 0.7559289460184345222, -0.6546536707080001793 ) ) ;
#85506=AXIS2_PLACEMENT_3D ( 'NONE', #36446, #42329, #64150 ) ;
#85522=ORIENTED_EDGE ( 'NONE', *, *, #6776, .F. ) ;
#85530=CARTESIAN_POINT ( 'NONE',  ( 97.81670390244700286, -67.87844715994096134, 55.21780685541800437 ) ) ;
#85533=DIRECTION ( 'NONE',  ( -0.000000000000000000, -0.000000000000000000, -1.000000000000000000 ) ) ;
#85548=DIRECTION ( 'NONE',  ( 0.000000000000000000, 0.000000000000000000, -1.000000000000000000 ) ) ;
#85551=DIRECTION ( 'NONE',  ( -1.000000000000000000, 0.000000000000000000, 0.000000000000000000 ) ) ;
#85567=ORIENTED_EDGE ( 'NONE', *, *, #39819, .T. ) ;
#85575=CARTESIAN_POINT ( 'NONE',  ( 145.1732792321600698, -139.1256337189776389, 247.0684060528939767 ) ) ;
#85579=ORIENTED_EDGE ( 'NONE', *, *, #5802, .F. ) ;
#85582=EDGE_CURVE ( 'NONE', #1745, #79206, #45466, .T. ) ;
#85583=LINE ( 'NONE', #71936, #9486 ) ;
#85596=CARTESIAN_POINT ( 'NONE',  ( 131.1848578969771211, -79.26006987685342153, 249.3134381260879877 ) ) ;
#85606=ORIENTED_EDGE ( 'NONE', *, *, #49003, .T. ) ;
#85607=EDGE_LOOP ( 'NONE', ( #56932, #29696, #34604, #117 ) ) ;
#85616=DIRECTION ( 'NONE',  ( -0.000000000000000000, -0.000000000000000000, -1.000000000000000000 ) ) ;
#85639=ORIENTED_EDGE ( 'NONE', *, *, #8692, .F. ) ;
#85645=DIRECTION ( 'NONE',  ( 3.100000000000000258E-29, -3.100000000000000044E-14, -1.000000000000000000 ) ) ;
#85697=CARTESIAN_POINT ( 'NONE',  ( 67.06670390244678970, -67.87844716023829506, 245.4990141143767630 ) ) ;
#85700=EDGE_CURVE ( 'NONE', #11860, #36556, #5054, .T. ) ;
#85717=EDGE_CURVE ( 'NONE', #61024, #84863, #25699, .T. ) ;
#85719=DIRECTION ( 'NONE',  ( 1.000000000000000000, 1.000000000000000078E-15, -0.000000000000000000 ) ) ;
#85724=VERTEX_POINT ( 'NONE', #13221 ) ;
#85726=ORIENTED_EDGE ( 'NONE', *, *, #5922, .F. ) ;
#85756=CARTESIAN_POINT ( 'NONE',  ( 153.0667045879000057, -71.37844715994090450, 222.2178068554179902 ) ) ;
#85762=ORIENTED_EDGE ( 'NONE', *, *, #8070, .F. ) ;
#85766=CARTESIAN_POINT ( 'NONE',  ( 107.0667039024470313, -104.2784471599418197, -11.78219314458200984 ) ) ;
#85778=ORIENTED_EDGE ( 'NONE', *, *, #21302, .F. ) ;
#85795=EDGE_CURVE ( 'NONE', #51345, #70808, #86838, .T. ) ;
#85821=CARTESIAN_POINT ( 'NONE',  ( 106.5667039024470455, -113.7784471599420613, -19.78219314458171141 ) ) ;
#85827=CARTESIAN_POINT ( 'NONE',  ( 100.6318841171118805, -120.9585416479406206, -9.274842254010108533 ) ) ;
#85833=CARTESIAN_POINT ( 'NONE',  ( 124.0667039024470313, -104.2784471599417486, -9.937637710810031777 ) ) ;
#85856=ORIENTED_EDGE ( 'NONE', *, *, #6124, .T. ) ;
#85859=FACE_OUTER_BOUND ( 'NONE', #20063, .T. ) ;
#85888=AXIS2_PLACEMENT_3D ( 'NONE', #66621, #16701, #86637 ) ;
#85891=VECTOR ( 'NONE', #26524, 1000.000000000000000 ) ;
#85937=DIRECTION ( 'NONE',  ( -3.100000000000000258E-29, 3.100000000000000044E-14, 1.000000000000000000 ) ) ;
#85940=VERTEX_POINT ( 'NONE', #84963 ) ;
#85952=FACE_BOUND ( 'NONE', #17522, .T. ) ;
#85962=FACE_OUTER_BOUND ( 'NONE', #27045, .T. ) ;
#85972=CARTESIAN_POINT ( 'NONE',  ( 151.0667039024469886, -67.87844715994090450, 85.21780685541799016 ) ) ;
#85975=AXIS2_PLACEMENT_3D ( 'NONE', #65249, #57076, #8506 ) ;
#85983=FACE_OUTER_BOUND ( 'NONE', #86226, .T. ) ;
#85989=FACE_BOUND ( 'NONE', #30618, .T. ) ;
#85990=CIRCLE ( 'NONE', #40962, 3.499999999999996003 ) ;
#86014=DIRECTION ( 'NONE',  ( 0.000000000000000000, 0.000000000000000000, -1.000000000000000000 ) ) ;
#86016=CARTESIAN_POINT ( 'NONE',  ( 144.1741083578144753, -138.0461846875238905, 247.6591807063120143 ) ) ;
#86038=CARTESIAN_POINT ( 'NONE',  ( 112.5622543395261062, -68.63512909430427555, 247.5000682988239760 ) ) ;
#86048=ORIENTED_EDGE ( 'NONE', *, *, #44641, .T. ) ;
#86056=EDGE_CURVE ( 'NONE', #53380, #1337, #88106, .T. ) ;
#86061=AXIS2_PLACEMENT_3D ( 'NONE', #48494, #1286, #36248 ) ;
#86076=EDGE_LOOP ( 'NONE', ( #12977, #42109, #6224, #37837 ) ) ;
#86077=ADVANCED_FACE ( 'NONE', ( #52607 ), #24944, .F. ) ;
#86085=DIRECTION ( 'NONE',  ( -3.114895971316861016E-16, 1.000000000000000000, 0.000000000000000000 ) ) ;
#86086=FACE_OUTER_BOUND ( 'NONE', #37794, .T. ) ;
#86092=CARTESIAN_POINT ( 'NONE',  ( 67.28251452665169552, -137.5317448489894332, 246.4199739687819317 ) ) ;
#86096=VERTEX_POINT ( 'NONE', #59446 ) ;
#86103=DIRECTION ( 'NONE',  ( -1.000000000000000000, -8.163404592832032979E-16, 0.000000000000000000 ) ) ;
#86107=ORIENTED_EDGE ( 'NONE', *, *, #20787, .F. ) ;
#86126=EDGE_LOOP ( 'NONE', ( #4717, #37120, #56312, #21157, #79346 ) ) ;
#86129=VECTOR ( 'NONE', #61794, 1000.000000000000000 ) ;
#86134=FACE_OUTER_BOUND ( 'NONE', #6950, .T. ) ;
#86156=CARTESIAN_POINT ( 'NONE',  ( 143.5667039024469886, -67.87844715994090450, 55.21780685541800437 ) ) ;
#86158=EDGE_LOOP ( 'NONE', ( #83710, #57827 ) ) ;
#86168=LINE ( 'NONE', #3930, #61185 ) ;
#86175=CARTESIAN_POINT ( 'NONE',  ( 147.0667039024470171, -77.84948640091441519, 245.5415602474340062 ) ) ;
#86184=AXIS2_PLACEMENT_3D ( 'NONE', #39134, #52279, #88203 ) ;
#86185=CARTESIAN_POINT ( 'NONE',  ( 108.0345720930109081, -87.33724612030414391, -19.23816774842054755 ) ) ;
#86196=EDGE_CURVE ( 'NONE', #30286, #56525, #61242, .T. ) ;
#86205=FACE_OUTER_BOUND ( 'NONE', #63534, .T. ) ;
#86206=DIRECTION ( 'NONE',  ( 0.000000000000000000, 0.000000000000000000, -1.000000000000000000 ) ) ;
#86218=FACE_OUTER_BOUND ( 'NONE', #44958, .T. ) ;
#86219=ADVANCED_FACE ( 'NONE', ( #19467 ), #48478, .T. ) ;
#86226=EDGE_LOOP ( 'NONE', ( #66903, #69151, #30686, #7185 ) ) ;
#86244=LINE ( 'NONE', #58080, #24210 ) ;
#86250=ORIENTED_EDGE ( 'NONE', *, *, #8590, .F. ) ;
#86256=CARTESIAN_POINT ( 'NONE',  ( 67.06681409635508828, -67.87844715994098976, 245.5130139786259917 ) ) ;
#86260=DIRECTION ( 'NONE',  ( 0.5000000000000015543, -0.8660254037844377084, 2.602085213965216006E-14 ) ) ;
#86261=AXIS2_PLACEMENT_3D ( 'NONE', #56135, #48874, #69801 ) ;
#86271=DIRECTION ( 'NONE',  ( 1.000000000000000078E-15, -1.000000000000000000, 0.000000000000000000 ) ) ;
#86273=LINE ( 'NONE', #51720, #31842 ) ;
#86303=VERTEX_POINT ( 'NONE', #88964 ) ;
#86306=LINE ( 'NONE', #46728, #83893 ) ;
#86321=ORIENTED_EDGE ( 'NONE', *, *, #81401, .F. ) ;
#86331=AXIS2_PLACEMENT_3D ( 'NONE', #84798, #50239, #83435 ) ;
#86335=B_SPLINE_CURVE_WITH_KNOTS ( 'NONE', 3,
 ( #21828, #7736, #16346, #77233 ),
 .UNSPECIFIED., .F., .F.,
 ( 4, 4 ),
 ( -0.3974825557268080178, -0.3842043193313759986 ),
 .UNSPECIFIED. ) ;
#86337=VERTEX_POINT ( 'NONE', #54853 ) ;
#86345=EDGE_CURVE ( 'NONE', #31932, #33837, #31529, .T. ) ;
#86350=ORIENTED_EDGE ( 'NONE', *, *, #58210, .F. ) ;
#86359=LINE ( 'NONE', #72722, #936 ) ;
#86373=ORIENTED_EDGE ( 'NONE', *, *, #18657, .T. ) ;
#86385=VERTEX_POINT ( 'NONE', #78033 ) ;
#86389=AXIS2_PLACEMENT_3D ( 'NONE', #24561, #4108, #31807 ) ;
#86394=VERTEX_POINT ( 'NONE', #49395 ) ;
#86405=B_SPLINE_CURVE_WITH_KNOTS ( 'NONE', 3,
 ( #59686, #17044, #3854, #30666, #86092, #45597, #59249, #37484, #3411, #72012, #23864, #44724, #51535, #11102, #31100, #66514, #17920, #79284, #60131, #39261, #79728, #86980, #58796, #86540, #24305, #24741, #17485, #45165, #80172 ),
 .UNSPECIFIED., .F., .F.,
 ( 4, 2, 2, 2, 1, 1, 2, 2, 2, 2, 1, 1, 1, 2, 2, 2, 4 ),
 ( 0.000000000000000000, 0.2500000000002159939, 0.3750000000003109735, 0.4375000000003584355, 0.4687500000003821943, 0.4843750000003940182, 0.4921875000003999023, 0.5000000000004057865, 0.6250000000005055956, 0.6875000000005423439, 0.7187500000005555556, 0.7343750000005554446, 0.7421875000005508927, 0.7460937500005536682, 0.7500000000005564438, 0.8750000000002782219, 1.000000000000000000 ),
 .UNSPECIFIED. ) ;
#86409=EDGE_CURVE ( 'NONE', #2107, #17136, #2168, .T. ) ;
#86418=CARTESIAN_POINT ( 'NONE',  ( 107.0667039024470313, -104.2784471599413791, 2.217806855418003043 ) ) ;
#86425=EDGE_CURVE ( 'NONE', #8767, #8874, #16248, .T. ) ;
#86455=CARTESIAN_POINT ( 'NONE',  ( 117.4590087478601248, -92.77844715994211811, -21.78219314458237932 ) ) ;
#86489=ORIENTED_EDGE ( 'NONE', *, *, #7140, .F. ) ;
#86500=CARTESIAN_POINT ( 'NONE',  ( 107.0667039024470313, -104.2784471599413934, 2.217806855418003043 ) ) ;
#86507=EDGE_CURVE ( 'NONE', #71967, #87130, #48935, .T. ) ;
#86526=VECTOR ( 'NONE', #23914, 1000.000000000000000 ) ;
#86532=FACE_OUTER_BOUND ( 'NONE', #39007, .T. ) ;
#86540=CARTESIAN_POINT ( 'NONE',  ( 68.11045611443701375, -137.1406750370357770, 247.2637542258202927 ) ) ;
#86542=CARTESIAN_POINT ( 'NONE',  ( 69.60882292926817172, -140.2205661867621700, 245.5201220391730033 ) ) ;
#86554=CARTESIAN_POINT ( 'NONE',  ( 110.2536356736639220, -106.6957733451327215, -19.78219314458193168 ) ) ;
#86558=VERTEX_POINT ( 'NONE', #24399 ) ;
#86584=VECTOR ( 'NONE', #70281, 1000.000000000000000 ) ;
#86585=CARTESIAN_POINT ( 'NONE',  ( 85.58879520791417406, -87.02121134100643474, 250.2178068554179333 ) ) ;
#86588=VECTOR ( 'NONE', #39698, 1000.000000000000000 ) ;
#86615=EDGE_CURVE ( 'NONE', #1864, #86337, #58952, .T. ) ;
#86637=DIRECTION ( 'NONE',  ( 1.000000000000000000, 1.132880637372608296E-15, 0.000000000000000000 ) ) ;
#86654=ORIENTED_EDGE ( 'NONE', *, *, #27290, .F. ) ;
#86660=ORIENTED_EDGE ( 'NONE', *, *, #79850, .F. ) ;
#86663=CARTESIAN_POINT ( 'NONE',  ( 52.06670390244699576, -68.87844715994100397, 222.2178068554179902 ) ) ;
#86686=ORIENTED_EDGE ( 'NONE', *, *, #1605, .F. ) ;
#86692=LINE ( 'NONE', #44434, #22942 ) ;
#86697=ORIENTED_EDGE ( 'NONE', *, *, #50674, .F. ) ;
#86706=CARTESIAN_POINT ( 'NONE',  ( 67.06332395966860815, -67.87844715994098976, 246.0535151165250056 ) ) ;
#86717=EDGE_CURVE ( 'NONE', #82398, #48031, #13448, .T. ) ;
#86737=DIRECTION ( 'NONE',  ( -0.9999999999998281375, 0.000000000000000000, 5.861124988064729938E-07 ) ) ;
#86746=EDGE_CURVE ( 'NONE', #37134, #4381, #72208, .T. ) ;
#86771=FACE_OUTER_BOUND ( 'NONE', #55361, .T. ) ;
#86776=AXIS2_PLACEMENT_3D ( 'NONE', #89685, #624, #7000 ) ;
#86777=VERTEX_POINT ( 'NONE', #26621 ) ;
#86794=VERTEX_POINT ( 'NONE', #6629 ) ;
#86816=VECTOR ( 'NONE', #16624, 1000.000000000000000 ) ;
#86825=LINE ( 'NONE', #51825, #61661 ) ;
#86826=DIRECTION ( 'NONE',  ( 1.000000000000000000, 1.000000000000000078E-15, 0.000000000000000000 ) ) ;
#86835=CIRCLE ( 'NONE', #14352, 3.499999999999996003 ) ;
#86837=CARTESIAN_POINT ( 'NONE',  ( 137.0667039024470171, -90.27844715994091018, 230.7030882296565721 ) ) ;
#86838=( BOUNDED_CURVE ( )  B_SPLINE_CURVE ( 3, ( #68629, #34546, #89074, #67727 ),
 .UNSPECIFIED., .F., .T. ) 
 B_SPLINE_CURVE_WITH_KNOTS ( ( 4, 4 ),
 ( 2.671434693666587812, 3.611750613512999308 ),
 .UNSPECIFIED. ) 
 CURVE ( )  GEOMETRIC_REPRESENTATION_ITEM ( )  RATIONAL_B_SPLINE_CURVE ( ( 1.000000000000000000, 0.9276644927932375939, 0.9276644927932375939, 1.000000000000000000 ) ) 
 REPRESENTATION_ITEM ( '' )  );
#86849=EDGE_CURVE ( 'NONE', #81381, #753, #25726, .T. ) ;
#86852=EDGE_CURVE ( 'NONE', #86777, #33131, #39356, .T. ) ;
#86854=DIRECTION ( 'NONE',  ( -1.000000000000000000, -3.114895971316861016E-16, 0.000000000000000000 ) ) ;
#86859=LINE ( 'NONE', #39140, #54572 ) ;
#86865=PLANE ( 'NONE',  #24521 ) ;
#86871=DIRECTION ( 'NONE',  ( -1.000000000000000078E-15, 1.000000000000000000, 0.000000000000000000 ) ) ;
#86887=DIRECTION ( 'NONE',  ( 0.000000000000000000, 0.000000000000000000, -1.000000000000000000 ) ) ;
#86894=PLANE ( 'NONE',  #8563 ) ;
#86902=LINE ( 'NONE', #52772, #47195 ) ;
#86921=CARTESIAN_POINT ( 'NONE',  ( 145.8651347429109251, -69.02927824504203613, 247.3313947546042755 ) ) ;
#86963=CIRCLE ( 'NONE', #50709, 3.999999999999998224 ) ;
#86971=CARTESIAN_POINT ( 'NONE',  ( 106.0667039024470171, -87.35579742913141388, -11.78219314458253741 ) ) ;
#86974=CARTESIAN_POINT ( 'NONE',  ( 74.06670390244701707, -90.27844715994098124, 45.21780685541799727 ) ) ;
#86980=CARTESIAN_POINT ( 'NONE',  ( 68.09855418781428682, -137.1459507998173137, 247.2571523348723019 ) ) ;
#86981=CARTESIAN_POINT ( 'NONE',  ( 56.06670390244699576, -67.87844715994098976, 85.21780685541799016 ) ) ;
#86992=FACE_OUTER_BOUND ( 'NONE', #14491, .T. ) ;
#87012=LINE ( 'NONE', #3443, #60170 ) ;
#87018=ADVANCED_FACE ( 'NONE', ( #18694 ), #72772, .F. ) ;
#87028=ADVANCED_FACE ( 'NONE', ( #39137 ), #25508, .T. ) ;
#87029=FACE_OUTER_BOUND ( 'NONE', #75976, .T. ) ;
#87035=EDGE_CURVE ( 'NONE', #21921, #24432, #24356, .T. ) ;
#87039=VECTOR ( 'NONE', #76427, 1000.000000000000000 ) ;
#87042=VERTEX_POINT ( 'NONE', #59562 ) ;
#87052=ORIENTED_EDGE ( 'NONE', *, *, #77859, .F. ) ;
#87069=ADVANCED_FACE ( 'NONE', ( #66842 ), #88205, .T. ) ;
#87073=VERTEX_POINT ( 'NONE', #5067 ) ;
#87087=DIRECTION ( 'NONE',  ( -1.000000000000000000, -1.000000000000000078E-15, 0.000000000000000000 ) ) ;
#87098=CARTESIAN_POINT ( 'NONE',  ( 117.0667039024470455, -109.9573555057414325, 7.717806855418146483 ) ) ;
#87109=DIRECTION ( 'NONE',  ( -1.000000000000000000, -8.540177112501204385E-16, 0.000000000000000000 ) ) ;
#87112=FACE_OUTER_BOUND ( 'NONE', #33848, .T. ) ;
#87115=ORIENTED_EDGE ( 'NONE', *, *, #46886, .F. ) ;
#87117=ORIENTED_EDGE ( 'NONE', *, *, #59201, .T. ) ;
#87125=CARTESIAN_POINT ( 'NONE',  ( 122.2211106478290219, -96.60847398039683753, -19.21044887263825984 ) ) ;
#87130=VERTEX_POINT ( 'NONE', #54974 ) ;
#87138=CARTESIAN_POINT ( 'NONE',  ( 117.4590087478601390, -115.7784471599421181, -21.78219314458165812 ) ) ;
#87139=EDGE_CURVE ( 'NONE', #38611, #81699, #50463, .T. ) ;
#87148=AXIS2_PLACEMENT_3D ( 'NONE', #67448, #60627, #68805 ) ;
#87150=CIRCLE ( 'NONE', #7390, 1.999999999999995781 ) ;
#87202=CARTESIAN_POINT ( 'NONE',  ( 110.7536356736639078, -102.7271463785351528, 2.217806855417947531 ) ) ;
#87204=AXIS2_PLACEMENT_3D ( 'NONE', #45929, #66390, #24622 ) ;
#87210=PRODUCT_CONTEXT ( 'NONE', #21423, 'mechanical' ) ;
#87215=DIRECTION ( 'NONE',  ( -3.100000000000000258E-29, 3.100000000000000044E-14, 1.000000000000000000 ) ) ;
#87218=CIRCLE ( 'NONE', #59627, 8.999999999999994671 ) ;
#87228=CARTESIAN_POINT ( 'NONE',  ( 107.9678037105606307, -121.2545485715093463, -19.18411693322849487 ) ) ;
#87231=ADVANCED_FACE ( 'NONE', ( #55874 ), #83625, .F. ) ;
#87235=AXIS2_PLACEMENT_3D ( 'NONE', #56571, #28421, #21630 ) ;
#87250=DIRECTION ( 'NONE',  ( -0.000000000000000000, -0.000000000000000000, -1.000000000000000000 ) ) ;
#87251=FACE_OUTER_BOUND ( 'NONE', #83828, .T. ) ;
#87258=FACE_OUTER_BOUND ( 'NONE', #87511, .T. ) ;
#87269=ORIENTED_EDGE ( 'NONE', *, *, #4254, .F. ) ;
#87293=EDGE_LOOP ( 'NONE', ( #44063, #23951, #32945, #64209, #35266, #44473 ) ) ;
#87304=EDGE_CURVE ( 'NONE', #27286, #63455, #43257, .T. ) ;
#87314=LINE ( 'NONE', #80063, #38773 ) ;
#87315=PLANE ( 'NONE',  #83564 ) ;
#87320=B_SPLINE_CURVE_WITH_KNOTS ( 'NONE', 3,
 ( #2016, #43330, #8844, #36543, #83346, #76522, #29719, #21118, #48791, #69717, #86921, #72836, #24244, #24684, #31936, #2467, #10165, #44667, #17865, #65575, #44212, #45993, #30610, #17429, #30162, #38749, #59629, #2910, #23808, #9721, #18309, #79225, #73725, #52351, #87365, #80553 ),
 .UNSPECIFIED., .F., .F.,
 ( 4, 2, 2, 2, 2, 1, 2, 2, 2, 2, 2, 2, 2, 2, 2, 1, 2, 2, 4 ),
 ( 0.000000000000000000, 0.06249999999997138400, 0.09374999999994827748, 0.1249999999999251710, 0.1874999999998892275, 0.2187499999998792077, 0.2343749999998742950, 0.2499999999998693823, 0.3749999999999009681, 0.4374999999999187872, 0.4687499999999116262, 0.4999999999999044098, 0.6249999999999289457, 0.6874999999999485967, 0.7499999999999681366, 0.8124999999999876765, 0.8437499999999974465, 0.8750000000000072164, 1.000000000000000000 ),
 .UNSPECIFIED. ) ;
#87349=DIRECTION ( 'NONE',  ( -3.100000000000000258E-29, 3.100000000000000044E-14, 1.000000000000000000 ) ) ;
#87353=LINE ( 'NONE', #25559, #37988 ) ;
#87364=CARTESIAN_POINT ( 'NONE',  ( 68.85834700699179223, -69.56425716864252706, 247.5000682988239760 ) ) ;
#87365=CARTESIAN_POINT ( 'NONE',  ( 147.0652011257825222, -67.87844715994089029, 245.6323489049700868 ) ) ;
#87370=( BOUNDED_CURVE ( )  B_SPLINE_CURVE ( 3, ( #13899, #67508, #19372, #67965 ),
 .UNSPECIFIED., .F., .T. ) 
 B_SPLINE_CURVE_WITH_KNOTS ( ( 4, 4 ),
 ( 3.141592653589793116, 3.611750613512999308 ),
 .UNSPECIFIED. ) 
 CURVE ( )  GEOMETRIC_REPRESENTATION_ITEM ( )  RATIONAL_B_SPLINE_CURVE ( ( 1.000000000000000000, 0.9816639655796099984, 0.9816639655796099984, 1.000000000000000000 ) ) 
 REPRESENTATION_ITEM ( '' )  );
#87374=ORIENTED_EDGE ( 'NONE', *, *, #33713, .F. ) ;
#87375=ORIENTED_EDGE ( 'NONE', *, *, #86746, .F. ) ;
#87398=CARTESIAN_POINT ( 'NONE',  ( 107.0667039024470313, -104.2784471599420755, -19.78219314458201694 ) ) ;
#87399=EDGE_LOOP ( 'NONE', ( #89163, #50886, #55431, #13828, #85339, #24394, #32837, #84334, #88545, #43883 ) ) ;
#87410=CARTESIAN_POINT ( 'NONE',  ( 143.5890317271348238, -139.7841266254118011, 247.2002237598829311 ) ) ;
#87445=PLANE ( 'NONE',  #77972 ) ;
#87450=CARTESIAN_POINT ( 'NONE',  ( 144.0667039024470739, -137.6784471599409017, 55.21780685541800437 ) ) ;
#87457=AXIS2_PLACEMENT_3D ( 'NONE', #10071, #57303, #30952 ) ;
#87472=DIRECTION ( 'NONE',  ( 1.000000000000000000, 1.132880637372608296E-15, 0.000000000000000000 ) ) ;
#87474=EDGE_CURVE ( 'NONE', #58142, #85724, #4523, .T. ) ;
#87477=VECTOR ( 'NONE', #8096, 1000.000000000000000 ) ;
#87490=CARTESIAN_POINT ( 'NONE',  ( 70.56670390244700286, -67.87844715994098976, 222.2178068554179902 ) ) ;
#87491=VERTEX_POINT ( 'NONE', #39482 ) ;
#87501=DIRECTION ( 'NONE',  ( 0.8660254037844382635, 0.5000000000000008882, -1.550000000000000022E-14 ) ) ;
#87502=DIRECTION ( 'NONE',  ( -3.100000000000000258E-29, 3.100000000000000044E-14, 1.000000000000000000 ) ) ;
#87511=EDGE_LOOP ( 'NONE', ( #10686, #12586, #53780, #4696, #23611, #2402, #71918, #85778 ) ) ;
#87514=ORIENTED_EDGE ( 'NONE', *, *, #13813, .F. ) ;
#87544=EDGE_CURVE ( 'NONE', #35902, #59214, #86306, .T. ) ;
#87579=CIRCLE ( 'NONE', #84684, 2.000000000000001776 ) ;
#87593=CARTESIAN_POINT ( 'NONE',  ( 106.0667039024470171, -87.35579742913172652, -21.78219314458254630 ) ) ;
#87594=DIRECTION ( 'NONE',  ( 1.000000000000000000, 1.132880637372608296E-15, 0.000000000000000000 ) ) ;
#87600=ORIENTED_EDGE ( 'NONE', *, *, #77859, .T. ) ;
#87656=ADVANCED_FACE ( 'NONE', ( #76243, #74904 ), #14924, .T. ) ;
#87661=CARTESIAN_POINT ( 'NONE',  ( 103.8797721312301405, -101.8611209747514010, -19.78219314458209865 ) ) ;
#87727=CARTESIAN_POINT ( 'NONE',  ( 107.9678037105606023, -87.30234574837481887, -21.78219314458254630 ) ) ;
#87732=CARTESIAN_POINT ( 'NONE',  ( 78.89953865151133527, -101.2959575815152675, 250.2190963482990185 ) ) ;
#87739=EDGE_CURVE ( 'NONE', #84388, #17172, #62137, .T. ) ;
#87754=CARTESIAN_POINT ( 'NONE',  ( 91.91125933621934507, -111.8737466215628160, -19.26696060647578435 ) ) ;
#87761=CARTESIAN_POINT ( 'NONE',  ( 147.0667039024470171, -77.84948640091441519, 245.5415602474340062 ) ) ;
#87780=DIRECTION ( 'NONE',  ( -1.000000000000000000, -1.206764157201257538E-15, 0.000000000000000000 ) ) ;
#87795=EDGE_CURVE ( 'NONE', #75315, #37650, #36086, .T. ) ;
#87797=CARTESIAN_POINT ( 'NONE',  ( 106.1656040943334318, -87.30234574837474781, -19.18411693322955003 ) ) ;
#87807=CARTESIAN_POINT ( 'NONE',  ( 121.3178890780284291, -95.01002112898673602, -19.18411693322930134 ) ) ;
#87814=DIRECTION ( 'NONE',  ( 1.000000000000000000, 1.000000000000000078E-15, 0.000000000000000000 ) ) ;
#87828=EDGE_CURVE ( 'NONE', #66416, #85229, #4179, .T. ) ;
#87829=LINE ( 'NONE', #81034, #44879 ) ;
#87846=DIRECTION ( 'NONE',  ( 1.000000000000000000, 0.000000000000000000, 0.000000000000000000 ) ) ;
#87859=CARTESIAN_POINT ( 'NONE',  ( 143.5320129146941213, -139.6569233413941618, 247.2784140332015568 ) ) ;
#87895=CARTESIAN_POINT ( 'NONE',  ( 92.91125933621934507, -113.6057974291317691, -21.78219314458173983 ) ) ;
#87911=CARTESIAN_POINT ( 'NONE',  ( 67.06804154766946624, -67.87911383296281542, 245.5633152175482223 ) ) ;
#87941=ORIENTED_EDGE ( 'NONE', *, *, #70487, .T. ) ;
#87949=CARTESIAN_POINT ( 'NONE',  ( 129.9695788989828600, -140.6784471599409301, 245.6313834131549925 ) ) ;
#87953=CARTESIAN_POINT ( 'NONE',  ( 106.0988423365887030, -87.33724229552865381, -19.23816181211554621 ) ) ;
#87967=AXIS2_PLACEMENT_3D ( 'NONE', #87661, #46745, #88119 ) ;
#87971=CARTESIAN_POINT ( 'NONE',  ( 115.5439452383992176, -108.5954344580498372, -19.78219314458187839 ) ) ;
#87984=EDGE_LOOP ( 'NONE', ( #27119, #89804, #29910, #32504, #69121, #20846, #44494, #74506 ) ) ;
#87993=PLANE ( 'NONE',  #39388 ) ;
#88002=CARTESIAN_POINT ( 'NONE',  ( 77.10595377993877264, -140.3990126765571631, 246.8970167045860080 ) ) ;
#88008=ORIENTED_EDGE ( 'NONE', *, *, #50859, .T. ) ;
#88032=B_SPLINE_CURVE_WITH_KNOTS ( 'NONE', 3,
 ( #76472, #14254, #42377, #7880 ),
 .UNSPECIFIED., .F., .F.,
 ( 4, 4 ),
 ( -0.3974825557268100162, -0.3842043193313829930 ),
 .UNSPECIFIED. ) ;
#88034=VERTEX_POINT ( 'NONE', #53869 ) ;
#88040=EDGE_LOOP ( 'NONE', ( #43791, #44243, #3832, #4712 ) ) ;
#88047=DIRECTION ( 'NONE',  ( -0.5000000000000008882, 0.8660254037844382635, -2.684678751731760294E-14 ) ) ;
#88048=CARTESIAN_POINT ( 'NONE',  ( 143.2705975587811906, -69.15250645760630732, 247.4440349298869819 ) ) ;
#88106=CIRCLE ( 'NONE', #66288, 3.500000000000003109 ) ;
#88107=CARTESIAN_POINT ( 'NONE',  ( 99.90204555947735798, -107.8376143137176939, -19.78219314458190681 ) ) ;
#88117=DIRECTION ( 'NONE',  ( -1.000000000000000000, -8.953411488912552682E-16, 0.000000000000000000 ) ) ;
#88119=DIRECTION ( 'NONE',  ( -3.100000000000000258E-29, 3.100000000000000044E-14, 1.000000000000000000 ) ) ;
#88126=VERTEX_POINT ( 'NONE', #40710 ) ;
#88142=CIRCLE ( 'NONE', #33016, 15.50000000000000000 ) ;
#88150=ORIENTED_EDGE ( 'NONE', *, *, #26302, .T. ) ;
#88193=VERTEX_POINT ( 'NONE', #83862 ) ;
#88201=DIRECTION ( 'NONE',  ( -1.000000000000000000, -1.000000000000000078E-15, -0.000000000000000000 ) ) ;
#88203=DIRECTION ( 'NONE',  ( -0.9217329428042198014, -0.3878251953515564066, 1.214306433183767175E-14 ) ) ;
#88205=PLANE ( 'NONE',  #25837 ) ;
#88259=CARTESIAN_POINT ( 'NONE',  ( 92.17622411536551397, -83.77844715994095282, 55.21780685541800437 ) ) ;
#88265=PLANE ( 'NONE',  #58866 ) ;
#88270=VECTOR ( 'NONE', #86085, 1000.000000000000000 ) ;
#88296=CARTESIAN_POINT ( 'NONE',  ( 144.0637245237351749, -140.6784087391956746, 245.5331728883010101 ) ) ;
#88302=LINE ( 'NONE', #74651, #60283 ) ;
#88312=EDGE_CURVE ( 'NONE', #49237, #24886, #35550, .T. ) ;
#88338=CARTESIAN_POINT ( 'NONE',  ( 125.5177273812784762, -131.0330679306342176, 55.21780685541800437 ) ) ;
#88348=ORIENTED_EDGE ( 'NONE', *, *, #37085, .F. ) ;
#88353=DIRECTION ( 'NONE',  ( -0.3535533905932733423, -0.6123724356957724879, 0.7071067811865668906 ) ) ;
#88357=LINE ( 'NONE', #88802, #84806 ) ;
#88362=ORIENTED_EDGE ( 'NONE', *, *, #48243, .F. ) ;
#88367=CARTESIAN_POINT ( 'NONE',  ( 107.0667039024470313, -104.2784471599420755, -19.78219314458201694 ) ) ;
#88368=CARTESIAN_POINT ( 'NONE',  ( 107.0667039024470313, -104.2784471599420755, -19.78219314458201694 ) ) ;
#88428=DIRECTION ( 'NONE',  ( -1.000000000000000078E-15, 1.000000000000000000, 0.000000000000000000 ) ) ;
#88429=DIRECTION ( 'NONE',  ( 0.000000000000000000, 0.000000000000000000, 1.000000000000000000 ) ) ;
#88452=VECTOR ( 'NONE', #54132, 1000.000000000000000 ) ;
#88461=CARTESIAN_POINT ( 'NONE',  ( 70.40117688449606703, -140.5784839457434998, 246.8085677970040024 ) ) ;
#88478=EDGE_CURVE ( 'NONE', #22589, #67053, #37828, .T. ) ;
#88487=VECTOR ( 'NONE', #30658, 1000.000000000000000 ) ;
#88490=CARTESIAN_POINT ( 'NONE',  ( 143.0667039024470171, -118.2784471599408960, 222.2178068554179902 ) ) ;
#88502=ADVANCED_FACE ( 'NONE', ( #88773 ), #67866, .T. ) ;
#88504=VECTOR ( 'NONE', #14974, 999.9999999999998863 ) ;
#88506=CARTESIAN_POINT ( 'NONE',  ( 107.0667039024470313, -104.2784471599420755, -19.78219314458201694 ) ) ;
#88510=VERTEX_POINT ( 'NONE', #27419 ) ;
#88513=PLANE ( 'NONE',  #13642 ) ;
#88521=EDGE_LOOP ( 'NONE', ( #33297, #4874, #34972, #31450, #72713 ) ) ;
#88545=ORIENTED_EDGE ( 'NONE', *, *, #5809, .F. ) ;
#88553=ORIENTED_EDGE ( 'NONE', *, *, #48916, .F. ) ;
#88554=ADVANCED_FACE ( 'NONE', ( #25632 ), #40145, .F. ) ;
#88601=ORIENTED_EDGE ( 'NONE', *, *, #56646, .F. ) ;
#88602=EDGE_CURVE ( 'NONE', #5461, #17136, #22417, .T. ) ;
#88618=ORIENTED_EDGE ( 'NONE', *, *, #40334, .F. ) ;
#88621=CIRCLE ( 'NONE', #4509, 23.50000000000000711 ) ;
#88626=CIRCLE ( 'NONE', #56892, 3.000000864267354572 ) ;
#88643=PLANE ( 'NONE',  #17071 ) ;
#88647=EDGE_LOOP ( 'NONE', ( #58702, #85606, #83620, #35446 ) ) ;
#88648=CYLINDRICAL_SURFACE ( 'NONE', #86184, 3.999999999999992895 ) ;
#88653=CARTESIAN_POINT ( 'NONE',  ( 98.58946256649487339, -99.96145986183429955, -19.78219314458215550 ) ) ;
#88671=CARTESIAN_POINT ( 'NONE',  ( 147.0667039024470739, -137.6758869494786097, 245.5072624240089851 ) ) ;
#88705=DIRECTION ( 'NONE',  ( 0.7349399772593259161, -0.6687953793059864260, 0.1121426343770440259 ) ) ;
#88739=EDGE_CURVE ( 'NONE', #71630, #11403, #88032, .T. ) ;
#88767=EDGE_CURVE ( 'NONE', #70410, #23818, #77369, .T. ) ;
#88769=CARTESIAN_POINT ( 'NONE',  ( 92.81551872686563343, -113.5468731908973723, -19.18411693322874356 ) ) ;
#88773=FACE_OUTER_BOUND ( 'NONE', #38829, .T. ) ;
#88802=CARTESIAN_POINT ( 'NONE',  ( 143.7922156418627821, -137.6784471599409017, 222.2178068554179902 ) ) ;
#88826=ADVANCED_FACE ( 'NONE', ( #23761, #85989, #57814, #17820, #9229, #59138, #79620, #78735, #78287, #37829 ), #3747, .T. ) ;
#88863=CARTESIAN_POINT ( 'NONE',  ( 74.06670390244704549, -118.2784471599409812, 45.21780685541799727 ) ) ;
#88893=CARTESIAN_POINT ( 'NONE',  ( 68.06670390244705970, -121.7784471599409954, 45.21780685541799727 ) ) ;
#88900=VERTEX_POINT ( 'NONE', #14556 ) ;
#88905=CARTESIAN_POINT ( 'NONE',  ( 129.9869660233263744, -139.6169024007319024, 247.4725286609620127 ) ) ;
#88921=DIRECTION ( 'NONE',  ( 0.7967329428042202455, -0.6043315462976655006, 1.908195823574484964E-14 ) ) ;
#88929=DIRECTION ( 'NONE',  ( -3.100000000000000258E-29, 3.100000000000000044E-14, 1.000000000000000000 ) ) ;
#88936=ORIENTED_EDGE ( 'NONE', *, *, #50337, .T. ) ;
#88939=PLANE ( 'NONE',  #14192 ) ;
#88940=CARTESIAN_POINT ( 'NONE',  ( 99.06670390244704549, -104.2784471599421323, -21.78219314458201694 ) ) ;
#88964=CARTESIAN_POINT ( 'NONE',  ( 138.0667039024470171, -104.2784471599409244, 25.71780685541800437 ) ) ;
#88977=CARTESIAN_POINT ( 'NONE',  ( 103.3797721312301547, -105.8297479413476196, 2.217806855418058554 ) ) ;
#88993=CIRCLE ( 'NONE', #35284, 3.000000000000002665 ) ;
#89022=ORIENTED_EDGE ( 'NONE', *, *, #27551, .T. ) ;
#89074=CARTESIAN_POINT ( 'NONE',  ( 113.5015236877821962, -87.59835267194286246, -9.274842254011153031 ) ) ;
#89093=CARTESIAN_POINT ( 'NONE',  ( 138.0264040502034391, -139.2425132489394457, 247.5112265945669776 ) ) ;
#89119=AXIS2_PLACEMENT_3D ( 'NONE', #26542, #12926, #81535 ) ;
#89134=FACE_OUTER_BOUND ( 'NONE', #29025, .T. ) ;
#89163=ORIENTED_EDGE ( 'NONE', *, *, #59519, .F. ) ;
#89164=EDGE_CURVE ( 'NONE', #67043, #27883, #26597, .T. ) ;
#89170=EDGE_CURVE ( 'NONE', #74974, #25248, #68111, .T. ) ;
#89215=B_SPLINE_CURVE_WITH_KNOTS ( 'NONE', 3,
 ( #14632, #29151, #56388, #48220, #35959, #69591 ),
 .UNSPECIFIED., .F., .F.,
 ( 4, 2, 4 ),
 ( -0.008552427134052589808, -0.004278148697845064567, -7.255242802014019721E-06 ),
 .UNSPECIFIED. ) ;
#89257=CARTESIAN_POINT ( 'NONE',  ( 98.58946256649485917, -108.5954344580491693, 2.217806855418142042 ) ) ;
#89259=PLANE ( 'NONE',  #3917 ) ;
#89310=CARTESIAN_POINT ( 'NONE',  ( 110.0667047667142953, -67.87844715994094713, 173.2178068554179902 ) ) ;
#89313=CIRCLE ( 'NONE', #50124, 3.500000000000003109 ) ;
#89318=CARTESIAN_POINT ( 'NONE',  ( 91.91125933621933086, -100.4807974291314423, -11.78219314458211997 ) ) ;
#89342=CARTESIAN_POINT ( 'NONE',  ( 70.06670390244707392, -137.6784471599409869, 222.2178068554179902 ) ) ;
#89353=CARTESIAN_POINT ( 'NONE',  ( 77.11349091887886686, -140.6783563551099689, 245.9764622033119963 ) ) ;
#89354=CARTESIAN_POINT ( 'NONE',  ( 145.1838268511080798, -139.0510231921375350, 246.8128416193126782 ) ) ;
#89357=ORIENTED_EDGE ( 'NONE', *, *, #52113, .F. ) ;
#89361=CARTESIAN_POINT ( 'NONE',  ( 67.06670390244701707, -79.67844715994098692, 55.21780685541800437 ) ) ;
#89362=VECTOR ( 'NONE', #25246, 1000.000000000000000 ) ;
#89374=LINE ( 'NONE', #59845, #256 ) ;
#89376=CIRCLE ( 'NONE', #13958, 23.50000000000000711 ) ;
#89377=VECTOR ( 'NONE', #36844, 1000.000000000000000 ) ;
#89379=CARTESIAN_POINT ( 'NONE',  ( 107.0667039024470313, -104.2784471599420755, -19.78219314458201694 ) ) ;
#89389=LINE ( 'NONE', #28036, #3975 ) ;
#89402=EDGE_LOOP ( 'NONE', ( #23738, #89357, #57690, #68393 ) ) ;
#89415=AXIS2_PLACEMENT_3D ( 'NONE', #29957, #64914, #24037 ) ;
#89420=CARTESIAN_POINT ( 'NONE',  ( 59.56670390244699576, -67.87844715994098976, 85.21780685541799016 ) ) ;
#89438=AXIS2_PLACEMENT_3D ( 'NONE', #61114, #26156, #18890 ) ;
#89450=VERTEX_POINT ( 'NONE', #64960 ) ;
#89462=EDGE_CURVE ( 'NONE', #40899, #35252, #82721, .T. ) ;
#89464=DIRECTION ( 'NONE',  ( 0.000000000000000000, 0.000000000000000000, 1.000000000000000000 ) ) ;
#89487=ORIENTED_EDGE ( 'NONE', *, *, #82003, .T. ) ;
#89504=ORIENTED_EDGE ( 'NONE', *, *, #61301, .F. ) ;
#89531=ORIENTED_EDGE ( 'NONE', *, *, #29932, .F. ) ;
#89554=PLANE ( 'NONE',  #56817 ) ;
#89562=VECTOR ( 'NONE', #52491, 1000.000000000000000 ) ;
#89569=CARTESIAN_POINT ( 'NONE',  ( 141.9478362311689068, -91.32555531421861872, 248.3919668373590071 ) ) ;
#89590=VECTOR ( 'NONE', #48654, 1000.000000000000000 ) ;
#89615=VERTEX_POINT ( 'NONE', #4520 ) ;
#89624=CARTESIAN_POINT ( 'NONE',  ( 154.5667039024469886, -67.87844715994090450, 190.2178068554179902 ) ) ;
#89656=CARTESIAN_POINT ( 'NONE',  ( 0.000000000000000000, 0.000000000000000000, 0.000000000000000000 ) ) ;
#89681=DIRECTION ( 'NONE',  ( 1.000000000000000078E-15, -1.000000000000000000, 0.000000000000000000 ) ) ;
#89685=CARTESIAN_POINT ( 'NONE',  ( 107.0667039024470313, -104.2784471599420755, -19.78219314458201694 ) ) ;
#89691=DIRECTION ( 'NONE',  ( 0.000000000000000000, 0.000000000000000000, -1.000000000000000000 ) ) ;
#89708=DIRECTION ( 'NONE',  ( -3.100000000000000258E-29, 3.100000000000000044E-14, 1.000000000000000000 ) ) ;
#89712=CARTESIAN_POINT ( 'NONE',  ( 98.58946256649485917, -108.5954344580498514, -19.78219314458187839 ) ) ;
#89715=CARTESIAN_POINT ( 'NONE',  ( 67.55352479590314374, -68.34655798362497592, 246.8010709169019776 ) ) ;
#89717=ORIENTED_EDGE ( 'NONE', *, *, #50711, .F. ) ;
#89721=VECTOR ( 'NONE', #11141, 1000.000000000000000 ) ;
#89726=DIRECTION ( 'NONE',  ( 1.000000000000000078E-15, -1.000000000000000000, 0.000000000000000000 ) ) ;
#89728=DIRECTION ( 'NONE',  ( -1.000000000000000000, -1.000000000000000078E-15, 0.000000000000000000 ) ) ;
#89733=DIRECTION ( 'NONE',  ( -0.7071067811865453523, -0.7071067811865496822, 0.000000000000000000 ) ) ;
#89760=ORIENTED_EDGE ( 'NONE', *, *, #52378, .F. ) ;
#89767=DIRECTION ( 'NONE',  ( 1.000000000000000000, 1.000000000000000078E-15, 0.000000000000000000 ) ) ;
#89773=DIRECTION ( 'NONE',  ( 0.000000000000000000, 0.000000000000000000, 1.000000000000000000 ) ) ;
#89776=CARTESIAN_POINT ( 'NONE',  ( 63.06670390244700997, -79.67844715994098692, 155.2178068554179902 ) ) ;
#89792=EDGE_CURVE ( 'NONE', #29468, #61133, #22635, .T. ) ;
#89799=ORIENTED_EDGE ( 'NONE', *, *, #38865, .F. ) ;
#89804=ORIENTED_EDGE ( 'NONE', *, *, #14113, .F. ) ;
#89820=CARTESIAN_POINT ( 'NONE',  ( 110.0667047667142953, -67.87844715994094713, 93.21780685541800437 ) ) ;
#89823=DIRECTION ( 'NONE',  ( 3.100000000000000258E-29, -3.100000000000000044E-14, -1.000000000000000000 ) ) ;
#89842=ORIENTED_EDGE ( 'NONE', *, *, #30302, .F. ) ;
#89852=ORIENTED_EDGE ( 'NONE', *, *, #622, .F. ) ;
#89856=VECTOR ( 'NONE', #26066, 1000.000000000000000 ) ;
#89868=EDGE_CURVE ( 'NONE', #43983, #72685, #17473, .T. ) ;
#89885=CARTESIAN_POINT ( 'NONE',  ( 71.06670390244701707, -83.77844715994098124, 55.21780685541800437 ) ) ;
#89886=ORIENTED_EDGE ( 'NONE', *, *, #72216, .T. ) ;
#89890=ORIENTED_EDGE ( 'NONE', *, *, #87544, .F. ) ;
#89901=DIRECTION ( 'NONE',  ( 3.100000000000000258E-29, -3.100000000000000044E-14, -1.000000000000000000 ) ) ;
#89908=EDGE_CURVE ( 'NONE', #76564, #57999, #43584, .T. ) ;
#89919=DIRECTION ( 'NONE',  ( -0.7071067811865477948, 0.7071067811865473507, 0.000000000000000000 ) ) ;
#89923=CARTESIAN_POINT ( 'NONE',  ( 103.8797721312301547, -106.6957733451320394, 2.217806855418086087 ) ) ;
ENDSEC;
END-ISO-10303-21;
